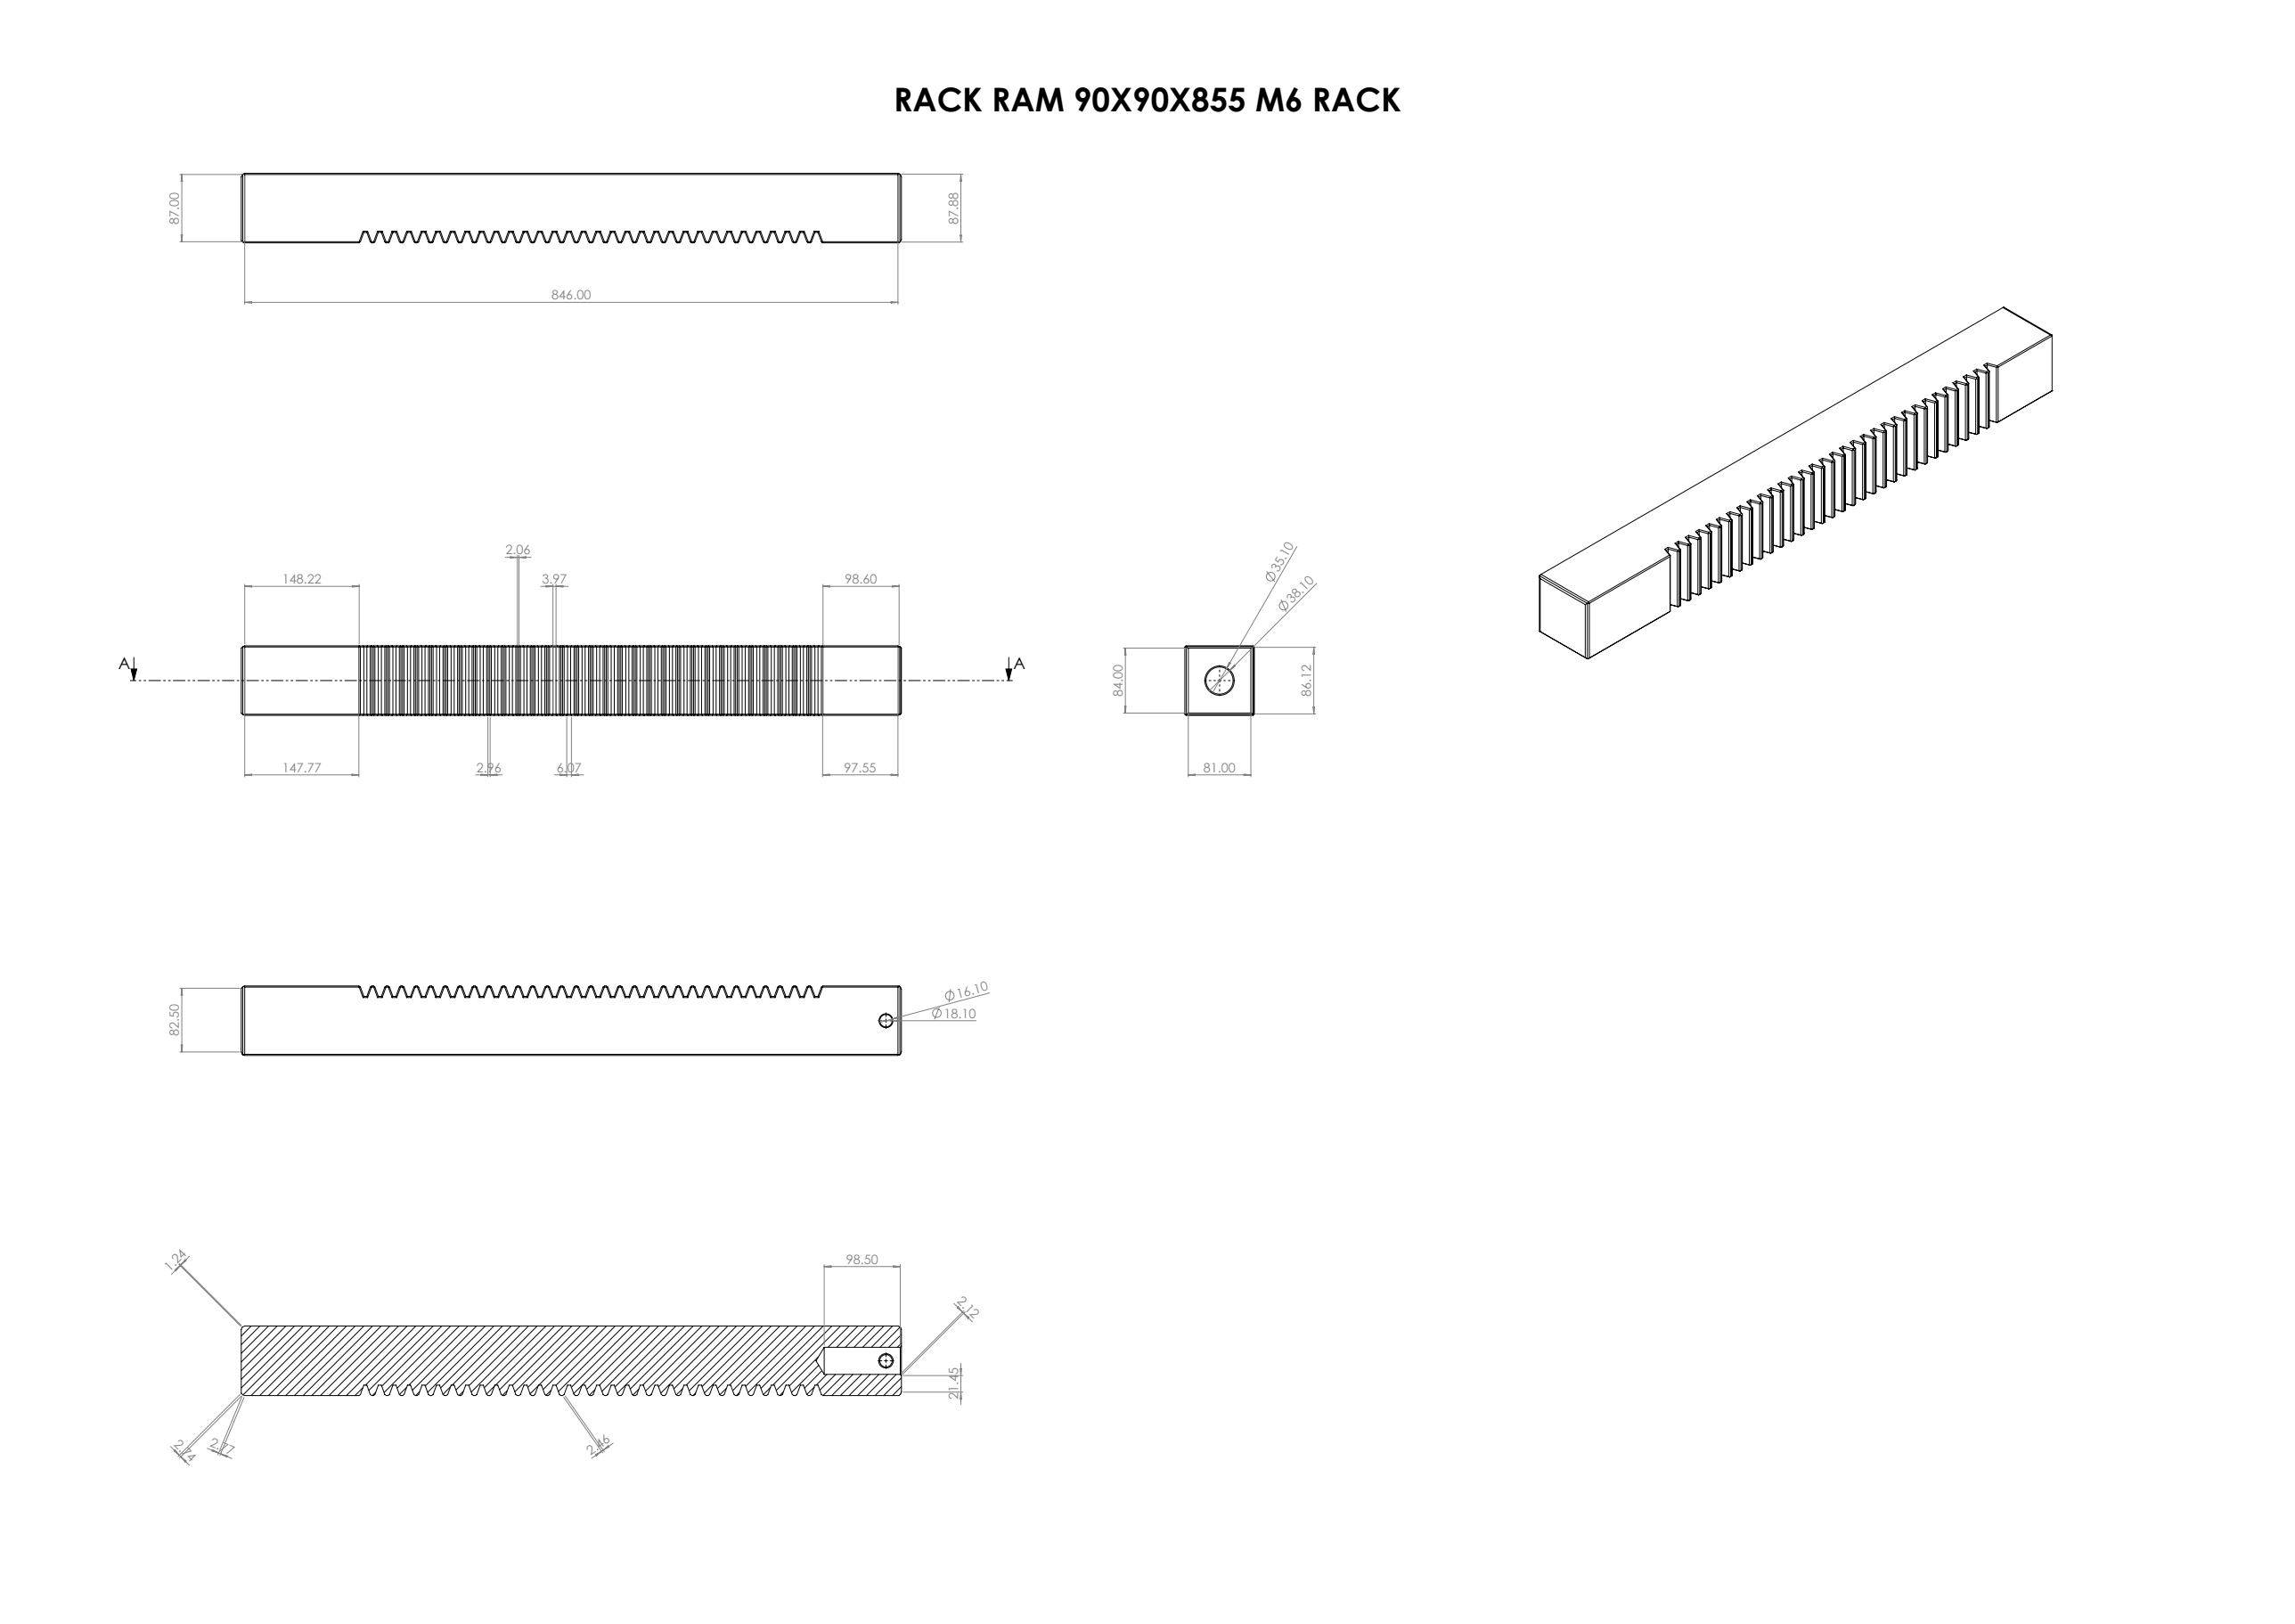
ISO-10303-21;
HEADER;
/* Generated by software containing ST-Developer
 * from STEP Tools, Inc. (www.steptools.com) 
 */

FILE_DESCRIPTION(
/* description */ (''),
/* implementation_level */ '2;1');

FILE_NAME(
/* name */ '02_Rack_Ram_90x90x855_m6_Rack.step',
/* time_stamp */ '2026-10-19T23:58:09-07:00',
/* author */ (''),
/* organization */ (''),
/* preprocessor_version */ 'ST-DEVELOPER v20.2',
/* originating_system */ 'Autodesk Translation Framework v15.15.0.0',
/* authorisation */ '');

FILE_SCHEMA (('AP203_CONFIGURATION_CONTROLLED_3D_DESIGN_OF_MECHANICAL_PARTS_AND_ASSEMBLIES_MIM_LF { 1 0 10303 203 3 1 4 }',
'AUTOMOTIVE_DESIGN { 1 0 10303 214 3 1 1 }','INTEGRATED_CNC_SCHEMA','MODEL_BASED_INTEGRATED_MANUFACTURING_SCHEMA',
'PROCESS_PLANNING_SCHEMA','AP242_MANAGED_MODEL_BASED_3D_ENGINEERING_MIM_LF { 1 0 10303 442 3 1 4 }'));
ENDSEC;

DATA;
#10=MECHANICAL_DESIGN_GEOMETRIC_PRESENTATION_REPRESENTATION('',(#418),#70757);
#286=B_SPLINE_SURFACE_WITH_KNOTS('',3,3,((#63397,#63398,#63399,#63400,#63401,
#63402,#63403,#63404,#63405,#63406,#63407,#63408,#63409,#63410,#63411,#63412,
#63413,#63414,#63415,#63416,#63417,#63418,#63419,#63420,#63421,#63422,#63423,
#63424,#63425,#63426,#63427,#63428,#63429,#63430,#63431,#63432,#63433,#63434,
#63435,#63436),(#63437,#63438,#63439,#63440,#63441,#63442,#63443,#63444,
#63445,#63446,#63447,#63448,#63449,#63450,#63451,#63452,#63453,#63454,#63455,
#63456,#63457,#63458,#63459,#63460,#63461,#63462,#63463,#63464,#63465,#63466,
#63467,#63468,#63469,#63470,#63471,#63472,#63473,#63474,#63475,#63476),
(#63477,#63478,#63479,#63480,#63481,#63482,#63483,#63484,#63485,#63486,
#63487,#63488,#63489,#63490,#63491,#63492,#63493,#63494,#63495,#63496,#63497,
#63498,#63499,#63500,#63501,#63502,#63503,#63504,#63505,#63506,#63507,#63508,
#63509,#63510,#63511,#63512,#63513,#63514,#63515,#63516),(#63517,#63518,
#63519,#63520,#63521,#63522,#63523,#63524,#63525,#63526,#63527,#63528,#63529,
#63530,#63531,#63532,#63533,#63534,#63535,#63536,#63537,#63538,#63539,#63540,
#63541,#63542,#63543,#63544,#63545,#63546,#63547,#63548,#63549,#63550,#63551,
#63552,#63553,#63554,#63555,#63556)),.UNSPECIFIED.,.F.,.T.,.F.,(4,4),(4,
1,1,1,1,1,1,1,1,1,1,1,1,1,1,1,1,1,1,1,1,1,1,1,1,1,1,1,1,1,1,1,1,1,1,1,1,
4),(0.,1.),(0.,0.176188248237271,0.352376496474541,0.528564744711812,0.704752992949082,
0.880941241186353,0.969035365304988,1.01308242736431,1.03510595839396,1.05712948942362,
1.40950598589816,1.42418833991794,1.43887069393771,1.46823540197725,1.52696481805635,
1.64442365021453,1.76188248237271,1.87934131453089,2.11425897884725,2.17298839492634,
2.23171781100543,2.34917664316361,2.58409430747997,2.64282372355906,2.81901197179633,
2.93647080395451,3.05392963611269,3.17138846827087,3.28884730042905,3.52376496474541,
3.64122379690359,3.75868262906177,3.99360029337813,4.22851795769449,4.40470620593176,
4.58089445416904,4.75708270240631,4.93327095064358),.UNSPECIFIED.);
#388=SHAPE_REPRESENTATION_RELATIONSHIP('SRR','None',#70829,#403);
#403=ADVANCED_BREP_SHAPE_REPRESENTATION('',(#478),#70753);
#418=STYLED_ITEM('',(#71033),#478);
#478=MANIFOLD_SOLID_BREP('Ram',#26883);
#728=CYLINDRICAL_SURFACE('',#28278,0.805);
#729=CYLINDRICAL_SURFACE('',#28280,1.755);
#875=FACE_BOUND('',#4734,.T.);
#876=FACE_BOUND('',#4990,.T.);
#877=FACE_BOUND('',#5104,.T.);
#1395=B_SPLINE_CURVE_WITH_KNOTS('',3,(#63561,#63562,#63563,#63564,#63565,
#63566,#63567,#63568,#63569,#63570,#63571,#63572,#63573),.UNSPECIFIED.,
 .F.,.F.,(4,1,1,1,1,1,1,1,1,1,4),(0.,0.176188248237271,0.352376496474541,
0.528564744711812,0.704752992949082,0.880941241186353,0.969035365304988,
1.01308242736431,1.03510595839396,1.05712948942362,1.23331773766089),
 .UNSPECIFIED.);
#1396=B_SPLINE_CURVE_WITH_KNOTS('',3,(#63574,#63575,#63576,#63577,#63578,
#63579,#63580,#63581,#63582,#63583,#63584,#63585,#63586,#63587,#63588,#63589,
#63590,#63591,#63592,#63593,#63594,#63595,#63596,#63597,#63598,#63599,#63600,
#63601,#63602,#63603,#63604),.UNSPECIFIED.,.F.,.F.,(4,1,1,1,1,1,1,1,1,1,
1,1,1,1,1,1,1,1,1,1,1,1,1,1,1,1,1,1,4),(1.23331773766089,1.40950598589816,
1.42418833991794,1.43887069393771,1.46823540197725,1.52696481805635,1.64442365021453,
1.76188248237271,1.87934131453089,2.11425897884725,2.17298839492634,2.23171781100543,
2.34917664316361,2.58409430747997,2.64282372355906,2.81901197179633,2.93647080395451,
3.05392963611269,3.17138846827087,3.28884730042905,3.52376496474541,3.64122379690359,
3.75868262906177,3.99360029337813,4.22851795769449,4.40470620593176,4.58089445416904,
4.75708270240631,4.93327095064358),.UNSPECIFIED.);
#1397=B_SPLINE_CURVE_WITH_KNOTS('',3,(#63605,#63606,#63607,#63608,#63609,
#63610,#63611,#63612,#63613,#63614,#63615,#63616,#63617,#63618,#63619,#63620,
#63621,#63622,#63623,#63624,#63625,#63626,#63627,#63628,#63629,#63630,#63631,
#63632,#63633,#63634,#63635,#63636,#63637,#63638,#63639,#63640,#63641,#63642,
#63643,#63644),.UNSPECIFIED.,.T.,.F.,(4,1,1,1,1,1,1,1,1,1,1,1,1,1,1,1,1,
1,1,1,1,1,1,1,1,1,1,1,1,1,1,1,1,1,1,1,1,4),(-4.93327095064358,-4.75708270240631,
-4.58089445416904,-4.40470620593176,-4.22851795769449,-3.99360029337813,
-3.75868262906177,-3.64122379690359,-3.52376496474541,-3.28884730042905,
-3.17138846827087,-3.05392963611269,-2.93647080395451,-2.81901197179633,
-2.64282372355906,-2.58409430747997,-2.34917664316361,-2.23171781100543,
-2.17298839492634,-2.11425897884725,-1.87934131453089,-1.76188248237271,
-1.64442365021453,-1.52696481805635,-1.46823540197725,-1.43887069393771,
-1.42418833991794,-1.40950598589816,-1.05712948942362,-1.03510595839396,
-1.01308242736431,-0.969035365304988,-0.880941241186353,-0.704752992949082,
-0.528564744711812,-0.352376496474541,-0.176188248237271,0.),
 .UNSPECIFIED.);
#1916=PLANE('',#27819);
#1917=PLANE('',#27820);
#1918=PLANE('',#27821);
#1919=PLANE('',#27822);
#1920=PLANE('',#27823);
#1921=PLANE('',#27824);
#1922=PLANE('',#27825);
#1923=PLANE('',#27826);
#1924=PLANE('',#27827);
#1925=PLANE('',#27828);
#1926=PLANE('',#27829);
#1927=PLANE('',#27830);
#1928=PLANE('',#27831);
#1929=PLANE('',#27832);
#1930=PLANE('',#27833);
#1931=PLANE('',#27834);
#1932=PLANE('',#27835);
#1933=PLANE('',#27836);
#1934=PLANE('',#27837);
#1935=PLANE('',#27838);
#1936=PLANE('',#27839);
#1937=PLANE('',#27840);
#1938=PLANE('',#27841);
#1939=PLANE('',#27842);
#1940=PLANE('',#27843);
#1941=PLANE('',#27844);
#1942=PLANE('',#27845);
#1943=PLANE('',#27846);
#1944=PLANE('',#27847);
#1945=PLANE('',#27848);
#1946=PLANE('',#27849);
#1947=PLANE('',#27850);
#1948=PLANE('',#27851);
#1949=PLANE('',#27852);
#1950=PLANE('',#27853);
#1951=PLANE('',#27854);
#1952=PLANE('',#27855);
#1953=PLANE('',#27856);
#1954=PLANE('',#27857);
#1955=PLANE('',#27858);
#1956=PLANE('',#27859);
#1957=PLANE('',#27860);
#1958=PLANE('',#27861);
#1959=PLANE('',#27862);
#1960=PLANE('',#27863);
#1961=PLANE('',#27864);
#1962=PLANE('',#27865);
#1963=PLANE('',#27866);
#1964=PLANE('',#27867);
#1965=PLANE('',#27868);
#1966=PLANE('',#27869);
#1967=PLANE('',#27870);
#1968=PLANE('',#27871);
#1969=PLANE('',#27872);
#1970=PLANE('',#27873);
#1971=PLANE('',#27874);
#1972=PLANE('',#27875);
#1973=PLANE('',#27876);
#1974=PLANE('',#27877);
#1975=PLANE('',#27878);
#1976=PLANE('',#27879);
#1977=PLANE('',#27880);
#1978=PLANE('',#27881);
#1979=PLANE('',#27882);
#1980=PLANE('',#27883);
#1981=PLANE('',#27884);
#1982=PLANE('',#27885);
#1983=PLANE('',#27886);
#1984=PLANE('',#27887);
#1985=PLANE('',#27888);
#1986=PLANE('',#27889);
#1987=PLANE('',#27890);
#1988=PLANE('',#27891);
#1989=PLANE('',#27892);
#1990=PLANE('',#27893);
#1991=PLANE('',#27894);
#1992=PLANE('',#27895);
#1993=PLANE('',#27896);
#1994=PLANE('',#27897);
#1995=PLANE('',#27898);
#1996=PLANE('',#27899);
#1997=PLANE('',#27900);
#1998=PLANE('',#27901);
#1999=PLANE('',#27902);
#2000=PLANE('',#27903);
#2001=PLANE('',#27904);
#2002=PLANE('',#27905);
#2003=PLANE('',#27906);
#2004=PLANE('',#27907);
#2005=PLANE('',#27908);
#2006=PLANE('',#27909);
#2007=PLANE('',#27910);
#2008=PLANE('',#27912);
#2009=PLANE('',#27913);
#2010=PLANE('',#27914);
#2011=PLANE('',#27915);
#2012=PLANE('',#27916);
#2013=PLANE('',#27917);
#2014=PLANE('',#27918);
#2015=PLANE('',#27919);
#2016=PLANE('',#27920);
#2017=PLANE('',#27921);
#2018=PLANE('',#27922);
#2019=PLANE('',#27923);
#2020=PLANE('',#27924);
#2021=PLANE('',#27925);
#2022=PLANE('',#27926);
#2023=PLANE('',#27927);
#2024=PLANE('',#27928);
#2025=PLANE('',#27929);
#2026=PLANE('',#27930);
#2027=PLANE('',#27931);
#2028=PLANE('',#27932);
#2029=PLANE('',#27933);
#2030=PLANE('',#27934);
#2031=PLANE('',#27935);
#2032=PLANE('',#27936);
#2033=PLANE('',#27937);
#2034=PLANE('',#27938);
#2035=PLANE('',#27939);
#2036=PLANE('',#27940);
#2037=PLANE('',#27941);
#2038=PLANE('',#27942);
#2039=PLANE('',#27943);
#2040=PLANE('',#27944);
#2041=PLANE('',#27945);
#2042=PLANE('',#27946);
#2043=PLANE('',#27947);
#2044=PLANE('',#27948);
#2045=PLANE('',#27949);
#2046=PLANE('',#27950);
#2047=PLANE('',#27951);
#2048=PLANE('',#27952);
#2049=PLANE('',#27953);
#2050=PLANE('',#27954);
#2051=PLANE('',#27955);
#2052=PLANE('',#27956);
#2053=PLANE('',#27957);
#2054=PLANE('',#27958);
#2055=PLANE('',#27959);
#2056=PLANE('',#27960);
#2057=PLANE('',#27961);
#2058=PLANE('',#27962);
#2059=PLANE('',#27963);
#2060=PLANE('',#27964);
#2061=PLANE('',#27965);
#2062=PLANE('',#27966);
#2063=PLANE('',#27967);
#2064=PLANE('',#27968);
#2065=PLANE('',#27969);
#2066=PLANE('',#27970);
#2067=PLANE('',#27971);
#2068=PLANE('',#27972);
#2069=PLANE('',#27973);
#2070=PLANE('',#27974);
#2071=PLANE('',#27975);
#2072=PLANE('',#27976);
#2073=PLANE('',#27977);
#2074=PLANE('',#27978);
#2075=PLANE('',#27979);
#2076=PLANE('',#27980);
#2077=PLANE('',#27981);
#2078=PLANE('',#27982);
#2079=PLANE('',#27983);
#2080=PLANE('',#27984);
#2081=PLANE('',#27985);
#2082=PLANE('',#27986);
#2083=PLANE('',#27987);
#2084=PLANE('',#27988);
#2085=PLANE('',#27989);
#2086=PLANE('',#27990);
#2087=PLANE('',#27991);
#2088=PLANE('',#27992);
#2089=PLANE('',#27993);
#2090=PLANE('',#27994);
#2091=PLANE('',#27995);
#2092=PLANE('',#27996);
#2093=PLANE('',#27997);
#2094=PLANE('',#27998);
#2095=PLANE('',#27999);
#2096=PLANE('',#28000);
#2097=PLANE('',#28001);
#2098=PLANE('',#28002);
#2099=PLANE('',#28003);
#2100=PLANE('',#28004);
#2101=PLANE('',#28005);
#2102=PLANE('',#28006);
#2103=PLANE('',#28007);
#2104=PLANE('',#28008);
#2105=PLANE('',#28009);
#2106=PLANE('',#28010);
#2107=PLANE('',#28011);
#2108=PLANE('',#28012);
#2109=PLANE('',#28013);
#2110=PLANE('',#28014);
#2111=PLANE('',#28015);
#2112=PLANE('',#28016);
#2113=PLANE('',#28017);
#2114=PLANE('',#28018);
#2115=PLANE('',#28019);
#2116=PLANE('',#28020);
#2117=PLANE('',#28021);
#2118=PLANE('',#28022);
#2119=PLANE('',#28023);
#2120=PLANE('',#28024);
#2121=PLANE('',#28025);
#2122=PLANE('',#28026);
#2123=PLANE('',#28027);
#2124=PLANE('',#28028);
#2125=PLANE('',#28029);
#2126=PLANE('',#28030);
#2127=PLANE('',#28031);
#2128=PLANE('',#28032);
#2129=PLANE('',#28033);
#2130=PLANE('',#28034);
#2131=PLANE('',#28035);
#2132=PLANE('',#28036);
#2133=PLANE('',#28037);
#2134=PLANE('',#28038);
#2135=PLANE('',#28039);
#2136=PLANE('',#28040);
#2137=PLANE('',#28041);
#2138=PLANE('',#28042);
#2139=PLANE('',#28043);
#2140=PLANE('',#28044);
#2141=PLANE('',#28045);
#2142=PLANE('',#28046);
#2143=PLANE('',#28047);
#2144=PLANE('',#28048);
#2145=PLANE('',#28049);
#2146=PLANE('',#28050);
#2147=PLANE('',#28051);
#2148=PLANE('',#28052);
#2149=PLANE('',#28053);
#2150=PLANE('',#28054);
#2151=PLANE('',#28055);
#2152=PLANE('',#28056);
#2153=PLANE('',#28057);
#2154=PLANE('',#28058);
#2155=PLANE('',#28059);
#2156=PLANE('',#28060);
#2157=PLANE('',#28061);
#2158=PLANE('',#28062);
#2159=PLANE('',#28063);
#2160=PLANE('',#28064);
#2161=PLANE('',#28065);
#2162=PLANE('',#28066);
#2163=PLANE('',#28067);
#2164=PLANE('',#28068);
#2165=PLANE('',#28069);
#2166=PLANE('',#28070);
#2167=PLANE('',#28071);
#2168=PLANE('',#28072);
#2169=PLANE('',#28073);
#2170=PLANE('',#28074);
#2171=PLANE('',#28075);
#2172=PLANE('',#28076);
#2173=PLANE('',#28077);
#2174=PLANE('',#28078);
#2175=PLANE('',#28079);
#2176=PLANE('',#28080);
#2177=PLANE('',#28081);
#2178=PLANE('',#28082);
#2179=PLANE('',#28083);
#2180=PLANE('',#28084);
#2181=PLANE('',#28085);
#2182=PLANE('',#28086);
#2183=PLANE('',#28087);
#2184=PLANE('',#28088);
#2185=PLANE('',#28089);
#2186=PLANE('',#28090);
#2187=PLANE('',#28091);
#2188=PLANE('',#28092);
#2189=PLANE('',#28093);
#2190=PLANE('',#28094);
#2191=PLANE('',#28095);
#2192=PLANE('',#28096);
#2193=PLANE('',#28097);
#2194=PLANE('',#28098);
#2195=PLANE('',#28099);
#2196=PLANE('',#28100);
#2197=PLANE('',#28101);
#2198=PLANE('',#28102);
#2199=PLANE('',#28103);
#2200=PLANE('',#28104);
#2201=PLANE('',#28105);
#2202=PLANE('',#28106);
#2203=PLANE('',#28107);
#2204=PLANE('',#28108);
#2205=PLANE('',#28109);
#2206=PLANE('',#28110);
#2207=PLANE('',#28111);
#2208=PLANE('',#28112);
#2209=PLANE('',#28113);
#2210=PLANE('',#28114);
#2211=PLANE('',#28115);
#2212=PLANE('',#28116);
#2213=PLANE('',#28117);
#2214=PLANE('',#28118);
#2215=PLANE('',#28119);
#2216=PLANE('',#28120);
#2217=PLANE('',#28121);
#2218=PLANE('',#28122);
#2219=PLANE('',#28123);
#2220=PLANE('',#28124);
#2221=PLANE('',#28125);
#2222=PLANE('',#28126);
#2223=PLANE('',#28127);
#2224=PLANE('',#28128);
#2225=PLANE('',#28129);
#2226=PLANE('',#28130);
#2227=PLANE('',#28131);
#2228=PLANE('',#28132);
#2229=PLANE('',#28133);
#2230=PLANE('',#28134);
#2231=PLANE('',#28135);
#2232=PLANE('',#28136);
#2233=PLANE('',#28137);
#2234=PLANE('',#28138);
#2235=PLANE('',#28139);
#2236=PLANE('',#28140);
#2237=PLANE('',#28141);
#2238=PLANE('',#28142);
#2239=PLANE('',#28143);
#2240=PLANE('',#28144);
#2241=PLANE('',#28145);
#2242=PLANE('',#28146);
#2243=PLANE('',#28147);
#2244=PLANE('',#28148);
#2245=PLANE('',#28149);
#2246=PLANE('',#28150);
#2247=PLANE('',#28151);
#2248=PLANE('',#28152);
#2249=PLANE('',#28153);
#2250=PLANE('',#28154);
#2251=PLANE('',#28155);
#2252=PLANE('',#28156);
#2253=PLANE('',#28157);
#2254=PLANE('',#28158);
#2255=PLANE('',#28159);
#2256=PLANE('',#28160);
#2257=PLANE('',#28161);
#2258=PLANE('',#28162);
#2259=PLANE('',#28163);
#2260=PLANE('',#28164);
#2261=PLANE('',#28165);
#2262=PLANE('',#28166);
#2263=PLANE('',#28168);
#2264=PLANE('',#28169);
#2265=PLANE('',#28170);
#2266=PLANE('',#28171);
#2267=PLANE('',#28172);
#2268=PLANE('',#28173);
#2269=PLANE('',#28174);
#2270=PLANE('',#28175);
#2271=PLANE('',#28176);
#2272=PLANE('',#28177);
#2273=PLANE('',#28178);
#2274=PLANE('',#28179);
#2275=PLANE('',#28180);
#2276=PLANE('',#28181);
#2277=PLANE('',#28182);
#2278=PLANE('',#28183);
#2279=PLANE('',#28184);
#2280=PLANE('',#28185);
#2281=PLANE('',#28186);
#2282=PLANE('',#28187);
#2283=PLANE('',#28188);
#2284=PLANE('',#28189);
#2285=PLANE('',#28190);
#2286=PLANE('',#28191);
#2287=PLANE('',#28192);
#2288=PLANE('',#28193);
#2289=PLANE('',#28194);
#2290=PLANE('',#28195);
#2291=PLANE('',#28196);
#2292=PLANE('',#28197);
#2293=PLANE('',#28198);
#2294=PLANE('',#28199);
#2295=PLANE('',#28200);
#2296=PLANE('',#28201);
#2297=PLANE('',#28202);
#2298=PLANE('',#28203);
#2299=PLANE('',#28204);
#2300=PLANE('',#28205);
#2301=PLANE('',#28206);
#2302=PLANE('',#28207);
#2303=PLANE('',#28208);
#2304=PLANE('',#28209);
#2305=PLANE('',#28210);
#2306=PLANE('',#28211);
#2307=PLANE('',#28212);
#2308=PLANE('',#28213);
#2309=PLANE('',#28214);
#2310=PLANE('',#28215);
#2311=PLANE('',#28216);
#2312=PLANE('',#28217);
#2313=PLANE('',#28218);
#2314=PLANE('',#28219);
#2315=PLANE('',#28220);
#2316=PLANE('',#28221);
#2317=PLANE('',#28222);
#2318=PLANE('',#28223);
#2319=PLANE('',#28224);
#2320=PLANE('',#28225);
#2321=PLANE('',#28226);
#2322=PLANE('',#28227);
#2323=PLANE('',#28228);
#2324=PLANE('',#28229);
#2325=PLANE('',#28230);
#2326=PLANE('',#28231);
#2327=PLANE('',#28232);
#2328=PLANE('',#28233);
#2329=PLANE('',#28234);
#2330=PLANE('',#28235);
#2331=PLANE('',#28236);
#2332=PLANE('',#28237);
#2333=PLANE('',#28238);
#2334=PLANE('',#28239);
#2335=PLANE('',#28240);
#2336=PLANE('',#28241);
#2337=PLANE('',#28242);
#2338=PLANE('',#28243);
#2339=PLANE('',#28244);
#2340=PLANE('',#28245);
#2341=PLANE('',#28246);
#2342=PLANE('',#28247);
#2343=PLANE('',#28248);
#2344=PLANE('',#28249);
#2345=PLANE('',#28250);
#2346=PLANE('',#28251);
#2347=PLANE('',#28252);
#2348=PLANE('',#28253);
#2349=PLANE('',#28254);
#2350=PLANE('',#28255);
#2351=PLANE('',#28256);
#2352=PLANE('',#28257);
#2353=PLANE('',#28258);
#2354=PLANE('',#28259);
#2355=PLANE('',#28260);
#2356=PLANE('',#28261);
#2357=PLANE('',#28262);
#2358=PLANE('',#28263);
#2359=PLANE('',#28264);
#2360=PLANE('',#28265);
#2361=PLANE('',#28266);
#2362=PLANE('',#28267);
#2363=PLANE('',#28268);
#2364=PLANE('',#28269);
#2365=PLANE('',#28270);
#2366=PLANE('',#28271);
#2367=PLANE('',#28272);
#2368=PLANE('',#28273);
#2369=PLANE('',#28274);
#2370=PLANE('',#28275);
#2371=PLANE('',#28276);
#2372=PLANE('',#28277);
#2373=PLANE('',#28286);
#2374=PLANE('',#28287);
#2375=PLANE('',#28288);
#2376=PLANE('',#28289);
#2377=PLANE('',#28290);
#2378=PLANE('',#28291);
#2379=PLANE('',#28292);
#2380=PLANE('',#28293);
#2381=PLANE('',#28294);
#2382=PLANE('',#28295);
#2383=PLANE('',#28296);
#2384=PLANE('',#28297);
#2385=PLANE('',#28298);
#2386=PLANE('',#28299);
#2387=PLANE('',#28300);
#2388=PLANE('',#28301);
#2389=PLANE('',#28302);
#2390=PLANE('',#28303);
#2391=PLANE('',#28304);
#3123=FACE_OUTER_BOUND('',#4642,.T.);
#3124=FACE_OUTER_BOUND('',#4643,.T.);
#3125=FACE_OUTER_BOUND('',#4644,.T.);
#3126=FACE_OUTER_BOUND('',#4645,.T.);
#3127=FACE_OUTER_BOUND('',#4646,.T.);
#3128=FACE_OUTER_BOUND('',#4647,.T.);
#3129=FACE_OUTER_BOUND('',#4648,.T.);
#3130=FACE_OUTER_BOUND('',#4649,.T.);
#3131=FACE_OUTER_BOUND('',#4650,.T.);
#3132=FACE_OUTER_BOUND('',#4651,.T.);
#3133=FACE_OUTER_BOUND('',#4652,.T.);
#3134=FACE_OUTER_BOUND('',#4653,.T.);
#3135=FACE_OUTER_BOUND('',#4654,.T.);
#3136=FACE_OUTER_BOUND('',#4655,.T.);
#3137=FACE_OUTER_BOUND('',#4656,.T.);
#3138=FACE_OUTER_BOUND('',#4657,.T.);
#3139=FACE_OUTER_BOUND('',#4658,.T.);
#3140=FACE_OUTER_BOUND('',#4659,.T.);
#3141=FACE_OUTER_BOUND('',#4660,.T.);
#3142=FACE_OUTER_BOUND('',#4661,.T.);
#3143=FACE_OUTER_BOUND('',#4662,.T.);
#3144=FACE_OUTER_BOUND('',#4663,.T.);
#3145=FACE_OUTER_BOUND('',#4664,.T.);
#3146=FACE_OUTER_BOUND('',#4665,.T.);
#3147=FACE_OUTER_BOUND('',#4666,.T.);
#3148=FACE_OUTER_BOUND('',#4667,.T.);
#3149=FACE_OUTER_BOUND('',#4668,.T.);
#3150=FACE_OUTER_BOUND('',#4669,.T.);
#3151=FACE_OUTER_BOUND('',#4670,.T.);
#3152=FACE_OUTER_BOUND('',#4671,.T.);
#3153=FACE_OUTER_BOUND('',#4672,.T.);
#3154=FACE_OUTER_BOUND('',#4673,.T.);
#3155=FACE_OUTER_BOUND('',#4674,.T.);
#3156=FACE_OUTER_BOUND('',#4675,.T.);
#3157=FACE_OUTER_BOUND('',#4676,.T.);
#3158=FACE_OUTER_BOUND('',#4677,.T.);
#3159=FACE_OUTER_BOUND('',#4678,.T.);
#3160=FACE_OUTER_BOUND('',#4679,.T.);
#3161=FACE_OUTER_BOUND('',#4680,.T.);
#3162=FACE_OUTER_BOUND('',#4681,.T.);
#3163=FACE_OUTER_BOUND('',#4682,.T.);
#3164=FACE_OUTER_BOUND('',#4683,.T.);
#3165=FACE_OUTER_BOUND('',#4684,.T.);
#3166=FACE_OUTER_BOUND('',#4685,.T.);
#3167=FACE_OUTER_BOUND('',#4686,.T.);
#3168=FACE_OUTER_BOUND('',#4687,.T.);
#3169=FACE_OUTER_BOUND('',#4688,.T.);
#3170=FACE_OUTER_BOUND('',#4689,.T.);
#3171=FACE_OUTER_BOUND('',#4690,.T.);
#3172=FACE_OUTER_BOUND('',#4691,.T.);
#3173=FACE_OUTER_BOUND('',#4692,.T.);
#3174=FACE_OUTER_BOUND('',#4693,.T.);
#3175=FACE_OUTER_BOUND('',#4694,.T.);
#3176=FACE_OUTER_BOUND('',#4695,.T.);
#3177=FACE_OUTER_BOUND('',#4696,.T.);
#3178=FACE_OUTER_BOUND('',#4697,.T.);
#3179=FACE_OUTER_BOUND('',#4698,.T.);
#3180=FACE_OUTER_BOUND('',#4699,.T.);
#3181=FACE_OUTER_BOUND('',#4700,.T.);
#3182=FACE_OUTER_BOUND('',#4701,.T.);
#3183=FACE_OUTER_BOUND('',#4702,.T.);
#3184=FACE_OUTER_BOUND('',#4703,.T.);
#3185=FACE_OUTER_BOUND('',#4704,.T.);
#3186=FACE_OUTER_BOUND('',#4705,.T.);
#3187=FACE_OUTER_BOUND('',#4706,.T.);
#3188=FACE_OUTER_BOUND('',#4707,.T.);
#3189=FACE_OUTER_BOUND('',#4708,.T.);
#3190=FACE_OUTER_BOUND('',#4709,.T.);
#3191=FACE_OUTER_BOUND('',#4710,.T.);
#3192=FACE_OUTER_BOUND('',#4711,.T.);
#3193=FACE_OUTER_BOUND('',#4712,.T.);
#3194=FACE_OUTER_BOUND('',#4713,.T.);
#3195=FACE_OUTER_BOUND('',#4714,.T.);
#3196=FACE_OUTER_BOUND('',#4715,.T.);
#3197=FACE_OUTER_BOUND('',#4716,.T.);
#3198=FACE_OUTER_BOUND('',#4717,.T.);
#3199=FACE_OUTER_BOUND('',#4718,.T.);
#3200=FACE_OUTER_BOUND('',#4719,.T.);
#3201=FACE_OUTER_BOUND('',#4720,.T.);
#3202=FACE_OUTER_BOUND('',#4721,.T.);
#3203=FACE_OUTER_BOUND('',#4722,.T.);
#3204=FACE_OUTER_BOUND('',#4723,.T.);
#3205=FACE_OUTER_BOUND('',#4724,.T.);
#3206=FACE_OUTER_BOUND('',#4725,.T.);
#3207=FACE_OUTER_BOUND('',#4726,.T.);
#3208=FACE_OUTER_BOUND('',#4727,.T.);
#3209=FACE_OUTER_BOUND('',#4728,.T.);
#3210=FACE_OUTER_BOUND('',#4729,.T.);
#3211=FACE_OUTER_BOUND('',#4730,.T.);
#3212=FACE_OUTER_BOUND('',#4731,.T.);
#3213=FACE_OUTER_BOUND('',#4732,.T.);
#3214=FACE_OUTER_BOUND('',#4733,.T.);
#3215=FACE_OUTER_BOUND('',#4735,.T.);
#3216=FACE_OUTER_BOUND('',#4736,.T.);
#3217=FACE_OUTER_BOUND('',#4737,.T.);
#3218=FACE_OUTER_BOUND('',#4738,.T.);
#3219=FACE_OUTER_BOUND('',#4739,.T.);
#3220=FACE_OUTER_BOUND('',#4740,.T.);
#3221=FACE_OUTER_BOUND('',#4741,.T.);
#3222=FACE_OUTER_BOUND('',#4742,.T.);
#3223=FACE_OUTER_BOUND('',#4743,.T.);
#3224=FACE_OUTER_BOUND('',#4744,.T.);
#3225=FACE_OUTER_BOUND('',#4745,.T.);
#3226=FACE_OUTER_BOUND('',#4746,.T.);
#3227=FACE_OUTER_BOUND('',#4747,.T.);
#3228=FACE_OUTER_BOUND('',#4748,.T.);
#3229=FACE_OUTER_BOUND('',#4749,.T.);
#3230=FACE_OUTER_BOUND('',#4750,.T.);
#3231=FACE_OUTER_BOUND('',#4751,.T.);
#3232=FACE_OUTER_BOUND('',#4752,.T.);
#3233=FACE_OUTER_BOUND('',#4753,.T.);
#3234=FACE_OUTER_BOUND('',#4754,.T.);
#3235=FACE_OUTER_BOUND('',#4755,.T.);
#3236=FACE_OUTER_BOUND('',#4756,.T.);
#3237=FACE_OUTER_BOUND('',#4757,.T.);
#3238=FACE_OUTER_BOUND('',#4758,.T.);
#3239=FACE_OUTER_BOUND('',#4759,.T.);
#3240=FACE_OUTER_BOUND('',#4760,.T.);
#3241=FACE_OUTER_BOUND('',#4761,.T.);
#3242=FACE_OUTER_BOUND('',#4762,.T.);
#3243=FACE_OUTER_BOUND('',#4763,.T.);
#3244=FACE_OUTER_BOUND('',#4764,.T.);
#3245=FACE_OUTER_BOUND('',#4765,.T.);
#3246=FACE_OUTER_BOUND('',#4766,.T.);
#3247=FACE_OUTER_BOUND('',#4767,.T.);
#3248=FACE_OUTER_BOUND('',#4768,.T.);
#3249=FACE_OUTER_BOUND('',#4769,.T.);
#3250=FACE_OUTER_BOUND('',#4770,.T.);
#3251=FACE_OUTER_BOUND('',#4771,.T.);
#3252=FACE_OUTER_BOUND('',#4772,.T.);
#3253=FACE_OUTER_BOUND('',#4773,.T.);
#3254=FACE_OUTER_BOUND('',#4774,.T.);
#3255=FACE_OUTER_BOUND('',#4775,.T.);
#3256=FACE_OUTER_BOUND('',#4776,.T.);
#3257=FACE_OUTER_BOUND('',#4777,.T.);
#3258=FACE_OUTER_BOUND('',#4778,.T.);
#3259=FACE_OUTER_BOUND('',#4779,.T.);
#3260=FACE_OUTER_BOUND('',#4780,.T.);
#3261=FACE_OUTER_BOUND('',#4781,.T.);
#3262=FACE_OUTER_BOUND('',#4782,.T.);
#3263=FACE_OUTER_BOUND('',#4783,.T.);
#3264=FACE_OUTER_BOUND('',#4784,.T.);
#3265=FACE_OUTER_BOUND('',#4785,.T.);
#3266=FACE_OUTER_BOUND('',#4786,.T.);
#3267=FACE_OUTER_BOUND('',#4787,.T.);
#3268=FACE_OUTER_BOUND('',#4788,.T.);
#3269=FACE_OUTER_BOUND('',#4789,.T.);
#3270=FACE_OUTER_BOUND('',#4790,.T.);
#3271=FACE_OUTER_BOUND('',#4791,.T.);
#3272=FACE_OUTER_BOUND('',#4792,.T.);
#3273=FACE_OUTER_BOUND('',#4793,.T.);
#3274=FACE_OUTER_BOUND('',#4794,.T.);
#3275=FACE_OUTER_BOUND('',#4795,.T.);
#3276=FACE_OUTER_BOUND('',#4796,.T.);
#3277=FACE_OUTER_BOUND('',#4797,.T.);
#3278=FACE_OUTER_BOUND('',#4798,.T.);
#3279=FACE_OUTER_BOUND('',#4799,.T.);
#3280=FACE_OUTER_BOUND('',#4800,.T.);
#3281=FACE_OUTER_BOUND('',#4801,.T.);
#3282=FACE_OUTER_BOUND('',#4802,.T.);
#3283=FACE_OUTER_BOUND('',#4803,.T.);
#3284=FACE_OUTER_BOUND('',#4804,.T.);
#3285=FACE_OUTER_BOUND('',#4805,.T.);
#3286=FACE_OUTER_BOUND('',#4806,.T.);
#3287=FACE_OUTER_BOUND('',#4807,.T.);
#3288=FACE_OUTER_BOUND('',#4808,.T.);
#3289=FACE_OUTER_BOUND('',#4809,.T.);
#3290=FACE_OUTER_BOUND('',#4810,.T.);
#3291=FACE_OUTER_BOUND('',#4811,.T.);
#3292=FACE_OUTER_BOUND('',#4812,.T.);
#3293=FACE_OUTER_BOUND('',#4813,.T.);
#3294=FACE_OUTER_BOUND('',#4814,.T.);
#3295=FACE_OUTER_BOUND('',#4815,.T.);
#3296=FACE_OUTER_BOUND('',#4816,.T.);
#3297=FACE_OUTER_BOUND('',#4817,.T.);
#3298=FACE_OUTER_BOUND('',#4818,.T.);
#3299=FACE_OUTER_BOUND('',#4819,.T.);
#3300=FACE_OUTER_BOUND('',#4820,.T.);
#3301=FACE_OUTER_BOUND('',#4821,.T.);
#3302=FACE_OUTER_BOUND('',#4822,.T.);
#3303=FACE_OUTER_BOUND('',#4823,.T.);
#3304=FACE_OUTER_BOUND('',#4824,.T.);
#3305=FACE_OUTER_BOUND('',#4825,.T.);
#3306=FACE_OUTER_BOUND('',#4826,.T.);
#3307=FACE_OUTER_BOUND('',#4827,.T.);
#3308=FACE_OUTER_BOUND('',#4828,.T.);
#3309=FACE_OUTER_BOUND('',#4829,.T.);
#3310=FACE_OUTER_BOUND('',#4830,.T.);
#3311=FACE_OUTER_BOUND('',#4831,.T.);
#3312=FACE_OUTER_BOUND('',#4832,.T.);
#3313=FACE_OUTER_BOUND('',#4833,.T.);
#3314=FACE_OUTER_BOUND('',#4834,.T.);
#3315=FACE_OUTER_BOUND('',#4835,.T.);
#3316=FACE_OUTER_BOUND('',#4836,.T.);
#3317=FACE_OUTER_BOUND('',#4837,.T.);
#3318=FACE_OUTER_BOUND('',#4838,.T.);
#3319=FACE_OUTER_BOUND('',#4839,.T.);
#3320=FACE_OUTER_BOUND('',#4840,.T.);
#3321=FACE_OUTER_BOUND('',#4841,.T.);
#3322=FACE_OUTER_BOUND('',#4842,.T.);
#3323=FACE_OUTER_BOUND('',#4843,.T.);
#3324=FACE_OUTER_BOUND('',#4844,.T.);
#3325=FACE_OUTER_BOUND('',#4845,.T.);
#3326=FACE_OUTER_BOUND('',#4846,.T.);
#3327=FACE_OUTER_BOUND('',#4847,.T.);
#3328=FACE_OUTER_BOUND('',#4848,.T.);
#3329=FACE_OUTER_BOUND('',#4849,.T.);
#3330=FACE_OUTER_BOUND('',#4850,.T.);
#3331=FACE_OUTER_BOUND('',#4851,.T.);
#3332=FACE_OUTER_BOUND('',#4852,.T.);
#3333=FACE_OUTER_BOUND('',#4853,.T.);
#3334=FACE_OUTER_BOUND('',#4854,.T.);
#3335=FACE_OUTER_BOUND('',#4855,.T.);
#3336=FACE_OUTER_BOUND('',#4856,.T.);
#3337=FACE_OUTER_BOUND('',#4857,.T.);
#3338=FACE_OUTER_BOUND('',#4858,.T.);
#3339=FACE_OUTER_BOUND('',#4859,.T.);
#3340=FACE_OUTER_BOUND('',#4860,.T.);
#3341=FACE_OUTER_BOUND('',#4861,.T.);
#3342=FACE_OUTER_BOUND('',#4862,.T.);
#3343=FACE_OUTER_BOUND('',#4863,.T.);
#3344=FACE_OUTER_BOUND('',#4864,.T.);
#3345=FACE_OUTER_BOUND('',#4865,.T.);
#3346=FACE_OUTER_BOUND('',#4866,.T.);
#3347=FACE_OUTER_BOUND('',#4867,.T.);
#3348=FACE_OUTER_BOUND('',#4868,.T.);
#3349=FACE_OUTER_BOUND('',#4869,.T.);
#3350=FACE_OUTER_BOUND('',#4870,.T.);
#3351=FACE_OUTER_BOUND('',#4871,.T.);
#3352=FACE_OUTER_BOUND('',#4872,.T.);
#3353=FACE_OUTER_BOUND('',#4873,.T.);
#3354=FACE_OUTER_BOUND('',#4874,.T.);
#3355=FACE_OUTER_BOUND('',#4875,.T.);
#3356=FACE_OUTER_BOUND('',#4876,.T.);
#3357=FACE_OUTER_BOUND('',#4877,.T.);
#3358=FACE_OUTER_BOUND('',#4878,.T.);
#3359=FACE_OUTER_BOUND('',#4879,.T.);
#3360=FACE_OUTER_BOUND('',#4880,.T.);
#3361=FACE_OUTER_BOUND('',#4881,.T.);
#3362=FACE_OUTER_BOUND('',#4882,.T.);
#3363=FACE_OUTER_BOUND('',#4883,.T.);
#3364=FACE_OUTER_BOUND('',#4884,.T.);
#3365=FACE_OUTER_BOUND('',#4885,.T.);
#3366=FACE_OUTER_BOUND('',#4886,.T.);
#3367=FACE_OUTER_BOUND('',#4887,.T.);
#3368=FACE_OUTER_BOUND('',#4888,.T.);
#3369=FACE_OUTER_BOUND('',#4889,.T.);
#3370=FACE_OUTER_BOUND('',#4890,.T.);
#3371=FACE_OUTER_BOUND('',#4891,.T.);
#3372=FACE_OUTER_BOUND('',#4892,.T.);
#3373=FACE_OUTER_BOUND('',#4893,.T.);
#3374=FACE_OUTER_BOUND('',#4894,.T.);
#3375=FACE_OUTER_BOUND('',#4895,.T.);
#3376=FACE_OUTER_BOUND('',#4896,.T.);
#3377=FACE_OUTER_BOUND('',#4897,.T.);
#3378=FACE_OUTER_BOUND('',#4898,.T.);
#3379=FACE_OUTER_BOUND('',#4899,.T.);
#3380=FACE_OUTER_BOUND('',#4900,.T.);
#3381=FACE_OUTER_BOUND('',#4901,.T.);
#3382=FACE_OUTER_BOUND('',#4902,.T.);
#3383=FACE_OUTER_BOUND('',#4903,.T.);
#3384=FACE_OUTER_BOUND('',#4904,.T.);
#3385=FACE_OUTER_BOUND('',#4905,.T.);
#3386=FACE_OUTER_BOUND('',#4906,.T.);
#3387=FACE_OUTER_BOUND('',#4907,.T.);
#3388=FACE_OUTER_BOUND('',#4908,.T.);
#3389=FACE_OUTER_BOUND('',#4909,.T.);
#3390=FACE_OUTER_BOUND('',#4910,.T.);
#3391=FACE_OUTER_BOUND('',#4911,.T.);
#3392=FACE_OUTER_BOUND('',#4912,.T.);
#3393=FACE_OUTER_BOUND('',#4913,.T.);
#3394=FACE_OUTER_BOUND('',#4914,.T.);
#3395=FACE_OUTER_BOUND('',#4915,.T.);
#3396=FACE_OUTER_BOUND('',#4916,.T.);
#3397=FACE_OUTER_BOUND('',#4917,.T.);
#3398=FACE_OUTER_BOUND('',#4918,.T.);
#3399=FACE_OUTER_BOUND('',#4919,.T.);
#3400=FACE_OUTER_BOUND('',#4920,.T.);
#3401=FACE_OUTER_BOUND('',#4921,.T.);
#3402=FACE_OUTER_BOUND('',#4922,.T.);
#3403=FACE_OUTER_BOUND('',#4923,.T.);
#3404=FACE_OUTER_BOUND('',#4924,.T.);
#3405=FACE_OUTER_BOUND('',#4925,.T.);
#3406=FACE_OUTER_BOUND('',#4926,.T.);
#3407=FACE_OUTER_BOUND('',#4927,.T.);
#3408=FACE_OUTER_BOUND('',#4928,.T.);
#3409=FACE_OUTER_BOUND('',#4929,.T.);
#3410=FACE_OUTER_BOUND('',#4930,.T.);
#3411=FACE_OUTER_BOUND('',#4931,.T.);
#3412=FACE_OUTER_BOUND('',#4932,.T.);
#3413=FACE_OUTER_BOUND('',#4933,.T.);
#3414=FACE_OUTER_BOUND('',#4934,.T.);
#3415=FACE_OUTER_BOUND('',#4935,.T.);
#3416=FACE_OUTER_BOUND('',#4936,.T.);
#3417=FACE_OUTER_BOUND('',#4937,.T.);
#3418=FACE_OUTER_BOUND('',#4938,.T.);
#3419=FACE_OUTER_BOUND('',#4939,.T.);
#3420=FACE_OUTER_BOUND('',#4940,.T.);
#3421=FACE_OUTER_BOUND('',#4941,.T.);
#3422=FACE_OUTER_BOUND('',#4942,.T.);
#3423=FACE_OUTER_BOUND('',#4943,.T.);
#3424=FACE_OUTER_BOUND('',#4944,.T.);
#3425=FACE_OUTER_BOUND('',#4945,.T.);
#3426=FACE_OUTER_BOUND('',#4946,.T.);
#3427=FACE_OUTER_BOUND('',#4947,.T.);
#3428=FACE_OUTER_BOUND('',#4948,.T.);
#3429=FACE_OUTER_BOUND('',#4949,.T.);
#3430=FACE_OUTER_BOUND('',#4950,.T.);
#3431=FACE_OUTER_BOUND('',#4951,.T.);
#3432=FACE_OUTER_BOUND('',#4952,.T.);
#3433=FACE_OUTER_BOUND('',#4953,.T.);
#3434=FACE_OUTER_BOUND('',#4954,.T.);
#3435=FACE_OUTER_BOUND('',#4955,.T.);
#3436=FACE_OUTER_BOUND('',#4956,.T.);
#3437=FACE_OUTER_BOUND('',#4957,.T.);
#3438=FACE_OUTER_BOUND('',#4958,.T.);
#3439=FACE_OUTER_BOUND('',#4959,.T.);
#3440=FACE_OUTER_BOUND('',#4960,.T.);
#3441=FACE_OUTER_BOUND('',#4961,.T.);
#3442=FACE_OUTER_BOUND('',#4962,.T.);
#3443=FACE_OUTER_BOUND('',#4963,.T.);
#3444=FACE_OUTER_BOUND('',#4964,.T.);
#3445=FACE_OUTER_BOUND('',#4965,.T.);
#3446=FACE_OUTER_BOUND('',#4966,.T.);
#3447=FACE_OUTER_BOUND('',#4967,.T.);
#3448=FACE_OUTER_BOUND('',#4968,.T.);
#3449=FACE_OUTER_BOUND('',#4969,.T.);
#3450=FACE_OUTER_BOUND('',#4970,.T.);
#3451=FACE_OUTER_BOUND('',#4971,.T.);
#3452=FACE_OUTER_BOUND('',#4972,.T.);
#3453=FACE_OUTER_BOUND('',#4973,.T.);
#3454=FACE_OUTER_BOUND('',#4974,.T.);
#3455=FACE_OUTER_BOUND('',#4975,.T.);
#3456=FACE_OUTER_BOUND('',#4976,.T.);
#3457=FACE_OUTER_BOUND('',#4977,.T.);
#3458=FACE_OUTER_BOUND('',#4978,.T.);
#3459=FACE_OUTER_BOUND('',#4979,.T.);
#3460=FACE_OUTER_BOUND('',#4980,.T.);
#3461=FACE_OUTER_BOUND('',#4981,.T.);
#3462=FACE_OUTER_BOUND('',#4982,.T.);
#3463=FACE_OUTER_BOUND('',#4983,.T.);
#3464=FACE_OUTER_BOUND('',#4984,.T.);
#3465=FACE_OUTER_BOUND('',#4985,.T.);
#3466=FACE_OUTER_BOUND('',#4986,.T.);
#3467=FACE_OUTER_BOUND('',#4987,.T.);
#3468=FACE_OUTER_BOUND('',#4988,.T.);
#3469=FACE_OUTER_BOUND('',#4989,.T.);
#3470=FACE_OUTER_BOUND('',#4991,.T.);
#3471=FACE_OUTER_BOUND('',#4992,.T.);
#3472=FACE_OUTER_BOUND('',#4993,.T.);
#3473=FACE_OUTER_BOUND('',#4994,.T.);
#3474=FACE_OUTER_BOUND('',#4995,.T.);
#3475=FACE_OUTER_BOUND('',#4996,.T.);
#3476=FACE_OUTER_BOUND('',#4997,.T.);
#3477=FACE_OUTER_BOUND('',#4998,.T.);
#3478=FACE_OUTER_BOUND('',#4999,.T.);
#3479=FACE_OUTER_BOUND('',#5000,.T.);
#3480=FACE_OUTER_BOUND('',#5001,.T.);
#3481=FACE_OUTER_BOUND('',#5002,.T.);
#3482=FACE_OUTER_BOUND('',#5003,.T.);
#3483=FACE_OUTER_BOUND('',#5004,.T.);
#3484=FACE_OUTER_BOUND('',#5005,.T.);
#3485=FACE_OUTER_BOUND('',#5006,.T.);
#3486=FACE_OUTER_BOUND('',#5007,.T.);
#3487=FACE_OUTER_BOUND('',#5008,.T.);
#3488=FACE_OUTER_BOUND('',#5009,.T.);
#3489=FACE_OUTER_BOUND('',#5010,.T.);
#3490=FACE_OUTER_BOUND('',#5011,.T.);
#3491=FACE_OUTER_BOUND('',#5012,.T.);
#3492=FACE_OUTER_BOUND('',#5013,.T.);
#3493=FACE_OUTER_BOUND('',#5014,.T.);
#3494=FACE_OUTER_BOUND('',#5015,.T.);
#3495=FACE_OUTER_BOUND('',#5016,.T.);
#3496=FACE_OUTER_BOUND('',#5017,.T.);
#3497=FACE_OUTER_BOUND('',#5018,.T.);
#3498=FACE_OUTER_BOUND('',#5019,.T.);
#3499=FACE_OUTER_BOUND('',#5020,.T.);
#3500=FACE_OUTER_BOUND('',#5021,.T.);
#3501=FACE_OUTER_BOUND('',#5022,.T.);
#3502=FACE_OUTER_BOUND('',#5023,.T.);
#3503=FACE_OUTER_BOUND('',#5024,.T.);
#3504=FACE_OUTER_BOUND('',#5025,.T.);
#3505=FACE_OUTER_BOUND('',#5026,.T.);
#3506=FACE_OUTER_BOUND('',#5027,.T.);
#3507=FACE_OUTER_BOUND('',#5028,.T.);
#3508=FACE_OUTER_BOUND('',#5029,.T.);
#3509=FACE_OUTER_BOUND('',#5030,.T.);
#3510=FACE_OUTER_BOUND('',#5031,.T.);
#3511=FACE_OUTER_BOUND('',#5032,.T.);
#3512=FACE_OUTER_BOUND('',#5033,.T.);
#3513=FACE_OUTER_BOUND('',#5034,.T.);
#3514=FACE_OUTER_BOUND('',#5035,.T.);
#3515=FACE_OUTER_BOUND('',#5036,.T.);
#3516=FACE_OUTER_BOUND('',#5037,.T.);
#3517=FACE_OUTER_BOUND('',#5038,.T.);
#3518=FACE_OUTER_BOUND('',#5039,.T.);
#3519=FACE_OUTER_BOUND('',#5040,.T.);
#3520=FACE_OUTER_BOUND('',#5041,.T.);
#3521=FACE_OUTER_BOUND('',#5042,.T.);
#3522=FACE_OUTER_BOUND('',#5043,.T.);
#3523=FACE_OUTER_BOUND('',#5044,.T.);
#3524=FACE_OUTER_BOUND('',#5045,.T.);
#3525=FACE_OUTER_BOUND('',#5046,.T.);
#3526=FACE_OUTER_BOUND('',#5047,.T.);
#3527=FACE_OUTER_BOUND('',#5048,.T.);
#3528=FACE_OUTER_BOUND('',#5049,.T.);
#3529=FACE_OUTER_BOUND('',#5050,.T.);
#3530=FACE_OUTER_BOUND('',#5051,.T.);
#3531=FACE_OUTER_BOUND('',#5052,.T.);
#3532=FACE_OUTER_BOUND('',#5053,.T.);
#3533=FACE_OUTER_BOUND('',#5054,.T.);
#3534=FACE_OUTER_BOUND('',#5055,.T.);
#3535=FACE_OUTER_BOUND('',#5056,.T.);
#3536=FACE_OUTER_BOUND('',#5057,.T.);
#3537=FACE_OUTER_BOUND('',#5058,.T.);
#3538=FACE_OUTER_BOUND('',#5059,.T.);
#3539=FACE_OUTER_BOUND('',#5060,.T.);
#3540=FACE_OUTER_BOUND('',#5061,.T.);
#3541=FACE_OUTER_BOUND('',#5062,.T.);
#3542=FACE_OUTER_BOUND('',#5063,.T.);
#3543=FACE_OUTER_BOUND('',#5064,.T.);
#3544=FACE_OUTER_BOUND('',#5065,.T.);
#3545=FACE_OUTER_BOUND('',#5066,.T.);
#3546=FACE_OUTER_BOUND('',#5067,.T.);
#3547=FACE_OUTER_BOUND('',#5068,.T.);
#3548=FACE_OUTER_BOUND('',#5069,.T.);
#3549=FACE_OUTER_BOUND('',#5070,.T.);
#3550=FACE_OUTER_BOUND('',#5071,.T.);
#3551=FACE_OUTER_BOUND('',#5072,.T.);
#3552=FACE_OUTER_BOUND('',#5073,.T.);
#3553=FACE_OUTER_BOUND('',#5074,.T.);
#3554=FACE_OUTER_BOUND('',#5075,.T.);
#3555=FACE_OUTER_BOUND('',#5076,.T.);
#3556=FACE_OUTER_BOUND('',#5077,.T.);
#3557=FACE_OUTER_BOUND('',#5078,.T.);
#3558=FACE_OUTER_BOUND('',#5079,.T.);
#3559=FACE_OUTER_BOUND('',#5080,.T.);
#3560=FACE_OUTER_BOUND('',#5081,.T.);
#3561=FACE_OUTER_BOUND('',#5082,.T.);
#3562=FACE_OUTER_BOUND('',#5083,.T.);
#3563=FACE_OUTER_BOUND('',#5084,.T.);
#3564=FACE_OUTER_BOUND('',#5085,.T.);
#3565=FACE_OUTER_BOUND('',#5086,.T.);
#3566=FACE_OUTER_BOUND('',#5087,.T.);
#3567=FACE_OUTER_BOUND('',#5088,.T.);
#3568=FACE_OUTER_BOUND('',#5089,.T.);
#3569=FACE_OUTER_BOUND('',#5090,.T.);
#3570=FACE_OUTER_BOUND('',#5091,.T.);
#3571=FACE_OUTER_BOUND('',#5092,.T.);
#3572=FACE_OUTER_BOUND('',#5093,.T.);
#3573=FACE_OUTER_BOUND('',#5094,.T.);
#3574=FACE_OUTER_BOUND('',#5095,.T.);
#3575=FACE_OUTER_BOUND('',#5096,.T.);
#3576=FACE_OUTER_BOUND('',#5097,.T.);
#3577=FACE_OUTER_BOUND('',#5098,.T.);
#3578=FACE_OUTER_BOUND('',#5099,.T.);
#3579=FACE_OUTER_BOUND('',#5100,.T.);
#3580=FACE_OUTER_BOUND('',#5101,.T.);
#3581=FACE_OUTER_BOUND('',#5102,.T.);
#3582=FACE_OUTER_BOUND('',#5103,.T.);
#3583=FACE_OUTER_BOUND('',#5105,.T.);
#3584=FACE_OUTER_BOUND('',#5106,.T.);
#3585=FACE_OUTER_BOUND('',#5107,.T.);
#3586=FACE_OUTER_BOUND('',#5108,.T.);
#3587=FACE_OUTER_BOUND('',#5109,.T.);
#3588=FACE_OUTER_BOUND('',#5110,.T.);
#3589=FACE_OUTER_BOUND('',#5111,.T.);
#3590=FACE_OUTER_BOUND('',#5112,.T.);
#3591=FACE_OUTER_BOUND('',#5113,.T.);
#3592=FACE_OUTER_BOUND('',#5114,.T.);
#3593=FACE_OUTER_BOUND('',#5115,.T.);
#3594=FACE_OUTER_BOUND('',#5116,.T.);
#3595=FACE_OUTER_BOUND('',#5117,.T.);
#3596=FACE_OUTER_BOUND('',#5118,.T.);
#3597=FACE_OUTER_BOUND('',#5119,.T.);
#3598=FACE_OUTER_BOUND('',#5120,.T.);
#3599=FACE_OUTER_BOUND('',#5121,.T.);
#3600=FACE_OUTER_BOUND('',#5122,.T.);
#3601=FACE_OUTER_BOUND('',#5123,.T.);
#3602=FACE_OUTER_BOUND('',#5124,.T.);
#3603=FACE_OUTER_BOUND('',#5125,.T.);
#3604=FACE_OUTER_BOUND('',#5126,.T.);
#4642=EDGE_LOOP('',(#20340,#20341,#20342,#20343,#20344,#20345));
#4643=EDGE_LOOP('',(#20346,#20347,#20348,#20349,#20350));
#4644=EDGE_LOOP('',(#20351,#20352,#20353,#20354));
#4645=EDGE_LOOP('',(#20355,#20356,#20357,#20358,#20359));
#4646=EDGE_LOOP('',(#20360,#20361,#20362,#20363,#20364,#20365));
#4647=EDGE_LOOP('',(#20366,#20367,#20368,#20369,#20370));
#4648=EDGE_LOOP('',(#20371,#20372,#20373,#20374));
#4649=EDGE_LOOP('',(#20375,#20376,#20377,#20378,#20379));
#4650=EDGE_LOOP('',(#20380,#20381,#20382,#20383,#20384,#20385));
#4651=EDGE_LOOP('',(#20386,#20387,#20388,#20389));
#4652=EDGE_LOOP('',(#20390,#20391,#20392,#20393,#20394));
#4653=EDGE_LOOP('',(#20395,#20396,#20397,#20398,#20399,#20400));
#4654=EDGE_LOOP('',(#20401,#20402,#20403,#20404,#20405,#20406));
#4655=EDGE_LOOP('',(#20407,#20408,#20409,#20410,#20411));
#4656=EDGE_LOOP('',(#20412,#20413,#20414,#20415));
#4657=EDGE_LOOP('',(#20416,#20417,#20418,#20419,#20420));
#4658=EDGE_LOOP('',(#20421,#20422,#20423,#20424,#20425,#20426));
#4659=EDGE_LOOP('',(#20427,#20428,#20429,#20430));
#4660=EDGE_LOOP('',(#20431,#20432,#20433,#20434,#20435,#20436));
#4661=EDGE_LOOP('',(#20437,#20438,#20439,#20440,#20441));
#4662=EDGE_LOOP('',(#20442,#20443,#20444,#20445,#20446,#20447));
#4663=EDGE_LOOP('',(#20448,#20449,#20450,#20451,#20452));
#4664=EDGE_LOOP('',(#20453,#20454,#20455,#20456,#20457,#20458));
#4665=EDGE_LOOP('',(#20459,#20460,#20461,#20462));
#4666=EDGE_LOOP('',(#20463,#20464,#20465,#20466,#20467,#20468));
#4667=EDGE_LOOP('',(#20469,#20470,#20471,#20472,#20473));
#4668=EDGE_LOOP('',(#20474,#20475,#20476,#20477,#20478,#20479));
#4669=EDGE_LOOP('',(#20480,#20481,#20482,#20483));
#4670=EDGE_LOOP('',(#20484,#20485,#20486,#20487,#20488));
#4671=EDGE_LOOP('',(#20489,#20490,#20491,#20492,#20493,#20494));
#4672=EDGE_LOOP('',(#20495,#20496,#20497,#20498,#20499,#20500));
#4673=EDGE_LOOP('',(#20501,#20502,#20503,#20504));
#4674=EDGE_LOOP('',(#20505,#20506,#20507,#20508,#20509,#20510));
#4675=EDGE_LOOP('',(#20511,#20512,#20513,#20514,#20515));
#4676=EDGE_LOOP('',(#20516,#20517,#20518,#20519,#20520,#20521));
#4677=EDGE_LOOP('',(#20522,#20523,#20524,#20525,#20526));
#4678=EDGE_LOOP('',(#20527,#20528,#20529,#20530,#20531,#20532));
#4679=EDGE_LOOP('',(#20533,#20534,#20535,#20536));
#4680=EDGE_LOOP('',(#20537,#20538,#20539,#20540,#20541,#20542));
#4681=EDGE_LOOP('',(#20543,#20544,#20545,#20546,#20547));
#4682=EDGE_LOOP('',(#20548,#20549,#20550,#20551,#20552,#20553));
#4683=EDGE_LOOP('',(#20554,#20555,#20556,#20557));
#4684=EDGE_LOOP('',(#20558,#20559,#20560,#20561,#20562));
#4685=EDGE_LOOP('',(#20563,#20564,#20565,#20566,#20567,#20568));
#4686=EDGE_LOOP('',(#20569,#20570,#20571,#20572,#20573,#20574));
#4687=EDGE_LOOP('',(#20575,#20576,#20577,#20578,#20579));
#4688=EDGE_LOOP('',(#20580,#20581,#20582,#20583,#20584,#20585));
#4689=EDGE_LOOP('',(#20586,#20587,#20588,#20589));
#4690=EDGE_LOOP('',(#20590,#20591,#20592,#20593,#20594,#20595));
#4691=EDGE_LOOP('',(#20596,#20597,#20598,#20599,#20600));
#4692=EDGE_LOOP('',(#20601,#20602,#20603,#20604,#20605,#20606));
#4693=EDGE_LOOP('',(#20607,#20608,#20609,#20610));
#4694=EDGE_LOOP('',(#20611,#20612,#20613,#20614,#20615));
#4695=EDGE_LOOP('',(#20616,#20617,#20618,#20619,#20620,#20621));
#4696=EDGE_LOOP('',(#20622,#20623,#20624,#20625,#20626,#20627));
#4697=EDGE_LOOP('',(#20628,#20629,#20630,#20631));
#4698=EDGE_LOOP('',(#20632,#20633,#20634,#20635,#20636));
#4699=EDGE_LOOP('',(#20637,#20638,#20639,#20640,#20641,#20642));
#4700=EDGE_LOOP('',(#20643,#20644,#20645,#20646,#20647,#20648));
#4701=EDGE_LOOP('',(#20649,#20650,#20651,#20652,#20653));
#4702=EDGE_LOOP('',(#20654,#20655,#20656,#20657,#20658,#20659));
#4703=EDGE_LOOP('',(#20660,#20661,#20662,#20663));
#4704=EDGE_LOOP('',(#20664,#20665,#20666,#20667,#20668,#20669));
#4705=EDGE_LOOP('',(#20670,#20671,#20672,#20673,#20674));
#4706=EDGE_LOOP('',(#20675,#20676,#20677,#20678,#20679,#20680));
#4707=EDGE_LOOP('',(#20681,#20682,#20683,#20684,#20685));
#4708=EDGE_LOOP('',(#20686,#20687,#20688,#20689,#20690,#20691));
#4709=EDGE_LOOP('',(#20692,#20693,#20694,#20695));
#4710=EDGE_LOOP('',(#20696,#20697,#20698,#20699,#20700,#20701));
#4711=EDGE_LOOP('',(#20702,#20703,#20704,#20705,#20706));
#4712=EDGE_LOOP('',(#20707,#20708,#20709,#20710,#20711,#20712));
#4713=EDGE_LOOP('',(#20713,#20714,#20715,#20716,#20717));
#4714=EDGE_LOOP('',(#20718,#20719,#20720,#20721));
#4715=EDGE_LOOP('',(#20722,#20723,#20724,#20725,#20726));
#4716=EDGE_LOOP('',(#20727,#20728,#20729,#20730,#20731,#20732));
#4717=EDGE_LOOP('',(#20733,#20734,#20735,#20736,#20737));
#4718=EDGE_LOOP('',(#20738,#20739,#20740,#20741,#20742,#20743));
#4719=EDGE_LOOP('',(#20744,#20745,#20746,#20747));
#4720=EDGE_LOOP('',(#20748,#20749,#20750,#20751,#20752,#20753));
#4721=EDGE_LOOP('',(#20754,#20755,#20756,#20757,#20758));
#4722=EDGE_LOOP('',(#20759,#20760,#20761,#20762,#20763,#20764));
#4723=EDGE_LOOP('',(#20765,#20766,#20767,#20768,#20769));
#4724=EDGE_LOOP('',(#20770,#20771,#20772,#20773,#20774,#20775));
#4725=EDGE_LOOP('',(#20776,#20777,#20778,#20779));
#4726=EDGE_LOOP('',(#20780,#20781,#20782,#20783,#20784,#20785));
#4727=EDGE_LOOP('',(#20786,#20787,#20788,#20789,#20790));
#4728=EDGE_LOOP('',(#20791,#20792,#20793,#20794,#20795,#20796));
#4729=EDGE_LOOP('',(#20797,#20798,#20799,#20800,#20801));
#4730=EDGE_LOOP('',(#20802,#20803,#20804,#20805));
#4731=EDGE_LOOP('',(#20806,#20807,#20808,#20809,#20810));
#4732=EDGE_LOOP('',(#20811,#20812,#20813,#20814));
#4733=EDGE_LOOP('',(#20815,#20816,#20817,#20818));
#4734=EDGE_LOOP('',(#20819));
#4735=EDGE_LOOP('',(#20820,#20821,#20822,#20823,#20824,#20825));
#4736=EDGE_LOOP('',(#20826,#20827,#20828,#20829,#20830,#20831));
#4737=EDGE_LOOP('',(#20832,#20833,#20834,#20835));
#4738=EDGE_LOOP('',(#20836,#20837,#20838,#20839,#20840,#20841));
#4739=EDGE_LOOP('',(#20842,#20843,#20844,#20845,#20846,#20847));
#4740=EDGE_LOOP('',(#20848,#20849,#20850,#20851));
#4741=EDGE_LOOP('',(#20852,#20853,#20854,#20855,#20856,#20857));
#4742=EDGE_LOOP('',(#20858,#20859,#20860,#20861,#20862,#20863));
#4743=EDGE_LOOP('',(#20864,#20865,#20866,#20867,#20868,#20869));
#4744=EDGE_LOOP('',(#20870,#20871,#20872,#20873));
#4745=EDGE_LOOP('',(#20874,#20875,#20876,#20877,#20878,#20879));
#4746=EDGE_LOOP('',(#20880,#20881,#20882,#20883,#20884));
#4747=EDGE_LOOP('',(#20885,#20886,#20887,#20888,#20889,#20890));
#4748=EDGE_LOOP('',(#20891,#20892,#20893,#20894));
#4749=EDGE_LOOP('',(#20895,#20896,#20897,#20898,#20899,#20900));
#4750=EDGE_LOOP('',(#20901,#20902,#20903,#20904,#20905));
#4751=EDGE_LOOP('',(#20906,#20907,#20908,#20909,#20910,#20911));
#4752=EDGE_LOOP('',(#20912,#20913,#20914,#20915,#20916));
#4753=EDGE_LOOP('',(#20917,#20918,#20919,#20920,#20921,#20922));
#4754=EDGE_LOOP('',(#20923,#20924,#20925,#20926));
#4755=EDGE_LOOP('',(#20927,#20928,#20929,#20930,#20931,#20932));
#4756=EDGE_LOOP('',(#20933,#20934,#20935,#20936,#20937));
#4757=EDGE_LOOP('',(#20938,#20939,#20940,#20941,#20942,#20943));
#4758=EDGE_LOOP('',(#20944,#20945,#20946,#20947,#20948));
#4759=EDGE_LOOP('',(#20949,#20950,#20951,#20952,#20953,#20954));
#4760=EDGE_LOOP('',(#20955,#20956,#20957,#20958));
#4761=EDGE_LOOP('',(#20959,#20960,#20961,#20962,#20963,#20964));
#4762=EDGE_LOOP('',(#20965,#20966,#20967,#20968,#20969));
#4763=EDGE_LOOP('',(#20970,#20971,#20972,#20973,#20974,#20975));
#4764=EDGE_LOOP('',(#20976,#20977,#20978,#20979,#20980));
#4765=EDGE_LOOP('',(#20981,#20982,#20983,#20984,#20985,#20986));
#4766=EDGE_LOOP('',(#20987,#20988,#20989,#20990));
#4767=EDGE_LOOP('',(#20991,#20992,#20993,#20994,#20995,#20996));
#4768=EDGE_LOOP('',(#20997,#20998,#20999,#21000,#21001));
#4769=EDGE_LOOP('',(#21002,#21003,#21004,#21005,#21006,#21007));
#4770=EDGE_LOOP('',(#21008,#21009,#21010,#21011));
#4771=EDGE_LOOP('',(#21012,#21013,#21014,#21015,#21016));
#4772=EDGE_LOOP('',(#21017,#21018,#21019,#21020,#21021,#21022));
#4773=EDGE_LOOP('',(#21023,#21024,#21025,#21026));
#4774=EDGE_LOOP('',(#21027,#21028,#21029,#21030));
#4775=EDGE_LOOP('',(#21031,#21032,#21033,#21034));
#4776=EDGE_LOOP('',(#21035,#21036,#21037,#21038));
#4777=EDGE_LOOP('',(#21039,#21040,#21041,#21042));
#4778=EDGE_LOOP('',(#21043,#21044,#21045,#21046));
#4779=EDGE_LOOP('',(#21047,#21048,#21049,#21050));
#4780=EDGE_LOOP('',(#21051,#21052,#21053,#21054));
#4781=EDGE_LOOP('',(#21055,#21056,#21057,#21058));
#4782=EDGE_LOOP('',(#21059,#21060,#21061,#21062));
#4783=EDGE_LOOP('',(#21063,#21064,#21065,#21066,#21067,#21068,#21069,#21070,
#21071,#21072,#21073,#21074,#21075,#21076,#21077,#21078,#21079,#21080,#21081,
#21082,#21083,#21084,#21085,#21086,#21087,#21088,#21089,#21090,#21091,#21092,
#21093,#21094,#21095,#21096,#21097,#21098,#21099,#21100,#21101,#21102,#21103,
#21104,#21105,#21106,#21107,#21108,#21109,#21110,#21111,#21112,#21113,#21114,
#21115,#21116,#21117,#21118,#21119,#21120,#21121,#21122,#21123,#21124,#21125,
#21126,#21127,#21128,#21129,#21130,#21131,#21132,#21133,#21134,#21135,#21136,
#21137,#21138,#21139,#21140,#21141,#21142,#21143,#21144,#21145,#21146,#21147,
#21148,#21149,#21150,#21151,#21152,#21153,#21154,#21155,#21156,#21157,#21158,
#21159,#21160,#21161,#21162,#21163,#21164,#21165,#21166,#21167,#21168,#21169,
#21170,#21171,#21172,#21173,#21174,#21175,#21176,#21177,#21178,#21179,#21180,
#21181,#21182,#21183,#21184,#21185,#21186,#21187,#21188,#21189,#21190,#21191,
#21192,#21193,#21194));
#4784=EDGE_LOOP('',(#21195,#21196,#21197,#21198));
#4785=EDGE_LOOP('',(#21199,#21200,#21201,#21202));
#4786=EDGE_LOOP('',(#21203,#21204,#21205,#21206));
#4787=EDGE_LOOP('',(#21207,#21208,#21209,#21210));
#4788=EDGE_LOOP('',(#21211,#21212,#21213,#21214));
#4789=EDGE_LOOP('',(#21215,#21216,#21217,#21218));
#4790=EDGE_LOOP('',(#21219,#21220,#21221,#21222));
#4791=EDGE_LOOP('',(#21223,#21224,#21225,#21226));
#4792=EDGE_LOOP('',(#21227,#21228,#21229,#21230));
#4793=EDGE_LOOP('',(#21231,#21232,#21233,#21234));
#4794=EDGE_LOOP('',(#21235,#21236,#21237,#21238));
#4795=EDGE_LOOP('',(#21239,#21240,#21241,#21242));
#4796=EDGE_LOOP('',(#21243,#21244,#21245,#21246));
#4797=EDGE_LOOP('',(#21247,#21248,#21249,#21250));
#4798=EDGE_LOOP('',(#21251,#21252,#21253,#21254));
#4799=EDGE_LOOP('',(#21255,#21256,#21257,#21258));
#4800=EDGE_LOOP('',(#21259,#21260,#21261,#21262));
#4801=EDGE_LOOP('',(#21263,#21264,#21265,#21266));
#4802=EDGE_LOOP('',(#21267,#21268,#21269,#21270));
#4803=EDGE_LOOP('',(#21271,#21272,#21273,#21274,#21275));
#4804=EDGE_LOOP('',(#21276,#21277,#21278,#21279));
#4805=EDGE_LOOP('',(#21280,#21281,#21282,#21283,#21284,#21285));
#4806=EDGE_LOOP('',(#21286,#21287,#21288,#21289,#21290,#21291));
#4807=EDGE_LOOP('',(#21292,#21293,#21294,#21295,#21296,#21297));
#4808=EDGE_LOOP('',(#21298,#21299,#21300,#21301,#21302,#21303));
#4809=EDGE_LOOP('',(#21304,#21305,#21306,#21307,#21308));
#4810=EDGE_LOOP('',(#21309,#21310,#21311,#21312,#21313,#21314));
#4811=EDGE_LOOP('',(#21315,#21316,#21317,#21318,#21319));
#4812=EDGE_LOOP('',(#21320,#21321,#21322,#21323,#21324,#21325));
#4813=EDGE_LOOP('',(#21326,#21327,#21328,#21329));
#4814=EDGE_LOOP('',(#21330,#21331,#21332,#21333,#21334,#21335));
#4815=EDGE_LOOP('',(#21336,#21337,#21338,#21339,#21340));
#4816=EDGE_LOOP('',(#21341,#21342,#21343,#21344));
#4817=EDGE_LOOP('',(#21345,#21346,#21347,#21348));
#4818=EDGE_LOOP('',(#21349,#21350,#21351,#21352));
#4819=EDGE_LOOP('',(#21353,#21354,#21355,#21356));
#4820=EDGE_LOOP('',(#21357,#21358,#21359,#21360));
#4821=EDGE_LOOP('',(#21361,#21362,#21363,#21364));
#4822=EDGE_LOOP('',(#21365,#21366,#21367,#21368));
#4823=EDGE_LOOP('',(#21369,#21370,#21371,#21372));
#4824=EDGE_LOOP('',(#21373,#21374,#21375,#21376));
#4825=EDGE_LOOP('',(#21377,#21378,#21379,#21380));
#4826=EDGE_LOOP('',(#21381,#21382,#21383,#21384));
#4827=EDGE_LOOP('',(#21385,#21386,#21387,#21388));
#4828=EDGE_LOOP('',(#21389,#21390,#21391,#21392,#21393));
#4829=EDGE_LOOP('',(#21394,#21395,#21396,#21397));
#4830=EDGE_LOOP('',(#21398,#21399,#21400,#21401));
#4831=EDGE_LOOP('',(#21402,#21403,#21404,#21405));
#4832=EDGE_LOOP('',(#21406,#21407,#21408,#21409));
#4833=EDGE_LOOP('',(#21410,#21411,#21412,#21413));
#4834=EDGE_LOOP('',(#21414,#21415,#21416,#21417));
#4835=EDGE_LOOP('',(#21418,#21419,#21420,#21421));
#4836=EDGE_LOOP('',(#21422,#21423,#21424,#21425));
#4837=EDGE_LOOP('',(#21426,#21427,#21428,#21429));
#4838=EDGE_LOOP('',(#21430,#21431,#21432,#21433));
#4839=EDGE_LOOP('',(#21434,#21435,#21436,#21437));
#4840=EDGE_LOOP('',(#21438,#21439,#21440,#21441));
#4841=EDGE_LOOP('',(#21442,#21443,#21444,#21445));
#4842=EDGE_LOOP('',(#21446,#21447,#21448,#21449));
#4843=EDGE_LOOP('',(#21450,#21451,#21452,#21453));
#4844=EDGE_LOOP('',(#21454,#21455,#21456,#21457));
#4845=EDGE_LOOP('',(#21458,#21459,#21460,#21461,#21462,#21463));
#4846=EDGE_LOOP('',(#21464,#21465,#21466,#21467,#21468));
#4847=EDGE_LOOP('',(#21469,#21470,#21471,#21472,#21473,#21474));
#4848=EDGE_LOOP('',(#21475,#21476,#21477,#21478));
#4849=EDGE_LOOP('',(#21479,#21480,#21481,#21482,#21483,#21484));
#4850=EDGE_LOOP('',(#21485,#21486,#21487,#21488,#21489));
#4851=EDGE_LOOP('',(#21490,#21491,#21492,#21493,#21494,#21495));
#4852=EDGE_LOOP('',(#21496,#21497,#21498,#21499,#21500));
#4853=EDGE_LOOP('',(#21501,#21502,#21503,#21504,#21505,#21506));
#4854=EDGE_LOOP('',(#21507,#21508,#21509,#21510));
#4855=EDGE_LOOP('',(#21511,#21512,#21513,#21514,#21515,#21516));
#4856=EDGE_LOOP('',(#21517,#21518,#21519,#21520,#21521));
#4857=EDGE_LOOP('',(#21522,#21523,#21524,#21525,#21526,#21527));
#4858=EDGE_LOOP('',(#21528,#21529,#21530,#21531,#21532));
#4859=EDGE_LOOP('',(#21533,#21534,#21535,#21536,#21537,#21538));
#4860=EDGE_LOOP('',(#21539,#21540,#21541,#21542));
#4861=EDGE_LOOP('',(#21543,#21544,#21545,#21546,#21547,#21548));
#4862=EDGE_LOOP('',(#21549,#21550,#21551,#21552,#21553));
#4863=EDGE_LOOP('',(#21554,#21555,#21556,#21557,#21558,#21559));
#4864=EDGE_LOOP('',(#21560,#21561,#21562,#21563));
#4865=EDGE_LOOP('',(#21564,#21565,#21566,#21567,#21568));
#4866=EDGE_LOOP('',(#21569,#21570,#21571,#21572,#21573,#21574));
#4867=EDGE_LOOP('',(#21575,#21576,#21577,#21578,#21579,#21580));
#4868=EDGE_LOOP('',(#21581,#21582,#21583,#21584));
#4869=EDGE_LOOP('',(#21585,#21586,#21587,#21588,#21589));
#4870=EDGE_LOOP('',(#21590,#21591,#21592,#21593,#21594,#21595));
#4871=EDGE_LOOP('',(#21596,#21597,#21598,#21599,#21600,#21601));
#4872=EDGE_LOOP('',(#21602,#21603,#21604,#21605,#21606));
#4873=EDGE_LOOP('',(#21607,#21608,#21609,#21610,#21611,#21612));
#4874=EDGE_LOOP('',(#21613,#21614,#21615,#21616));
#4875=EDGE_LOOP('',(#21617,#21618,#21619,#21620,#21621,#21622));
#4876=EDGE_LOOP('',(#21623,#21624,#21625,#21626,#21627));
#4877=EDGE_LOOP('',(#21628,#21629,#21630,#21631,#21632,#21633));
#4878=EDGE_LOOP('',(#21634,#21635,#21636,#21637,#21638));
#4879=EDGE_LOOP('',(#21639,#21640,#21641,#21642,#21643,#21644));
#4880=EDGE_LOOP('',(#21645,#21646,#21647,#21648));
#4881=EDGE_LOOP('',(#21649,#21650,#21651,#21652,#21653,#21654));
#4882=EDGE_LOOP('',(#21655,#21656,#21657,#21658,#21659));
#4883=EDGE_LOOP('',(#21660,#21661,#21662,#21663,#21664,#21665));
#4884=EDGE_LOOP('',(#21666,#21667,#21668,#21669,#21670));
#4885=EDGE_LOOP('',(#21671,#21672,#21673,#21674));
#4886=EDGE_LOOP('',(#21675,#21676,#21677,#21678,#21679));
#4887=EDGE_LOOP('',(#21680,#21681,#21682,#21683));
#4888=EDGE_LOOP('',(#21684,#21685,#21686,#21687));
#4889=EDGE_LOOP('',(#21688,#21689,#21690,#21691));
#4890=EDGE_LOOP('',(#21692,#21693,#21694,#21695));
#4891=EDGE_LOOP('',(#21696,#21697,#21698,#21699));
#4892=EDGE_LOOP('',(#21700,#21701,#21702,#21703));
#4893=EDGE_LOOP('',(#21704,#21705,#21706,#21707));
#4894=EDGE_LOOP('',(#21708,#21709,#21710,#21711,#21712));
#4895=EDGE_LOOP('',(#21713,#21714,#21715,#21716));
#4896=EDGE_LOOP('',(#21717,#21718,#21719,#21720));
#4897=EDGE_LOOP('',(#21721,#21722,#21723,#21724));
#4898=EDGE_LOOP('',(#21725,#21726,#21727,#21728));
#4899=EDGE_LOOP('',(#21729,#21730,#21731,#21732));
#4900=EDGE_LOOP('',(#21733,#21734,#21735,#21736));
#4901=EDGE_LOOP('',(#21737,#21738,#21739,#21740));
#4902=EDGE_LOOP('',(#21741,#21742,#21743,#21744));
#4903=EDGE_LOOP('',(#21745,#21746,#21747,#21748));
#4904=EDGE_LOOP('',(#21749,#21750,#21751,#21752));
#4905=EDGE_LOOP('',(#21753,#21754,#21755,#21756));
#4906=EDGE_LOOP('',(#21757,#21758,#21759,#21760));
#4907=EDGE_LOOP('',(#21761,#21762,#21763,#21764));
#4908=EDGE_LOOP('',(#21765,#21766,#21767,#21768));
#4909=EDGE_LOOP('',(#21769,#21770,#21771,#21772));
#4910=EDGE_LOOP('',(#21773,#21774,#21775,#21776));
#4911=EDGE_LOOP('',(#21777,#21778,#21779,#21780));
#4912=EDGE_LOOP('',(#21781,#21782,#21783,#21784));
#4913=EDGE_LOOP('',(#21785,#21786,#21787,#21788));
#4914=EDGE_LOOP('',(#21789,#21790,#21791,#21792));
#4915=EDGE_LOOP('',(#21793,#21794,#21795,#21796));
#4916=EDGE_LOOP('',(#21797,#21798,#21799,#21800));
#4917=EDGE_LOOP('',(#21801,#21802,#21803,#21804));
#4918=EDGE_LOOP('',(#21805,#21806,#21807,#21808));
#4919=EDGE_LOOP('',(#21809,#21810,#21811,#21812,#21813,#21814));
#4920=EDGE_LOOP('',(#21815,#21816,#21817,#21818,#21819));
#4921=EDGE_LOOP('',(#21820,#21821,#21822,#21823,#21824,#21825));
#4922=EDGE_LOOP('',(#21826,#21827,#21828,#21829));
#4923=EDGE_LOOP('',(#21830,#21831,#21832,#21833,#21834,#21835));
#4924=EDGE_LOOP('',(#21836,#21837,#21838,#21839,#21840));
#4925=EDGE_LOOP('',(#21841,#21842,#21843,#21844,#21845,#21846));
#4926=EDGE_LOOP('',(#21847,#21848,#21849,#21850,#21851));
#4927=EDGE_LOOP('',(#21852,#21853,#21854,#21855,#21856,#21857));
#4928=EDGE_LOOP('',(#21858,#21859,#21860,#21861));
#4929=EDGE_LOOP('',(#21862,#21863,#21864,#21865,#21866,#21867));
#4930=EDGE_LOOP('',(#21868,#21869,#21870,#21871,#21872));
#4931=EDGE_LOOP('',(#21873,#21874,#21875,#21876,#21877,#21878));
#4932=EDGE_LOOP('',(#21879,#21880,#21881,#21882,#21883));
#4933=EDGE_LOOP('',(#21884,#21885,#21886,#21887,#21888,#21889));
#4934=EDGE_LOOP('',(#21890,#21891,#21892,#21893));
#4935=EDGE_LOOP('',(#21894,#21895,#21896,#21897,#21898,#21899));
#4936=EDGE_LOOP('',(#21900,#21901,#21902,#21903,#21904));
#4937=EDGE_LOOP('',(#21905,#21906,#21907,#21908,#21909,#21910));
#4938=EDGE_LOOP('',(#21911,#21912,#21913,#21914,#21915));
#4939=EDGE_LOOP('',(#21916,#21917,#21918,#21919,#21920,#21921));
#4940=EDGE_LOOP('',(#21922,#21923,#21924,#21925));
#4941=EDGE_LOOP('',(#21926,#21927,#21928,#21929,#21930,#21931));
#4942=EDGE_LOOP('',(#21932,#21933,#21934,#21935,#21936));
#4943=EDGE_LOOP('',(#21937,#21938,#21939,#21940,#21941,#21942));
#4944=EDGE_LOOP('',(#21943,#21944,#21945,#21946,#21947));
#4945=EDGE_LOOP('',(#21948,#21949,#21950,#21951,#21952,#21953));
#4946=EDGE_LOOP('',(#21954,#21955,#21956,#21957));
#4947=EDGE_LOOP('',(#21958,#21959,#21960,#21961,#21962,#21963));
#4948=EDGE_LOOP('',(#21964,#21965,#21966,#21967,#21968));
#4949=EDGE_LOOP('',(#21969,#21970,#21971,#21972,#21973,#21974));
#4950=EDGE_LOOP('',(#21975,#21976,#21977,#21978,#21979));
#4951=EDGE_LOOP('',(#21980,#21981,#21982,#21983,#21984,#21985));
#4952=EDGE_LOOP('',(#21986,#21987,#21988,#21989));
#4953=EDGE_LOOP('',(#21990,#21991,#21992,#21993,#21994,#21995));
#4954=EDGE_LOOP('',(#21996,#21997,#21998,#21999,#22000));
#4955=EDGE_LOOP('',(#22001,#22002,#22003,#22004,#22005,#22006));
#4956=EDGE_LOOP('',(#22007,#22008,#22009,#22010,#22011));
#4957=EDGE_LOOP('',(#22012,#22013,#22014,#22015));
#4958=EDGE_LOOP('',(#22016,#22017,#22018,#22019,#22020));
#4959=EDGE_LOOP('',(#22021,#22022,#22023,#22024));
#4960=EDGE_LOOP('',(#22025,#22026,#22027,#22028));
#4961=EDGE_LOOP('',(#22029,#22030,#22031,#22032));
#4962=EDGE_LOOP('',(#22033,#22034,#22035,#22036));
#4963=EDGE_LOOP('',(#22037,#22038,#22039,#22040));
#4964=EDGE_LOOP('',(#22041,#22042,#22043,#22044));
#4965=EDGE_LOOP('',(#22045,#22046,#22047,#22048));
#4966=EDGE_LOOP('',(#22049,#22050,#22051,#22052));
#4967=EDGE_LOOP('',(#22053,#22054,#22055,#22056));
#4968=EDGE_LOOP('',(#22057,#22058,#22059,#22060));
#4969=EDGE_LOOP('',(#22061,#22062,#22063,#22064));
#4970=EDGE_LOOP('',(#22065,#22066,#22067,#22068));
#4971=EDGE_LOOP('',(#22069,#22070,#22071,#22072));
#4972=EDGE_LOOP('',(#22073,#22074,#22075,#22076));
#4973=EDGE_LOOP('',(#22077,#22078,#22079,#22080));
#4974=EDGE_LOOP('',(#22081,#22082,#22083,#22084));
#4975=EDGE_LOOP('',(#22085,#22086,#22087,#22088));
#4976=EDGE_LOOP('',(#22089,#22090,#22091,#22092));
#4977=EDGE_LOOP('',(#22093,#22094,#22095,#22096));
#4978=EDGE_LOOP('',(#22097,#22098,#22099,#22100));
#4979=EDGE_LOOP('',(#22101,#22102,#22103,#22104));
#4980=EDGE_LOOP('',(#22105,#22106,#22107,#22108));
#4981=EDGE_LOOP('',(#22109,#22110,#22111,#22112));
#4982=EDGE_LOOP('',(#22113,#22114,#22115,#22116));
#4983=EDGE_LOOP('',(#22117,#22118,#22119,#22120));
#4984=EDGE_LOOP('',(#22121,#22122,#22123,#22124));
#4985=EDGE_LOOP('',(#22125,#22126,#22127,#22128,#22129));
#4986=EDGE_LOOP('',(#22130,#22131,#22132,#22133,#22134));
#4987=EDGE_LOOP('',(#22135,#22136,#22137,#22138));
#4988=EDGE_LOOP('',(#22139,#22140,#22141,#22142,#22143));
#4989=EDGE_LOOP('',(#22144,#22145,#22146,#22147,#22148,#22149,#22150,#22151,
#22152,#22153,#22154,#22155,#22156,#22157,#22158,#22159,#22160,#22161,#22162,
#22163,#22164,#22165,#22166,#22167,#22168,#22169,#22170,#22171,#22172,#22173,
#22174,#22175,#22176,#22177,#22178,#22179,#22180,#22181,#22182,#22183,#22184,
#22185,#22186,#22187,#22188,#22189,#22190,#22191,#22192,#22193,#22194,#22195,
#22196,#22197,#22198,#22199,#22200,#22201,#22202,#22203,#22204,#22205,#22206,
#22207,#22208,#22209,#22210,#22211,#22212,#22213,#22214,#22215,#22216,#22217,
#22218,#22219,#22220,#22221,#22222,#22223,#22224,#22225,#22226,#22227,#22228,
#22229,#22230,#22231,#22232,#22233,#22234,#22235,#22236,#22237,#22238,#22239,
#22240,#22241,#22242,#22243,#22244,#22245,#22246,#22247,#22248,#22249,#22250,
#22251,#22252,#22253,#22254,#22255,#22256,#22257,#22258,#22259,#22260,#22261,
#22262,#22263,#22264,#22265,#22266,#22267,#22268,#22269,#22270,#22271,#22272,
#22273,#22274,#22275));
#4990=EDGE_LOOP('',(#22276));
#4991=EDGE_LOOP('',(#22277,#22278,#22279,#22280,#22281,#22282));
#4992=EDGE_LOOP('',(#22283,#22284,#22285,#22286,#22287));
#4993=EDGE_LOOP('',(#22288,#22289,#22290,#22291));
#4994=EDGE_LOOP('',(#22292,#22293,#22294,#22295,#22296));
#4995=EDGE_LOOP('',(#22297,#22298,#22299,#22300,#22301,#22302));
#4996=EDGE_LOOP('',(#22303,#22304,#22305,#22306,#22307));
#4997=EDGE_LOOP('',(#22308,#22309,#22310,#22311));
#4998=EDGE_LOOP('',(#22312,#22313,#22314,#22315,#22316));
#4999=EDGE_LOOP('',(#22317,#22318,#22319,#22320,#22321,#22322));
#5000=EDGE_LOOP('',(#22323,#22324,#22325,#22326,#22327));
#5001=EDGE_LOOP('',(#22328,#22329,#22330,#22331));
#5002=EDGE_LOOP('',(#22332,#22333,#22334,#22335,#22336));
#5003=EDGE_LOOP('',(#22337,#22338,#22339,#22340,#22341,#22342));
#5004=EDGE_LOOP('',(#22343,#22344,#22345,#22346));
#5005=EDGE_LOOP('',(#22347,#22348,#22349,#22350,#22351));
#5006=EDGE_LOOP('',(#22352,#22353,#22354,#22355,#22356,#22357));
#5007=EDGE_LOOP('',(#22358,#22359,#22360,#22361,#22362));
#5008=EDGE_LOOP('',(#22363,#22364,#22365,#22366));
#5009=EDGE_LOOP('',(#22367,#22368,#22369,#22370,#22371));
#5010=EDGE_LOOP('',(#22372,#22373,#22374,#22375,#22376,#22377));
#5011=EDGE_LOOP('',(#22378,#22379,#22380,#22381,#22382));
#5012=EDGE_LOOP('',(#22383,#22384,#22385,#22386));
#5013=EDGE_LOOP('',(#22387,#22388,#22389,#22390));
#5014=EDGE_LOOP('',(#22391,#22392,#22393,#22394,#22395));
#5015=EDGE_LOOP('',(#22396,#22397,#22398,#22399,#22400));
#5016=EDGE_LOOP('',(#22401,#22402,#22403,#22404));
#5017=EDGE_LOOP('',(#22405,#22406,#22407,#22408,#22409));
#5018=EDGE_LOOP('',(#22410,#22411,#22412,#22413,#22414,#22415));
#5019=EDGE_LOOP('',(#22416,#22417,#22418,#22419,#22420));
#5020=EDGE_LOOP('',(#22421,#22422,#22423,#22424));
#5021=EDGE_LOOP('',(#22425,#22426,#22427,#22428,#22429));
#5022=EDGE_LOOP('',(#22430,#22431,#22432,#22433,#22434,#22435));
#5023=EDGE_LOOP('',(#22436,#22437,#22438,#22439,#22440));
#5024=EDGE_LOOP('',(#22441,#22442,#22443,#22444));
#5025=EDGE_LOOP('',(#22445,#22446,#22447,#22448,#22449));
#5026=EDGE_LOOP('',(#22450,#22451,#22452,#22453,#22454,#22455));
#5027=EDGE_LOOP('',(#22456,#22457,#22458,#22459,#22460));
#5028=EDGE_LOOP('',(#22461,#22462,#22463,#22464));
#5029=EDGE_LOOP('',(#22465,#22466,#22467,#22468,#22469));
#5030=EDGE_LOOP('',(#22470,#22471,#22472,#22473,#22474,#22475));
#5031=EDGE_LOOP('',(#22476,#22477,#22478,#22479,#22480));
#5032=EDGE_LOOP('',(#22481,#22482,#22483,#22484));
#5033=EDGE_LOOP('',(#22485,#22486,#22487,#22488,#22489));
#5034=EDGE_LOOP('',(#22490,#22491,#22492,#22493,#22494,#22495));
#5035=EDGE_LOOP('',(#22496,#22497,#22498,#22499,#22500));
#5036=EDGE_LOOP('',(#22501,#22502,#22503,#22504));
#5037=EDGE_LOOP('',(#22505,#22506,#22507,#22508,#22509,#22510));
#5038=EDGE_LOOP('',(#22511,#22512,#22513,#22514,#22515));
#5039=EDGE_LOOP('',(#22516,#22517,#22518,#22519));
#5040=EDGE_LOOP('',(#22520,#22521,#22522,#22523,#22524));
#5041=EDGE_LOOP('',(#22525,#22526,#22527,#22528,#22529,#22530));
#5042=EDGE_LOOP('',(#22531,#22532,#22533,#22534,#22535));
#5043=EDGE_LOOP('',(#22536,#22537,#22538,#22539));
#5044=EDGE_LOOP('',(#22540,#22541,#22542,#22543,#22544));
#5045=EDGE_LOOP('',(#22545,#22546,#22547,#22548,#22549,#22550));
#5046=EDGE_LOOP('',(#22551,#22552,#22553,#22554));
#5047=EDGE_LOOP('',(#22555,#22556,#22557,#22558,#22559));
#5048=EDGE_LOOP('',(#22560,#22561,#22562,#22563,#22564,#22565));
#5049=EDGE_LOOP('',(#22566,#22567,#22568,#22569,#22570));
#5050=EDGE_LOOP('',(#22571,#22572,#22573,#22574));
#5051=EDGE_LOOP('',(#22575,#22576,#22577,#22578,#22579));
#5052=EDGE_LOOP('',(#22580,#22581,#22582,#22583,#22584,#22585));
#5053=EDGE_LOOP('',(#22586,#22587,#22588,#22589,#22590));
#5054=EDGE_LOOP('',(#22591,#22592,#22593,#22594));
#5055=EDGE_LOOP('',(#22595,#22596,#22597,#22598,#22599));
#5056=EDGE_LOOP('',(#22600,#22601,#22602,#22603,#22604,#22605));
#5057=EDGE_LOOP('',(#22606,#22607,#22608,#22609,#22610));
#5058=EDGE_LOOP('',(#22611,#22612,#22613,#22614));
#5059=EDGE_LOOP('',(#22615,#22616,#22617,#22618,#22619));
#5060=EDGE_LOOP('',(#22620,#22621,#22622,#22623));
#5061=EDGE_LOOP('',(#22624,#22625,#22626,#22627,#22628));
#5062=EDGE_LOOP('',(#22629,#22630,#22631,#22632,#22633));
#5063=EDGE_LOOP('',(#22634,#22635,#22636,#22637));
#5064=EDGE_LOOP('',(#22638,#22639,#22640,#22641,#22642));
#5065=EDGE_LOOP('',(#22643,#22644,#22645,#22646,#22647,#22648));
#5066=EDGE_LOOP('',(#22649,#22650,#22651,#22652,#22653));
#5067=EDGE_LOOP('',(#22654,#22655,#22656,#22657));
#5068=EDGE_LOOP('',(#22658,#22659,#22660,#22661,#22662,#22663));
#5069=EDGE_LOOP('',(#22664,#22665,#22666,#22667,#22668));
#5070=EDGE_LOOP('',(#22669,#22670,#22671,#22672));
#5071=EDGE_LOOP('',(#22673,#22674,#22675,#22676,#22677));
#5072=EDGE_LOOP('',(#22678,#22679,#22680,#22681,#22682,#22683));
#5073=EDGE_LOOP('',(#22684,#22685,#22686,#22687,#22688));
#5074=EDGE_LOOP('',(#22689,#22690,#22691,#22692));
#5075=EDGE_LOOP('',(#22693,#22694,#22695,#22696,#22697));
#5076=EDGE_LOOP('',(#22698,#22699,#22700,#22701,#22702,#22703));
#5077=EDGE_LOOP('',(#22704,#22705,#22706,#22707));
#5078=EDGE_LOOP('',(#22708,#22709,#22710,#22711,#22712));
#5079=EDGE_LOOP('',(#22713,#22714,#22715,#22716,#22717,#22718));
#5080=EDGE_LOOP('',(#22719,#22720,#22721,#22722,#22723));
#5081=EDGE_LOOP('',(#22724,#22725,#22726,#22727));
#5082=EDGE_LOOP('',(#22728,#22729,#22730,#22731,#22732));
#5083=EDGE_LOOP('',(#22733,#22734,#22735,#22736));
#5084=EDGE_LOOP('',(#22737,#22738,#22739,#22740,#22741));
#5085=EDGE_LOOP('',(#22742,#22743,#22744,#22745,#22746));
#5086=EDGE_LOOP('',(#22747,#22748,#22749,#22750));
#5087=EDGE_LOOP('',(#22751,#22752,#22753,#22754,#22755));
#5088=EDGE_LOOP('',(#22756,#22757,#22758,#22759,#22760,#22761));
#5089=EDGE_LOOP('',(#22762,#22763,#22764,#22765,#22766));
#5090=EDGE_LOOP('',(#22767,#22768,#22769,#22770));
#5091=EDGE_LOOP('',(#22771,#22772,#22773,#22774,#22775,#22776));
#5092=EDGE_LOOP('',(#22777,#22778,#22779,#22780,#22781,#22782));
#5093=EDGE_LOOP('',(#22783,#22784,#22785,#22786,#22787));
#5094=EDGE_LOOP('',(#22788,#22789,#22790,#22791));
#5095=EDGE_LOOP('',(#22792,#22793,#22794,#22795,#22796));
#5096=EDGE_LOOP('',(#22797,#22798,#22799,#22800,#22801,#22802));
#5097=EDGE_LOOP('',(#22803,#22804,#22805,#22806,#22807));
#5098=EDGE_LOOP('',(#22808,#22809,#22810,#22811));
#5099=EDGE_LOOP('',(#22812,#22813,#22814,#22815,#22816));
#5100=EDGE_LOOP('',(#22817,#22818,#22819,#22820,#22821,#22822));
#5101=EDGE_LOOP('',(#22823,#22824,#22825,#22826,#22827));
#5102=EDGE_LOOP('',(#22828,#22829,#22830,#22831,#22832));
#5103=EDGE_LOOP('',(#22833,#22834,#22835,#22836));
#5104=EDGE_LOOP('',(#22837));
#5105=EDGE_LOOP('',(#22838,#22839,#22840,#22841));
#5106=EDGE_LOOP('',(#22842,#22843,#22844,#22845));
#5107=EDGE_LOOP('',(#22846,#22847,#22848));
#5108=EDGE_LOOP('',(#22849,#22850,#22851,#22852,#22853,#22854));
#5109=EDGE_LOOP('',(#22855,#22856,#22857,#22858,#22859,#22860));
#5110=EDGE_LOOP('',(#22861,#22862,#22863,#22864));
#5111=EDGE_LOOP('',(#22865,#22866,#22867,#22868));
#5112=EDGE_LOOP('',(#22869,#22870,#22871,#22872));
#5113=EDGE_LOOP('',(#22873,#22874,#22875,#22876));
#5114=EDGE_LOOP('',(#22877,#22878,#22879,#22880));
#5115=EDGE_LOOP('',(#22881,#22882,#22883,#22884));
#5116=EDGE_LOOP('',(#22885,#22886,#22887,#22888));
#5117=EDGE_LOOP('',(#22889,#22890,#22891,#22892,#22893,#22894));
#5118=EDGE_LOOP('',(#22895,#22896,#22897,#22898,#22899,#22900));
#5119=EDGE_LOOP('',(#22901,#22902,#22903,#22904,#22905,#22906));
#5120=EDGE_LOOP('',(#22907,#22908,#22909,#22910,#22911,#22912));
#5121=EDGE_LOOP('',(#22913,#22914,#22915,#22916,#22917));
#5122=EDGE_LOOP('',(#22918,#22919,#22920,#22921,#22922,#22923,#22924,#22925));
#5123=EDGE_LOOP('',(#22926,#22927,#22928,#22929));
#5124=EDGE_LOOP('',(#22930,#22931,#22932,#22933,#22934,#22935));
#5125=EDGE_LOOP('',(#22936,#22937,#22938,#22939));
#5126=EDGE_LOOP('',(#22940,#22941,#22942,#22943));
#6249=LINE('',#60850,#8746);
#6250=LINE('',#60852,#8747);
#6251=LINE('',#60854,#8748);
#6252=LINE('',#60856,#8749);
#6253=LINE('',#60858,#8750);
#6254=LINE('',#60859,#8751);
#6255=LINE('',#60862,#8752);
#6256=LINE('',#60864,#8753);
#6257=LINE('',#60866,#8754);
#6258=LINE('',#60867,#8755);
#6259=LINE('',#60870,#8756);
#6260=LINE('',#60871,#8757);
#6261=LINE('',#60874,#8758);
#6262=LINE('',#60876,#8759);
#6263=LINE('',#60877,#8760);
#6264=LINE('',#60881,#8761);
#6265=LINE('',#60883,#8762);
#6266=LINE('',#60885,#8763);
#6267=LINE('',#60887,#8764);
#6268=LINE('',#60889,#8765);
#6269=LINE('',#60890,#8766);
#6270=LINE('',#60893,#8767);
#6271=LINE('',#60895,#8768);
#6272=LINE('',#60897,#8769);
#6273=LINE('',#60898,#8770);
#6274=LINE('',#60901,#8771);
#6275=LINE('',#60902,#8772);
#6276=LINE('',#60905,#8773);
#6277=LINE('',#60907,#8774);
#6278=LINE('',#60908,#8775);
#6279=LINE('',#60912,#8776);
#6280=LINE('',#60914,#8777);
#6281=LINE('',#60916,#8778);
#6282=LINE('',#60918,#8779);
#6283=LINE('',#60920,#8780);
#6284=LINE('',#60921,#8781);
#6285=LINE('',#60924,#8782);
#6286=LINE('',#60926,#8783);
#6287=LINE('',#60927,#8784);
#6288=LINE('',#60930,#8785);
#6289=LINE('',#60932,#8786);
#6290=LINE('',#60933,#8787);
#6291=LINE('',#60936,#8788);
#6292=LINE('',#60938,#8789);
#6293=LINE('',#60940,#8790);
#6294=LINE('',#60941,#8791);
#6295=LINE('',#60945,#8792);
#6296=LINE('',#60947,#8793);
#6297=LINE('',#60949,#8794);
#6298=LINE('',#60951,#8795);
#6299=LINE('',#60953,#8796);
#6300=LINE('',#60954,#8797);
#6301=LINE('',#60957,#8798);
#6302=LINE('',#60959,#8799);
#6303=LINE('',#60961,#8800);
#6304=LINE('',#60962,#8801);
#6305=LINE('',#60965,#8802);
#6306=LINE('',#60966,#8803);
#6307=LINE('',#60969,#8804);
#6308=LINE('',#60971,#8805);
#6309=LINE('',#60972,#8806);
#6310=LINE('',#60976,#8807);
#6311=LINE('',#60978,#8808);
#6312=LINE('',#60980,#8809);
#6313=LINE('',#60982,#8810);
#6314=LINE('',#60984,#8811);
#6315=LINE('',#60985,#8812);
#6316=LINE('',#60988,#8813);
#6317=LINE('',#60990,#8814);
#6318=LINE('',#60991,#8815);
#6319=LINE('',#60994,#8816);
#6320=LINE('',#60996,#8817);
#6321=LINE('',#60998,#8818);
#6322=LINE('',#60999,#8819);
#6323=LINE('',#61002,#8820);
#6324=LINE('',#61004,#8821);
#6325=LINE('',#61005,#8822);
#6326=LINE('',#61009,#8823);
#6327=LINE('',#61011,#8824);
#6328=LINE('',#61013,#8825);
#6329=LINE('',#61015,#8826);
#6330=LINE('',#61017,#8827);
#6331=LINE('',#61018,#8828);
#6332=LINE('',#61021,#8829);
#6333=LINE('',#61023,#8830);
#6334=LINE('',#61025,#8831);
#6335=LINE('',#61026,#8832);
#6336=LINE('',#61029,#8833);
#6337=LINE('',#61031,#8834);
#6338=LINE('',#61033,#8835);
#6339=LINE('',#61034,#8836);
#6340=LINE('',#61037,#8837);
#6341=LINE('',#61038,#8838);
#6342=LINE('',#61041,#8839);
#6343=LINE('',#61043,#8840);
#6344=LINE('',#61045,#8841);
#6345=LINE('',#61046,#8842);
#6346=LINE('',#61049,#8843);
#6347=LINE('',#61051,#8844);
#6348=LINE('',#61052,#8845);
#6349=LINE('',#61056,#8846);
#6350=LINE('',#61058,#8847);
#6351=LINE('',#61060,#8848);
#6352=LINE('',#61062,#8849);
#6353=LINE('',#61064,#8850);
#6354=LINE('',#61065,#8851);
#6355=LINE('',#61068,#8852);
#6356=LINE('',#61070,#8853);
#6357=LINE('',#61071,#8854);
#6358=LINE('',#61074,#8855);
#6359=LINE('',#61076,#8856);
#6360=LINE('',#61077,#8857);
#6361=LINE('',#61079,#8858);
#6362=LINE('',#61080,#8859);
#6363=LINE('',#61084,#8860);
#6364=LINE('',#61086,#8861);
#6365=LINE('',#61088,#8862);
#6366=LINE('',#61090,#8863);
#6367=LINE('',#61092,#8864);
#6368=LINE('',#61093,#8865);
#6369=LINE('',#61096,#8866);
#6370=LINE('',#61098,#8867);
#6371=LINE('',#61099,#8868);
#6372=LINE('',#61102,#8869);
#6373=LINE('',#61104,#8870);
#6374=LINE('',#61106,#8871);
#6375=LINE('',#61107,#8872);
#6376=LINE('',#61110,#8873);
#6377=LINE('',#61112,#8874);
#6378=LINE('',#61113,#8875);
#6379=LINE('',#61117,#8876);
#6380=LINE('',#61119,#8877);
#6381=LINE('',#61121,#8878);
#6382=LINE('',#61123,#8879);
#6383=LINE('',#61125,#8880);
#6384=LINE('',#61126,#8881);
#6385=LINE('',#61129,#8882);
#6386=LINE('',#61131,#8883);
#6387=LINE('',#61133,#8884);
#6388=LINE('',#61134,#8885);
#6389=LINE('',#61137,#8886);
#6390=LINE('',#61139,#8887);
#6391=LINE('',#61141,#8888);
#6392=LINE('',#61142,#8889);
#6393=LINE('',#61145,#8890);
#6394=LINE('',#61146,#8891);
#6395=LINE('',#61149,#8892);
#6396=LINE('',#61151,#8893);
#6397=LINE('',#61153,#8894);
#6398=LINE('',#61154,#8895);
#6399=LINE('',#61157,#8896);
#6400=LINE('',#61159,#8897);
#6401=LINE('',#61160,#8898);
#6402=LINE('',#61164,#8899);
#6403=LINE('',#61166,#8900);
#6404=LINE('',#61168,#8901);
#6405=LINE('',#61170,#8902);
#6406=LINE('',#61172,#8903);
#6407=LINE('',#61173,#8904);
#6408=LINE('',#61176,#8905);
#6409=LINE('',#61178,#8906);
#6410=LINE('',#61179,#8907);
#6411=LINE('',#61182,#8908);
#6412=LINE('',#61184,#8909);
#6413=LINE('',#61185,#8910);
#6414=LINE('',#61187,#8911);
#6415=LINE('',#61188,#8912);
#6416=LINE('',#61192,#8913);
#6417=LINE('',#61194,#8914);
#6418=LINE('',#61196,#8915);
#6419=LINE('',#61198,#8916);
#6420=LINE('',#61200,#8917);
#6421=LINE('',#61201,#8918);
#6422=LINE('',#61204,#8919);
#6423=LINE('',#61206,#8920);
#6424=LINE('',#61208,#8921);
#6425=LINE('',#61209,#8922);
#6426=LINE('',#61212,#8923);
#6427=LINE('',#61214,#8924);
#6428=LINE('',#61216,#8925);
#6429=LINE('',#61217,#8926);
#6430=LINE('',#61220,#8927);
#6431=LINE('',#61221,#8928);
#6432=LINE('',#61224,#8929);
#6433=LINE('',#61226,#8930);
#6434=LINE('',#61228,#8931);
#6435=LINE('',#61229,#8932);
#6436=LINE('',#61232,#8933);
#6437=LINE('',#61234,#8934);
#6438=LINE('',#61235,#8935);
#6439=LINE('',#61239,#8936);
#6440=LINE('',#61241,#8937);
#6441=LINE('',#61243,#8938);
#6442=LINE('',#61245,#8939);
#6443=LINE('',#61247,#8940);
#6444=LINE('',#61248,#8941);
#6445=LINE('',#61251,#8942);
#6446=LINE('',#61253,#8943);
#6447=LINE('',#61254,#8944);
#6448=LINE('',#61257,#8945);
#6449=LINE('',#61259,#8946);
#6450=LINE('',#61260,#8947);
#6451=LINE('',#61263,#8948);
#6452=LINE('',#61265,#8949);
#6453=LINE('',#61267,#8950);
#6454=LINE('',#61268,#8951);
#6455=LINE('',#61271,#8952);
#6456=LINE('',#61273,#8953);
#6457=LINE('',#61275,#8954);
#6458=LINE('',#61277,#8955);
#6459=LINE('',#61278,#8956);
#6460=LINE('',#61281,#8957);
#6461=LINE('',#61283,#8958);
#6462=LINE('',#61284,#8959);
#6463=LINE('',#61287,#8960);
#6464=LINE('',#61289,#8961);
#6465=LINE('',#61290,#8962);
#6466=LINE('',#61293,#8963);
#6467=LINE('',#61294,#8964);
#6468=LINE('',#61295,#8965);
#6469=LINE('',#61299,#8966);
#6470=LINE('',#61301,#8967);
#6471=LINE('',#61303,#8968);
#6472=LINE('',#61305,#8969);
#6473=LINE('',#61307,#8970);
#6474=LINE('',#61308,#8971);
#6475=LINE('',#61311,#8972);
#6476=LINE('',#61313,#8973);
#6477=LINE('',#61315,#8974);
#6478=LINE('',#61316,#8975);
#6479=LINE('',#61319,#8976);
#6480=LINE('',#61321,#8977);
#6481=LINE('',#61323,#8978);
#6482=LINE('',#61324,#8979);
#6483=LINE('',#61327,#8980);
#6484=LINE('',#61328,#8981);
#6485=LINE('',#61331,#8982);
#6486=LINE('',#61333,#8983);
#6487=LINE('',#61335,#8984);
#6488=LINE('',#61336,#8985);
#6489=LINE('',#61339,#8986);
#6490=LINE('',#61341,#8987);
#6491=LINE('',#61342,#8988);
#6492=LINE('',#61346,#8989);
#6493=LINE('',#61348,#8990);
#6494=LINE('',#61350,#8991);
#6495=LINE('',#61352,#8992);
#6496=LINE('',#61354,#8993);
#6497=LINE('',#61355,#8994);
#6498=LINE('',#61358,#8995);
#6499=LINE('',#61360,#8996);
#6500=LINE('',#61362,#8997);
#6501=LINE('',#61363,#8998);
#6502=LINE('',#61366,#8999);
#6503=LINE('',#61368,#9000);
#6504=LINE('',#61370,#9001);
#6505=LINE('',#61371,#9002);
#6506=LINE('',#61374,#9003);
#6507=LINE('',#61375,#9004);
#6508=LINE('',#61378,#9005);
#6509=LINE('',#61380,#9006);
#6510=LINE('',#61382,#9007);
#6511=LINE('',#61383,#9008);
#6512=LINE('',#61386,#9009);
#6513=LINE('',#61388,#9010);
#6514=LINE('',#61389,#9011);
#6515=LINE('',#61393,#9012);
#6516=LINE('',#61395,#9013);
#6517=LINE('',#61397,#9014);
#6518=LINE('',#61399,#9015);
#6519=LINE('',#61401,#9016);
#6520=LINE('',#61402,#9017);
#6521=LINE('',#61405,#9018);
#6522=LINE('',#61407,#9019);
#6523=LINE('',#61409,#9020);
#6524=LINE('',#61410,#9021);
#6525=LINE('',#61413,#9022);
#6526=LINE('',#61414,#9023);
#6527=LINE('',#61417,#9024);
#6528=LINE('',#61419,#9025);
#6529=LINE('',#61420,#9026);
#6530=LINE('',#61424,#9027);
#6531=LINE('',#61426,#9028);
#6532=LINE('',#61428,#9029);
#6533=LINE('',#61430,#9030);
#6534=LINE('',#61432,#9031);
#6535=LINE('',#61433,#9032);
#6536=LINE('',#61436,#9033);
#6537=LINE('',#61438,#9034);
#6538=LINE('',#61440,#9035);
#6539=LINE('',#61441,#9036);
#6540=LINE('',#61444,#9037);
#6541=LINE('',#61446,#9038);
#6542=LINE('',#61448,#9039);
#6543=LINE('',#61449,#9040);
#6544=LINE('',#61452,#9041);
#6545=LINE('',#61453,#9042);
#6546=LINE('',#61456,#9043);
#6547=LINE('',#61458,#9044);
#6548=LINE('',#61460,#9045);
#6549=LINE('',#61461,#9046);
#6550=LINE('',#61464,#9047);
#6551=LINE('',#61466,#9048);
#6552=LINE('',#61467,#9049);
#6553=LINE('',#61471,#9050);
#6554=LINE('',#61473,#9051);
#6555=LINE('',#61475,#9052);
#6556=LINE('',#61477,#9053);
#6557=LINE('',#61479,#9054);
#6558=LINE('',#61480,#9055);
#6559=LINE('',#61483,#9056);
#6560=LINE('',#61485,#9057);
#6561=LINE('',#61487,#9058);
#6562=LINE('',#61488,#9059);
#6563=LINE('',#61491,#9060);
#6564=LINE('',#61493,#9061);
#6565=LINE('',#61495,#9062);
#6566=LINE('',#61496,#9063);
#6567=LINE('',#61499,#9064);
#6568=LINE('',#61500,#9065);
#6569=LINE('',#61503,#9066);
#6570=LINE('',#61505,#9067);
#6571=LINE('',#61507,#9068);
#6572=LINE('',#61508,#9069);
#6573=LINE('',#61511,#9070);
#6574=LINE('',#61513,#9071);
#6575=LINE('',#61514,#9072);
#6576=LINE('',#61517,#9073);
#6577=LINE('',#61519,#9074);
#6578=LINE('',#61521,#9075);
#6579=LINE('',#61523,#9076);
#6580=LINE('',#61524,#9077);
#6581=LINE('',#61527,#9078);
#6582=LINE('',#61529,#9079);
#6583=LINE('',#61530,#9080);
#6584=LINE('',#61533,#9081);
#6585=LINE('',#61534,#9082);
#6586=LINE('',#61537,#9083);
#6587=LINE('',#61539,#9084);
#6588=LINE('',#61540,#9085);
#6589=LINE('',#61544,#9086);
#6590=LINE('',#61546,#9087);
#6591=LINE('',#61548,#9088);
#6592=LINE('',#61549,#9089);
#6593=LINE('',#61552,#9090);
#6594=LINE('',#61554,#9091);
#6595=LINE('',#61555,#9092);
#6596=LINE('',#61560,#9093);
#6597=LINE('',#61562,#9094);
#6598=LINE('',#61564,#9095);
#6599=LINE('',#61565,#9096);
#6600=LINE('',#61569,#9097);
#6601=LINE('',#61570,#9098);
#6602=LINE('',#61572,#9099);
#6603=LINE('',#61574,#9100);
#6604=LINE('',#61576,#9101);
#6605=LINE('',#61577,#9102);
#6606=LINE('',#61580,#9103);
#6607=LINE('',#61581,#9104);
#6608=LINE('',#61584,#9105);
#6609=LINE('',#61586,#9106);
#6610=LINE('',#61588,#9107);
#6611=LINE('',#61590,#9108);
#6612=LINE('',#61591,#9109);
#6613=LINE('',#61594,#9110);
#6614=LINE('',#61596,#9111);
#6615=LINE('',#61598,#9112);
#6616=LINE('',#61599,#9113);
#6617=LINE('',#61601,#9114);
#6618=LINE('',#61605,#9115);
#6619=LINE('',#61607,#9116);
#6620=LINE('',#61609,#9117);
#6621=LINE('',#61611,#9118);
#6622=LINE('',#61613,#9119);
#6623=LINE('',#61614,#9120);
#6624=LINE('',#61617,#9121);
#6625=LINE('',#61618,#9122);
#6626=LINE('',#61620,#9123);
#6627=LINE('',#61621,#9124);
#6628=LINE('',#61624,#9125);
#6629=LINE('',#61626,#9126);
#6630=LINE('',#61628,#9127);
#6631=LINE('',#61629,#9128);
#6632=LINE('',#61632,#9129);
#6633=LINE('',#61633,#9130);
#6634=LINE('',#61637,#9131);
#6635=LINE('',#61639,#9132);
#6636=LINE('',#61641,#9133);
#6637=LINE('',#61643,#9134);
#6638=LINE('',#61645,#9135);
#6639=LINE('',#61646,#9136);
#6640=LINE('',#61649,#9137);
#6641=LINE('',#61651,#9138);
#6642=LINE('',#61653,#9139);
#6643=LINE('',#61654,#9140);
#6644=LINE('',#61657,#9141);
#6645=LINE('',#61659,#9142);
#6646=LINE('',#61661,#9143);
#6647=LINE('',#61662,#9144);
#6648=LINE('',#61665,#9145);
#6649=LINE('',#61666,#9146);
#6650=LINE('',#61669,#9147);
#6651=LINE('',#61671,#9148);
#6652=LINE('',#61673,#9149);
#6653=LINE('',#61674,#9150);
#6654=LINE('',#61677,#9151);
#6655=LINE('',#61679,#9152);
#6656=LINE('',#61680,#9153);
#6657=LINE('',#61684,#9154);
#6658=LINE('',#61686,#9155);
#6659=LINE('',#61688,#9156);
#6660=LINE('',#61690,#9157);
#6661=LINE('',#61692,#9158);
#6662=LINE('',#61693,#9159);
#6663=LINE('',#61696,#9160);
#6664=LINE('',#61698,#9161);
#6665=LINE('',#61700,#9162);
#6666=LINE('',#61701,#9163);
#6667=LINE('',#61704,#9164);
#6668=LINE('',#61706,#9165);
#6669=LINE('',#61708,#9166);
#6670=LINE('',#61709,#9167);
#6671=LINE('',#61712,#9168);
#6672=LINE('',#61713,#9169);
#6673=LINE('',#61716,#9170);
#6674=LINE('',#61718,#9171);
#6675=LINE('',#61720,#9172);
#6676=LINE('',#61721,#9173);
#6677=LINE('',#61724,#9174);
#6678=LINE('',#61726,#9175);
#6679=LINE('',#61727,#9176);
#6680=LINE('',#61731,#9177);
#6681=LINE('',#61733,#9178);
#6682=LINE('',#61735,#9179);
#6683=LINE('',#61737,#9180);
#6684=LINE('',#61739,#9181);
#6685=LINE('',#61740,#9182);
#6686=LINE('',#61743,#9183);
#6687=LINE('',#61745,#9184);
#6688=LINE('',#61747,#9185);
#6689=LINE('',#61748,#9186);
#6690=LINE('',#61751,#9187);
#6691=LINE('',#61753,#9188);
#6692=LINE('',#61755,#9189);
#6693=LINE('',#61756,#9190);
#6694=LINE('',#61759,#9191);
#6695=LINE('',#61760,#9192);
#6696=LINE('',#61763,#9193);
#6697=LINE('',#61765,#9194);
#6698=LINE('',#61767,#9195);
#6699=LINE('',#61768,#9196);
#6700=LINE('',#61771,#9197);
#6701=LINE('',#61773,#9198);
#6702=LINE('',#61774,#9199);
#6703=LINE('',#61778,#9200);
#6704=LINE('',#61780,#9201);
#6705=LINE('',#61782,#9202);
#6706=LINE('',#61784,#9203);
#6707=LINE('',#61786,#9204);
#6708=LINE('',#61787,#9205);
#6709=LINE('',#61790,#9206);
#6710=LINE('',#61792,#9207);
#6711=LINE('',#61794,#9208);
#6712=LINE('',#61795,#9209);
#6713=LINE('',#61798,#9210);
#6714=LINE('',#61800,#9211);
#6715=LINE('',#61802,#9212);
#6716=LINE('',#61803,#9213);
#6717=LINE('',#61806,#9214);
#6718=LINE('',#61807,#9215);
#6719=LINE('',#61810,#9216);
#6720=LINE('',#61812,#9217);
#6721=LINE('',#61814,#9218);
#6722=LINE('',#61815,#9219);
#6723=LINE('',#61818,#9220);
#6724=LINE('',#61820,#9221);
#6725=LINE('',#61821,#9222);
#6726=LINE('',#61825,#9223);
#6727=LINE('',#61827,#9224);
#6728=LINE('',#61829,#9225);
#6729=LINE('',#61831,#9226);
#6730=LINE('',#61833,#9227);
#6731=LINE('',#61834,#9228);
#6732=LINE('',#61837,#9229);
#6733=LINE('',#61839,#9230);
#6734=LINE('',#61840,#9231);
#6735=LINE('',#61843,#9232);
#6736=LINE('',#61845,#9233);
#6737=LINE('',#61846,#9234);
#6738=LINE('',#61848,#9235);
#6739=LINE('',#61849,#9236);
#6740=LINE('',#61851,#9237);
#6741=LINE('',#61852,#9238);
#6742=LINE('',#61855,#9239);
#6743=LINE('',#61856,#9240);
#6744=LINE('',#61858,#9241);
#6745=LINE('',#61860,#9242);
#6746=LINE('',#61861,#9243);
#6747=LINE('',#61864,#9244);
#6748=LINE('',#61865,#9245);
#6749=LINE('',#61868,#9246);
#6750=LINE('',#61869,#9247);
#6751=LINE('',#61871,#9248);
#6752=LINE('',#61873,#9249);
#6753=LINE('',#61874,#9250);
#6754=LINE('',#61877,#9251);
#6755=LINE('',#61878,#9252);
#6756=LINE('',#61880,#9253);
#6757=LINE('',#61883,#9254);
#6758=LINE('',#61885,#9255);
#6759=LINE('',#61887,#9256);
#6760=LINE('',#61889,#9257);
#6761=LINE('',#61891,#9258);
#6762=LINE('',#61893,#9259);
#6763=LINE('',#61895,#9260);
#6764=LINE('',#61897,#9261);
#6765=LINE('',#61899,#9262);
#6766=LINE('',#61901,#9263);
#6767=LINE('',#61903,#9264);
#6768=LINE('',#61905,#9265);
#6769=LINE('',#61907,#9266);
#6770=LINE('',#61909,#9267);
#6771=LINE('',#61911,#9268);
#6772=LINE('',#61913,#9269);
#6773=LINE('',#61915,#9270);
#6774=LINE('',#61917,#9271);
#6775=LINE('',#61919,#9272);
#6776=LINE('',#61921,#9273);
#6777=LINE('',#61923,#9274);
#6778=LINE('',#61925,#9275);
#6779=LINE('',#61927,#9276);
#6780=LINE('',#61929,#9277);
#6781=LINE('',#61931,#9278);
#6782=LINE('',#61933,#9279);
#6783=LINE('',#61935,#9280);
#6784=LINE('',#61936,#9281);
#6785=LINE('',#61937,#9282);
#6786=LINE('',#61938,#9283);
#6787=LINE('',#61940,#9284);
#6788=LINE('',#61942,#9285);
#6789=LINE('',#61944,#9286);
#6790=LINE('',#61946,#9287);
#6791=LINE('',#61948,#9288);
#6792=LINE('',#61950,#9289);
#6793=LINE('',#61952,#9290);
#6794=LINE('',#61954,#9291);
#6795=LINE('',#61956,#9292);
#6796=LINE('',#61958,#9293);
#6797=LINE('',#61960,#9294);
#6798=LINE('',#61962,#9295);
#6799=LINE('',#61964,#9296);
#6800=LINE('',#61966,#9297);
#6801=LINE('',#61968,#9298);
#6802=LINE('',#61970,#9299);
#6803=LINE('',#61972,#9300);
#6804=LINE('',#61974,#9301);
#6805=LINE('',#61976,#9302);
#6806=LINE('',#61978,#9303);
#6807=LINE('',#61980,#9304);
#6808=LINE('',#61982,#9305);
#6809=LINE('',#61984,#9306);
#6810=LINE('',#61986,#9307);
#6811=LINE('',#61988,#9308);
#6812=LINE('',#61989,#9309);
#6813=LINE('',#61990,#9310);
#6814=LINE('',#61991,#9311);
#6815=LINE('',#61992,#9312);
#6816=LINE('',#61993,#9313);
#6817=LINE('',#61995,#9314);
#6818=LINE('',#61996,#9315);
#6819=LINE('',#61997,#9316);
#6820=LINE('',#61998,#9317);
#6821=LINE('',#61999,#9318);
#6822=LINE('',#62001,#9319);
#6823=LINE('',#62003,#9320);
#6824=LINE('',#62005,#9321);
#6825=LINE('',#62007,#9322);
#6826=LINE('',#62009,#9323);
#6827=LINE('',#62010,#9324);
#6828=LINE('',#62011,#9325);
#6829=LINE('',#62012,#9326);
#6830=LINE('',#62013,#9327);
#6831=LINE('',#62014,#9328);
#6832=LINE('',#62016,#9329);
#6833=LINE('',#62019,#9330);
#6834=LINE('',#62020,#9331);
#6835=LINE('',#62022,#9332);
#6836=LINE('',#62024,#9333);
#6837=LINE('',#62027,#9334);
#6838=LINE('',#62028,#9335);
#6839=LINE('',#62031,#9336);
#6840=LINE('',#62032,#9337);
#6841=LINE('',#62034,#9338);
#6842=LINE('',#62036,#9339);
#6843=LINE('',#62039,#9340);
#6844=LINE('',#62040,#9341);
#6845=LINE('',#62043,#9342);
#6846=LINE('',#62044,#9343);
#6847=LINE('',#62046,#9344);
#6848=LINE('',#62048,#9345);
#6849=LINE('',#62051,#9346);
#6850=LINE('',#62052,#9347);
#6851=LINE('',#62055,#9348);
#6852=LINE('',#62056,#9349);
#6853=LINE('',#62058,#9350);
#6854=LINE('',#62061,#9351);
#6855=LINE('',#62062,#9352);
#6856=LINE('',#62065,#9353);
#6857=LINE('',#62066,#9354);
#6858=LINE('',#62069,#9355);
#6859=LINE('',#62070,#9356);
#6860=LINE('',#62074,#9357);
#6861=LINE('',#62076,#9358);
#6862=LINE('',#62078,#9359);
#6863=LINE('',#62079,#9360);
#6864=LINE('',#62082,#9361);
#6865=LINE('',#62083,#9362);
#6866=LINE('',#62085,#9363);
#6867=LINE('',#62086,#9364);
#6868=LINE('',#62088,#9365);
#6869=LINE('',#62089,#9366);
#6870=LINE('',#62092,#9367);
#6871=LINE('',#62094,#9368);
#6872=LINE('',#62095,#9369);
#6873=LINE('',#62098,#9370);
#6874=LINE('',#62100,#9371);
#6875=LINE('',#62101,#9372);
#6876=LINE('',#62104,#9373);
#6877=LINE('',#62105,#9374);
#6878=LINE('',#62106,#9375);
#6879=LINE('',#62109,#9376);
#6880=LINE('',#62111,#9377);
#6881=LINE('',#62113,#9378);
#6882=LINE('',#62114,#9379);
#6883=LINE('',#62117,#9380);
#6884=LINE('',#62118,#9381);
#6885=LINE('',#62122,#9382);
#6886=LINE('',#62124,#9383);
#6887=LINE('',#62126,#9384);
#6888=LINE('',#62128,#9385);
#6889=LINE('',#62130,#9386);
#6890=LINE('',#62131,#9387);
#6891=LINE('',#62133,#9388);
#6892=LINE('',#62135,#9389);
#6893=LINE('',#62136,#9390);
#6894=LINE('',#62139,#9391);
#6895=LINE('',#62141,#9392);
#6896=LINE('',#62142,#9393);
#6897=LINE('',#62145,#9394);
#6898=LINE('',#62146,#9395);
#6899=LINE('',#62149,#9396);
#6900=LINE('',#62151,#9397);
#6901=LINE('',#62153,#9398);
#6902=LINE('',#62154,#9399);
#6903=LINE('',#62156,#9400);
#6904=LINE('',#62158,#9401);
#6905=LINE('',#62160,#9402);
#6906=LINE('',#62163,#9403);
#6907=LINE('',#62164,#9404);
#6908=LINE('',#62167,#9405);
#6909=LINE('',#62168,#9406);
#6910=LINE('',#62170,#9407);
#6911=LINE('',#62172,#9408);
#6912=LINE('',#62175,#9409);
#6913=LINE('',#62176,#9410);
#6914=LINE('',#62178,#9411);
#6915=LINE('',#62180,#9412);
#6916=LINE('',#62183,#9413);
#6917=LINE('',#62184,#9414);
#6918=LINE('',#62187,#9415);
#6919=LINE('',#62188,#9416);
#6920=LINE('',#62190,#9417);
#6921=LINE('',#62192,#9418);
#6922=LINE('',#62194,#9419);
#6923=LINE('',#62197,#9420);
#6924=LINE('',#62198,#9421);
#6925=LINE('',#62200,#9422);
#6926=LINE('',#62202,#9423);
#6927=LINE('',#62205,#9424);
#6928=LINE('',#62206,#9425);
#6929=LINE('',#62208,#9426);
#6930=LINE('',#62210,#9427);
#6931=LINE('',#62213,#9428);
#6932=LINE('',#62214,#9429);
#6933=LINE('',#62216,#9430);
#6934=LINE('',#62218,#9431);
#6935=LINE('',#62221,#9432);
#6936=LINE('',#62222,#9433);
#6937=LINE('',#62224,#9434);
#6938=LINE('',#62226,#9435);
#6939=LINE('',#62229,#9436);
#6940=LINE('',#62230,#9437);
#6941=LINE('',#62233,#9438);
#6942=LINE('',#62234,#9439);
#6943=LINE('',#62236,#9440);
#6944=LINE('',#62240,#9441);
#6945=LINE('',#62242,#9442);
#6946=LINE('',#62244,#9443);
#6947=LINE('',#62246,#9444);
#6948=LINE('',#62248,#9445);
#6949=LINE('',#62249,#9446);
#6950=LINE('',#62251,#9447);
#6951=LINE('',#62253,#9448);
#6952=LINE('',#62254,#9449);
#6953=LINE('',#62257,#9450);
#6954=LINE('',#62259,#9451);
#6955=LINE('',#62260,#9452);
#6956=LINE('',#62263,#9453);
#6957=LINE('',#62264,#9454);
#6958=LINE('',#62267,#9455);
#6959=LINE('',#62269,#9456);
#6960=LINE('',#62271,#9457);
#6961=LINE('',#62272,#9458);
#6962=LINE('',#62275,#9459);
#6963=LINE('',#62276,#9460);
#6964=LINE('',#62280,#9461);
#6965=LINE('',#62282,#9462);
#6966=LINE('',#62284,#9463);
#6967=LINE('',#62286,#9464);
#6968=LINE('',#62288,#9465);
#6969=LINE('',#62289,#9466);
#6970=LINE('',#62291,#9467);
#6971=LINE('',#62293,#9468);
#6972=LINE('',#62294,#9469);
#6973=LINE('',#62297,#9470);
#6974=LINE('',#62299,#9471);
#6975=LINE('',#62300,#9472);
#6976=LINE('',#62303,#9473);
#6977=LINE('',#62304,#9474);
#6978=LINE('',#62307,#9475);
#6979=LINE('',#62309,#9476);
#6980=LINE('',#62311,#9477);
#6981=LINE('',#62312,#9478);
#6982=LINE('',#62315,#9479);
#6983=LINE('',#62316,#9480);
#6984=LINE('',#62320,#9481);
#6985=LINE('',#62322,#9482);
#6986=LINE('',#62324,#9483);
#6987=LINE('',#62326,#9484);
#6988=LINE('',#62328,#9485);
#6989=LINE('',#62329,#9486);
#6990=LINE('',#62331,#9487);
#6991=LINE('',#62333,#9488);
#6992=LINE('',#62334,#9489);
#6993=LINE('',#62337,#9490);
#6994=LINE('',#62339,#9491);
#6995=LINE('',#62340,#9492);
#6996=LINE('',#62343,#9493);
#6997=LINE('',#62344,#9494);
#6998=LINE('',#62347,#9495);
#6999=LINE('',#62349,#9496);
#7000=LINE('',#62351,#9497);
#7001=LINE('',#62352,#9498);
#7002=LINE('',#62355,#9499);
#7003=LINE('',#62356,#9500);
#7004=LINE('',#62360,#9501);
#7005=LINE('',#62362,#9502);
#7006=LINE('',#62364,#9503);
#7007=LINE('',#62366,#9504);
#7008=LINE('',#62368,#9505);
#7009=LINE('',#62369,#9506);
#7010=LINE('',#62372,#9507);
#7011=LINE('',#62374,#9508);
#7012=LINE('',#62375,#9509);
#7013=LINE('',#62377,#9510);
#7014=LINE('',#62378,#9511);
#7015=LINE('',#62381,#9512);
#7016=LINE('',#62383,#9513);
#7017=LINE('',#62384,#9514);
#7018=LINE('',#62387,#9515);
#7019=LINE('',#62389,#9516);
#7020=LINE('',#62391,#9517);
#7021=LINE('',#62393,#9518);
#7022=LINE('',#62394,#9519);
#7023=LINE('',#62397,#9520);
#7024=LINE('',#62399,#9521);
#7025=LINE('',#62400,#9522);
#7026=LINE('',#62403,#9523);
#7027=LINE('',#62405,#9524);
#7028=LINE('',#62406,#9525);
#7029=LINE('',#62409,#9526);
#7030=LINE('',#62410,#9527);
#7031=LINE('',#62411,#9528);
#7032=LINE('',#62415,#9529);
#7033=LINE('',#62417,#9530);
#7034=LINE('',#62419,#9531);
#7035=LINE('',#62421,#9532);
#7036=LINE('',#62423,#9533);
#7037=LINE('',#62424,#9534);
#7038=LINE('',#62426,#9535);
#7039=LINE('',#62428,#9536);
#7040=LINE('',#62429,#9537);
#7041=LINE('',#62432,#9538);
#7042=LINE('',#62434,#9539);
#7043=LINE('',#62435,#9540);
#7044=LINE('',#62438,#9541);
#7045=LINE('',#62439,#9542);
#7046=LINE('',#62442,#9543);
#7047=LINE('',#62444,#9544);
#7048=LINE('',#62446,#9545);
#7049=LINE('',#62447,#9546);
#7050=LINE('',#62450,#9547);
#7051=LINE('',#62451,#9548);
#7052=LINE('',#62455,#9549);
#7053=LINE('',#62457,#9550);
#7054=LINE('',#62459,#9551);
#7055=LINE('',#62461,#9552);
#7056=LINE('',#62463,#9553);
#7057=LINE('',#62464,#9554);
#7058=LINE('',#62466,#9555);
#7059=LINE('',#62468,#9556);
#7060=LINE('',#62469,#9557);
#7061=LINE('',#62472,#9558);
#7062=LINE('',#62474,#9559);
#7063=LINE('',#62475,#9560);
#7064=LINE('',#62478,#9561);
#7065=LINE('',#62479,#9562);
#7066=LINE('',#62482,#9563);
#7067=LINE('',#62484,#9564);
#7068=LINE('',#62486,#9565);
#7069=LINE('',#62487,#9566);
#7070=LINE('',#62490,#9567);
#7071=LINE('',#62491,#9568);
#7072=LINE('',#62494,#9569);
#7073=LINE('',#62496,#9570);
#7074=LINE('',#62498,#9571);
#7075=LINE('',#62499,#9572);
#7076=LINE('',#62502,#9573);
#7077=LINE('',#62504,#9574);
#7078=LINE('',#62506,#9575);
#7079=LINE('',#62507,#9576);
#7080=LINE('',#62510,#9577);
#7081=LINE('',#62511,#9578);
#7082=LINE('',#62513,#9579);
#7083=LINE('',#62515,#9580);
#7084=LINE('',#62518,#9581);
#7085=LINE('',#62519,#9582);
#7086=LINE('',#62521,#9583);
#7087=LINE('',#62523,#9584);
#7088=LINE('',#62526,#9585);
#7089=LINE('',#62527,#9586);
#7090=LINE('',#62530,#9587);
#7091=LINE('',#62531,#9588);
#7092=LINE('',#62533,#9589);
#7093=LINE('',#62535,#9590);
#7094=LINE('',#62537,#9591);
#7095=LINE('',#62540,#9592);
#7096=LINE('',#62541,#9593);
#7097=LINE('',#62543,#9594);
#7098=LINE('',#62545,#9595);
#7099=LINE('',#62548,#9596);
#7100=LINE('',#62549,#9597);
#7101=LINE('',#62551,#9598);
#7102=LINE('',#62553,#9599);
#7103=LINE('',#62556,#9600);
#7104=LINE('',#62557,#9601);
#7105=LINE('',#62560,#9602);
#7106=LINE('',#62561,#9603);
#7107=LINE('',#62563,#9604);
#7108=LINE('',#62565,#9605);
#7109=LINE('',#62568,#9606);
#7110=LINE('',#62569,#9607);
#7111=LINE('',#62572,#9608);
#7112=LINE('',#62573,#9609);
#7113=LINE('',#62575,#9610);
#7114=LINE('',#62577,#9611);
#7115=LINE('',#62580,#9612);
#7116=LINE('',#62581,#9613);
#7117=LINE('',#62583,#9614);
#7118=LINE('',#62585,#9615);
#7119=LINE('',#62588,#9616);
#7120=LINE('',#62589,#9617);
#7121=LINE('',#62591,#9618);
#7122=LINE('',#62593,#9619);
#7123=LINE('',#62596,#9620);
#7124=LINE('',#62597,#9621);
#7125=LINE('',#62600,#9622);
#7126=LINE('',#62601,#9623);
#7127=LINE('',#62603,#9624);
#7128=LINE('',#62607,#9625);
#7129=LINE('',#62609,#9626);
#7130=LINE('',#62611,#9627);
#7131=LINE('',#62613,#9628);
#7132=LINE('',#62615,#9629);
#7133=LINE('',#62616,#9630);
#7134=LINE('',#62618,#9631);
#7135=LINE('',#62620,#9632);
#7136=LINE('',#62621,#9633);
#7137=LINE('',#62624,#9634);
#7138=LINE('',#62626,#9635);
#7139=LINE('',#62627,#9636);
#7140=LINE('',#62630,#9637);
#7141=LINE('',#62631,#9638);
#7142=LINE('',#62634,#9639);
#7143=LINE('',#62636,#9640);
#7144=LINE('',#62638,#9641);
#7145=LINE('',#62639,#9642);
#7146=LINE('',#62642,#9643);
#7147=LINE('',#62643,#9644);
#7148=LINE('',#62647,#9645);
#7149=LINE('',#62649,#9646);
#7150=LINE('',#62651,#9647);
#7151=LINE('',#62653,#9648);
#7152=LINE('',#62655,#9649);
#7153=LINE('',#62656,#9650);
#7154=LINE('',#62658,#9651);
#7155=LINE('',#62660,#9652);
#7156=LINE('',#62661,#9653);
#7157=LINE('',#62664,#9654);
#7158=LINE('',#62666,#9655);
#7159=LINE('',#62667,#9656);
#7160=LINE('',#62670,#9657);
#7161=LINE('',#62671,#9658);
#7162=LINE('',#62674,#9659);
#7163=LINE('',#62676,#9660);
#7164=LINE('',#62678,#9661);
#7165=LINE('',#62679,#9662);
#7166=LINE('',#62682,#9663);
#7167=LINE('',#62683,#9664);
#7168=LINE('',#62687,#9665);
#7169=LINE('',#62689,#9666);
#7170=LINE('',#62691,#9667);
#7171=LINE('',#62693,#9668);
#7172=LINE('',#62695,#9669);
#7173=LINE('',#62696,#9670);
#7174=LINE('',#62698,#9671);
#7175=LINE('',#62700,#9672);
#7176=LINE('',#62701,#9673);
#7177=LINE('',#62704,#9674);
#7178=LINE('',#62706,#9675);
#7179=LINE('',#62707,#9676);
#7180=LINE('',#62710,#9677);
#7181=LINE('',#62711,#9678);
#7182=LINE('',#62714,#9679);
#7183=LINE('',#62716,#9680);
#7184=LINE('',#62718,#9681);
#7185=LINE('',#62719,#9682);
#7186=LINE('',#62722,#9683);
#7187=LINE('',#62723,#9684);
#7188=LINE('',#62727,#9685);
#7189=LINE('',#62729,#9686);
#7190=LINE('',#62731,#9687);
#7191=LINE('',#62733,#9688);
#7192=LINE('',#62735,#9689);
#7193=LINE('',#62736,#9690);
#7194=LINE('',#62738,#9691);
#7195=LINE('',#62740,#9692);
#7196=LINE('',#62741,#9693);
#7197=LINE('',#62744,#9694);
#7198=LINE('',#62746,#9695);
#7199=LINE('',#62747,#9696);
#7200=LINE('',#62750,#9697);
#7201=LINE('',#62751,#9698);
#7202=LINE('',#62754,#9699);
#7203=LINE('',#62756,#9700);
#7204=LINE('',#62758,#9701);
#7205=LINE('',#62759,#9702);
#7206=LINE('',#62762,#9703);
#7207=LINE('',#62763,#9704);
#7208=LINE('',#62767,#9705);
#7209=LINE('',#62769,#9706);
#7210=LINE('',#62771,#9707);
#7211=LINE('',#62773,#9708);
#7212=LINE('',#62775,#9709);
#7213=LINE('',#62776,#9710);
#7214=LINE('',#62778,#9711);
#7215=LINE('',#62780,#9712);
#7216=LINE('',#62781,#9713);
#7217=LINE('',#62784,#9714);
#7218=LINE('',#62786,#9715);
#7219=LINE('',#62787,#9716);
#7220=LINE('',#62790,#9717);
#7221=LINE('',#62791,#9718);
#7222=LINE('',#62794,#9719);
#7223=LINE('',#62796,#9720);
#7224=LINE('',#62798,#9721);
#7225=LINE('',#62799,#9722);
#7226=LINE('',#62802,#9723);
#7227=LINE('',#62803,#9724);
#7228=LINE('',#62807,#9725);
#7229=LINE('',#62809,#9726);
#7230=LINE('',#62811,#9727);
#7231=LINE('',#62813,#9728);
#7232=LINE('',#62815,#9729);
#7233=LINE('',#62816,#9730);
#7234=LINE('',#62818,#9731);
#7235=LINE('',#62820,#9732);
#7236=LINE('',#62821,#9733);
#7237=LINE('',#62824,#9734);
#7238=LINE('',#62826,#9735);
#7239=LINE('',#62827,#9736);
#7240=LINE('',#62830,#9737);
#7241=LINE('',#62831,#9738);
#7242=LINE('',#62834,#9739);
#7243=LINE('',#62836,#9740);
#7244=LINE('',#62838,#9741);
#7245=LINE('',#62839,#9742);
#7246=LINE('',#62842,#9743);
#7247=LINE('',#62843,#9744);
#7248=LINE('',#62846,#9745);
#7249=LINE('',#62848,#9746);
#7250=LINE('',#62850,#9747);
#7251=LINE('',#62851,#9748);
#7252=LINE('',#62854,#9749);
#7253=LINE('',#62856,#9750);
#7254=LINE('',#62858,#9751);
#7255=LINE('',#62859,#9752);
#7256=LINE('',#62862,#9753);
#7257=LINE('',#62863,#9754);
#7258=LINE('',#62865,#9755);
#7259=LINE('',#62867,#9756);
#7260=LINE('',#62870,#9757);
#7261=LINE('',#62871,#9758);
#7262=LINE('',#62873,#9759);
#7263=LINE('',#62875,#9760);
#7264=LINE('',#62878,#9761);
#7265=LINE('',#62879,#9762);
#7266=LINE('',#62882,#9763);
#7267=LINE('',#62883,#9764);
#7268=LINE('',#62885,#9765);
#7269=LINE('',#62887,#9766);
#7270=LINE('',#62890,#9767);
#7271=LINE('',#62891,#9768);
#7272=LINE('',#62894,#9769);
#7273=LINE('',#62895,#9770);
#7274=LINE('',#62897,#9771);
#7275=LINE('',#62899,#9772);
#7276=LINE('',#62902,#9773);
#7277=LINE('',#62903,#9774);
#7278=LINE('',#62906,#9775);
#7279=LINE('',#62907,#9776);
#7280=LINE('',#62909,#9777);
#7281=LINE('',#62911,#9778);
#7282=LINE('',#62914,#9779);
#7283=LINE('',#62915,#9780);
#7284=LINE('',#62918,#9781);
#7285=LINE('',#62919,#9782);
#7286=LINE('',#62921,#9783);
#7287=LINE('',#62923,#9784);
#7288=LINE('',#62926,#9785);
#7289=LINE('',#62927,#9786);
#7290=LINE('',#62930,#9787);
#7291=LINE('',#62931,#9788);
#7292=LINE('',#62933,#9789);
#7293=LINE('',#62935,#9790);
#7294=LINE('',#62936,#9791);
#7295=LINE('',#62939,#9792);
#7296=LINE('',#62940,#9793);
#7297=LINE('',#62942,#9794);
#7298=LINE('',#62944,#9795);
#7299=LINE('',#62947,#9796);
#7300=LINE('',#62949,#9797);
#7301=LINE('',#62950,#9798);
#7302=LINE('',#62953,#9799);
#7303=LINE('',#62954,#9800);
#7304=LINE('',#62957,#9801);
#7305=LINE('',#62958,#9802);
#7306=LINE('',#62961,#9803);
#7307=LINE('',#62963,#9804);
#7308=LINE('',#62965,#9805);
#7309=LINE('',#62967,#9806);
#7310=LINE('',#62969,#9807);
#7311=LINE('',#62971,#9808);
#7312=LINE('',#62973,#9809);
#7313=LINE('',#62975,#9810);
#7314=LINE('',#62976,#9811);
#7315=LINE('',#62978,#9812);
#7316=LINE('',#62979,#9813);
#7317=LINE('',#62981,#9814);
#7318=LINE('',#62983,#9815);
#7319=LINE('',#62985,#9816);
#7320=LINE('',#62987,#9817);
#7321=LINE('',#62989,#9818);
#7322=LINE('',#62991,#9819);
#7323=LINE('',#62993,#9820);
#7324=LINE('',#62995,#9821);
#7325=LINE('',#62996,#9822);
#7326=LINE('',#62998,#9823);
#7327=LINE('',#63000,#9824);
#7328=LINE('',#63002,#9825);
#7329=LINE('',#63004,#9826);
#7330=LINE('',#63006,#9827);
#7331=LINE('',#63007,#9828);
#7332=LINE('',#63009,#9829);
#7333=LINE('',#63011,#9830);
#7334=LINE('',#63013,#9831);
#7335=LINE('',#63015,#9832);
#7336=LINE('',#63017,#9833);
#7337=LINE('',#63019,#9834);
#7338=LINE('',#63021,#9835);
#7339=LINE('',#63023,#9836);
#7340=LINE('',#63024,#9837);
#7341=LINE('',#63026,#9838);
#7342=LINE('',#63028,#9839);
#7343=LINE('',#63030,#9840);
#7344=LINE('',#63032,#9841);
#7345=LINE('',#63034,#9842);
#7346=LINE('',#63036,#9843);
#7347=LINE('',#63038,#9844);
#7348=LINE('',#63040,#9845);
#7349=LINE('',#63041,#9846);
#7350=LINE('',#63043,#9847);
#7351=LINE('',#63045,#9848);
#7352=LINE('',#63047,#9849);
#7353=LINE('',#63049,#9850);
#7354=LINE('',#63051,#9851);
#7355=LINE('',#63053,#9852);
#7356=LINE('',#63055,#9853);
#7357=LINE('',#63057,#9854);
#7358=LINE('',#63059,#9855);
#7359=LINE('',#63061,#9856);
#7360=LINE('',#63063,#9857);
#7361=LINE('',#63065,#9858);
#7362=LINE('',#63067,#9859);
#7363=LINE('',#63068,#9860);
#7364=LINE('',#63070,#9861);
#7365=LINE('',#63072,#9862);
#7366=LINE('',#63074,#9863);
#7367=LINE('',#63076,#9864);
#7368=LINE('',#63078,#9865);
#7369=LINE('',#63080,#9866);
#7370=LINE('',#63082,#9867);
#7371=LINE('',#63084,#9868);
#7372=LINE('',#63085,#9869);
#7373=LINE('',#63087,#9870);
#7374=LINE('',#63089,#9871);
#7375=LINE('',#63091,#9872);
#7376=LINE('',#63093,#9873);
#7377=LINE('',#63095,#9874);
#7378=LINE('',#63097,#9875);
#7379=LINE('',#63099,#9876);
#7380=LINE('',#63101,#9877);
#7381=LINE('',#63103,#9878);
#7382=LINE('',#63105,#9879);
#7383=LINE('',#63107,#9880);
#7384=LINE('',#63109,#9881);
#7385=LINE('',#63111,#9882);
#7386=LINE('',#63113,#9883);
#7387=LINE('',#63115,#9884);
#7388=LINE('',#63117,#9885);
#7389=LINE('',#63119,#9886);
#7390=LINE('',#63121,#9887);
#7391=LINE('',#63123,#9888);
#7392=LINE('',#63125,#9889);
#7393=LINE('',#63127,#9890);
#7394=LINE('',#63129,#9891);
#7395=LINE('',#63131,#9892);
#7396=LINE('',#63133,#9893);
#7397=LINE('',#63134,#9894);
#7398=LINE('',#63136,#9895);
#7399=LINE('',#63138,#9896);
#7400=LINE('',#63140,#9897);
#7401=LINE('',#63142,#9898);
#7402=LINE('',#63144,#9899);
#7403=LINE('',#63146,#9900);
#7404=LINE('',#63148,#9901);
#7405=LINE('',#63150,#9902);
#7406=LINE('',#63151,#9903);
#7407=LINE('',#63153,#9904);
#7408=LINE('',#63155,#9905);
#7409=LINE('',#63157,#9906);
#7410=LINE('',#63159,#9907);
#7411=LINE('',#63161,#9908);
#7412=LINE('',#63163,#9909);
#7413=LINE('',#63165,#9910);
#7414=LINE('',#63167,#9911);
#7415=LINE('',#63169,#9912);
#7416=LINE('',#63171,#9913);
#7417=LINE('',#63173,#9914);
#7418=LINE('',#63175,#9915);
#7419=LINE('',#63176,#9916);
#7420=LINE('',#63180,#9917);
#7421=LINE('',#63182,#9918);
#7422=LINE('',#63183,#9919);
#7423=LINE('',#63185,#9920);
#7424=LINE('',#63187,#9921);
#7425=LINE('',#63190,#9922);
#7426=LINE('',#63191,#9923);
#7427=LINE('',#63193,#9924);
#7428=LINE('',#63195,#9925);
#7429=LINE('',#63198,#9926);
#7430=LINE('',#63199,#9927);
#7431=LINE('',#63201,#9928);
#7432=LINE('',#63203,#9929);
#7433=LINE('',#63206,#9930);
#7434=LINE('',#63208,#9931);
#7435=LINE('',#63210,#9932);
#7436=LINE('',#63212,#9933);
#7437=LINE('',#63213,#9934);
#7438=LINE('',#63215,#9935);
#7439=LINE('',#63217,#9936);
#7440=LINE('',#63220,#9937);
#7441=LINE('',#63221,#9938);
#7442=LINE('',#63224,#9939);
#7443=LINE('',#63226,#9940);
#7444=LINE('',#63228,#9941);
#7445=LINE('',#63229,#9942);
#7446=LINE('',#63231,#9943);
#7447=LINE('',#63233,#9944);
#7448=LINE('',#63236,#9945);
#7449=LINE('',#63237,#9946);
#7450=LINE('',#63239,#9947);
#7451=LINE('',#63241,#9948);
#7452=LINE('',#63244,#9949);
#7453=LINE('',#63245,#9950);
#7454=LINE('',#63247,#9951);
#7455=LINE('',#63249,#9952);
#7456=LINE('',#63252,#9953);
#7457=LINE('',#63253,#9954);
#7458=LINE('',#63255,#9955);
#7459=LINE('',#63257,#9956);
#7460=LINE('',#63260,#9957);
#7461=LINE('',#63261,#9958);
#7462=LINE('',#63263,#9959);
#7463=LINE('',#63265,#9960);
#7464=LINE('',#63268,#9961);
#7465=LINE('',#63269,#9962);
#7466=LINE('',#63273,#9963);
#7467=LINE('',#63274,#9964);
#7468=LINE('',#63276,#9965);
#7469=LINE('',#63278,#9966);
#7470=LINE('',#63281,#9967);
#7471=LINE('',#63282,#9968);
#7472=LINE('',#63284,#9969);
#7473=LINE('',#63286,#9970);
#7474=LINE('',#63289,#9971);
#7475=LINE('',#63291,#9972);
#7476=LINE('',#63293,#9973);
#7477=LINE('',#63295,#9974);
#7478=LINE('',#63296,#9975);
#7479=LINE('',#63298,#9976);
#7480=LINE('',#63300,#9977);
#7481=LINE('',#63303,#9978);
#7482=LINE('',#63304,#9979);
#7483=LINE('',#63306,#9980);
#7484=LINE('',#63308,#9981);
#7485=LINE('',#63311,#9982);
#7486=LINE('',#63312,#9983);
#7487=LINE('',#63314,#9984);
#7488=LINE('',#63317,#9985);
#7489=LINE('',#63319,#9986);
#7490=LINE('',#63321,#9987);
#7491=LINE('',#63322,#9988);
#7492=LINE('',#63324,#9989);
#7493=LINE('',#63326,#9990);
#7494=LINE('',#63329,#9991);
#7495=LINE('',#63330,#9992);
#7496=LINE('',#63334,#9993);
#7497=LINE('',#63335,#9994);
#7498=LINE('',#63337,#9995);
#7499=LINE('',#63339,#9996);
#7500=LINE('',#63342,#9997);
#7501=LINE('',#63343,#9998);
#7502=LINE('',#63345,#9999);
#7503=LINE('',#63347,#10000);
#7504=LINE('',#63350,#10001);
#7505=LINE('',#63352,#10002);
#7506=LINE('',#63354,#10003);
#7507=LINE('',#63356,#10004);
#7508=LINE('',#63357,#10005);
#7509=LINE('',#63359,#10006);
#7510=LINE('',#63362,#10007);
#7511=LINE('',#63364,#10008);
#7512=LINE('',#63366,#10009);
#7513=LINE('',#63367,#10010);
#7514=LINE('',#63369,#10011);
#7515=LINE('',#63371,#10012);
#7516=LINE('',#63374,#10013);
#7517=LINE('',#63375,#10014);
#7518=LINE('',#63380,#10015);
#7519=LINE('',#63381,#10016);
#7520=LINE('',#63383,#10017);
#7521=LINE('',#63384,#10018);
#7522=LINE('',#63386,#10019);
#7523=LINE('',#63388,#10020);
#7524=LINE('',#63391,#10021);
#7525=LINE('',#63392,#10022);
#7526=LINE('',#63394,#10023);
#7527=LINE('',#63559,#10024);
#7528=LINE('',#63648,#10025);
#7529=LINE('',#63653,#10026);
#7530=LINE('',#63656,#10027);
#7531=LINE('',#63658,#10028);
#7532=LINE('',#63661,#10029);
#7533=LINE('',#63664,#10030);
#7534=LINE('',#63665,#10031);
#7535=LINE('',#63667,#10032);
#7536=LINE('',#63670,#10033);
#7537=LINE('',#63671,#10034);
#7538=LINE('',#63679,#10035);
#7539=LINE('',#63685,#10036);
#7540=LINE('',#63686,#10037);
#7541=LINE('',#63688,#10038);
#7542=LINE('',#63690,#10039);
#8746=VECTOR('',#31138,1.);
#8747=VECTOR('',#31139,1.);
#8748=VECTOR('',#31140,1.);
#8749=VECTOR('',#31141,1.);
#8750=VECTOR('',#31142,1.);
#8751=VECTOR('',#31143,1.);
#8752=VECTOR('',#31146,1.);
#8753=VECTOR('',#31147,1.);
#8754=VECTOR('',#31148,1.);
#8755=VECTOR('',#31149,1.);
#8756=VECTOR('',#31152,1.);
#8757=VECTOR('',#31153,1.);
#8758=VECTOR('',#31156,1.);
#8759=VECTOR('',#31157,1.);
#8760=VECTOR('',#31158,1.);
#8761=VECTOR('',#31161,1.);
#8762=VECTOR('',#31162,1.);
#8763=VECTOR('',#31163,1.);
#8764=VECTOR('',#31164,1.);
#8765=VECTOR('',#31165,1.);
#8766=VECTOR('',#31166,1.);
#8767=VECTOR('',#31169,1.);
#8768=VECTOR('',#31170,1.);
#8769=VECTOR('',#31171,1.);
#8770=VECTOR('',#31172,1.);
#8771=VECTOR('',#31175,1.);
#8772=VECTOR('',#31176,1.);
#8773=VECTOR('',#31179,1.);
#8774=VECTOR('',#31180,1.);
#8775=VECTOR('',#31181,1.);
#8776=VECTOR('',#31184,1.);
#8777=VECTOR('',#31185,1.);
#8778=VECTOR('',#31186,1.);
#8779=VECTOR('',#31187,1.);
#8780=VECTOR('',#31188,1.);
#8781=VECTOR('',#31189,1.);
#8782=VECTOR('',#31192,1.);
#8783=VECTOR('',#31193,1.);
#8784=VECTOR('',#31194,1.);
#8785=VECTOR('',#31197,1.);
#8786=VECTOR('',#31198,1.);
#8787=VECTOR('',#31199,1.);
#8788=VECTOR('',#31202,1.);
#8789=VECTOR('',#31203,1.);
#8790=VECTOR('',#31204,1.);
#8791=VECTOR('',#31205,1.);
#8792=VECTOR('',#31208,1.);
#8793=VECTOR('',#31209,1.);
#8794=VECTOR('',#31210,1.);
#8795=VECTOR('',#31211,1.);
#8796=VECTOR('',#31212,1.);
#8797=VECTOR('',#31213,1.);
#8798=VECTOR('',#31216,1.);
#8799=VECTOR('',#31217,1.);
#8800=VECTOR('',#31218,1.);
#8801=VECTOR('',#31219,1.);
#8802=VECTOR('',#31222,1.);
#8803=VECTOR('',#31223,1.);
#8804=VECTOR('',#31226,1.);
#8805=VECTOR('',#31227,1.);
#8806=VECTOR('',#31228,1.);
#8807=VECTOR('',#31231,1.);
#8808=VECTOR('',#31232,1.);
#8809=VECTOR('',#31233,1.);
#8810=VECTOR('',#31234,1.);
#8811=VECTOR('',#31235,1.);
#8812=VECTOR('',#31236,1.);
#8813=VECTOR('',#31239,1.);
#8814=VECTOR('',#31240,1.);
#8815=VECTOR('',#31241,1.);
#8816=VECTOR('',#31244,1.);
#8817=VECTOR('',#31245,1.);
#8818=VECTOR('',#31246,1.);
#8819=VECTOR('',#31247,1.);
#8820=VECTOR('',#31250,1.);
#8821=VECTOR('',#31251,1.);
#8822=VECTOR('',#31252,1.);
#8823=VECTOR('',#31255,1.);
#8824=VECTOR('',#31256,1.);
#8825=VECTOR('',#31257,1.);
#8826=VECTOR('',#31258,1.);
#8827=VECTOR('',#31259,1.);
#8828=VECTOR('',#31260,1.);
#8829=VECTOR('',#31263,1.);
#8830=VECTOR('',#31264,1.);
#8831=VECTOR('',#31265,1.);
#8832=VECTOR('',#31266,1.);
#8833=VECTOR('',#31269,1.);
#8834=VECTOR('',#31270,1.);
#8835=VECTOR('',#31271,1.);
#8836=VECTOR('',#31272,1.);
#8837=VECTOR('',#31275,1.);
#8838=VECTOR('',#31276,1.);
#8839=VECTOR('',#31279,1.);
#8840=VECTOR('',#31280,1.);
#8841=VECTOR('',#31281,1.);
#8842=VECTOR('',#31282,1.);
#8843=VECTOR('',#31285,1.);
#8844=VECTOR('',#31286,1.);
#8845=VECTOR('',#31287,1.);
#8846=VECTOR('',#31290,1.);
#8847=VECTOR('',#31291,1.);
#8848=VECTOR('',#31292,1.);
#8849=VECTOR('',#31293,1.);
#8850=VECTOR('',#31294,1.);
#8851=VECTOR('',#31295,1.);
#8852=VECTOR('',#31298,1.);
#8853=VECTOR('',#31299,1.);
#8854=VECTOR('',#31300,1.);
#8855=VECTOR('',#31303,1.);
#8856=VECTOR('',#31304,1.);
#8857=VECTOR('',#31305,1.);
#8858=VECTOR('',#31308,1.);
#8859=VECTOR('',#31309,1.);
#8860=VECTOR('',#31312,1.);
#8861=VECTOR('',#31313,1.);
#8862=VECTOR('',#31314,1.);
#8863=VECTOR('',#31315,1.);
#8864=VECTOR('',#31316,1.);
#8865=VECTOR('',#31317,1.);
#8866=VECTOR('',#31320,1.);
#8867=VECTOR('',#31321,1.);
#8868=VECTOR('',#31322,1.);
#8869=VECTOR('',#31325,1.);
#8870=VECTOR('',#31326,1.);
#8871=VECTOR('',#31327,1.);
#8872=VECTOR('',#31328,1.);
#8873=VECTOR('',#31331,1.);
#8874=VECTOR('',#31332,1.);
#8875=VECTOR('',#31333,1.);
#8876=VECTOR('',#31336,1.);
#8877=VECTOR('',#31337,1.);
#8878=VECTOR('',#31338,1.);
#8879=VECTOR('',#31339,1.);
#8880=VECTOR('',#31340,1.);
#8881=VECTOR('',#31341,1.);
#8882=VECTOR('',#31344,1.);
#8883=VECTOR('',#31345,1.);
#8884=VECTOR('',#31346,1.);
#8885=VECTOR('',#31347,1.);
#8886=VECTOR('',#31350,1.);
#8887=VECTOR('',#31351,1.);
#8888=VECTOR('',#31352,1.);
#8889=VECTOR('',#31353,1.);
#8890=VECTOR('',#31356,1.);
#8891=VECTOR('',#31357,1.);
#8892=VECTOR('',#31360,1.);
#8893=VECTOR('',#31361,1.);
#8894=VECTOR('',#31362,1.);
#8895=VECTOR('',#31363,1.);
#8896=VECTOR('',#31366,1.);
#8897=VECTOR('',#31367,1.);
#8898=VECTOR('',#31368,1.);
#8899=VECTOR('',#31371,1.);
#8900=VECTOR('',#31372,1.);
#8901=VECTOR('',#31373,1.);
#8902=VECTOR('',#31374,1.);
#8903=VECTOR('',#31375,1.);
#8904=VECTOR('',#31376,1.);
#8905=VECTOR('',#31379,1.);
#8906=VECTOR('',#31380,1.);
#8907=VECTOR('',#31381,1.);
#8908=VECTOR('',#31384,1.);
#8909=VECTOR('',#31385,1.);
#8910=VECTOR('',#31386,1.);
#8911=VECTOR('',#31389,1.);
#8912=VECTOR('',#31390,1.);
#8913=VECTOR('',#31393,1.);
#8914=VECTOR('',#31394,1.);
#8915=VECTOR('',#31395,1.);
#8916=VECTOR('',#31396,1.);
#8917=VECTOR('',#31397,1.);
#8918=VECTOR('',#31398,1.);
#8919=VECTOR('',#31401,1.);
#8920=VECTOR('',#31402,1.);
#8921=VECTOR('',#31403,1.);
#8922=VECTOR('',#31404,1.);
#8923=VECTOR('',#31407,1.);
#8924=VECTOR('',#31408,1.);
#8925=VECTOR('',#31409,1.);
#8926=VECTOR('',#31410,1.);
#8927=VECTOR('',#31413,1.);
#8928=VECTOR('',#31414,1.);
#8929=VECTOR('',#31417,1.);
#8930=VECTOR('',#31418,1.);
#8931=VECTOR('',#31419,1.);
#8932=VECTOR('',#31420,1.);
#8933=VECTOR('',#31423,1.);
#8934=VECTOR('',#31424,1.);
#8935=VECTOR('',#31425,1.);
#8936=VECTOR('',#31428,1.);
#8937=VECTOR('',#31429,1.);
#8938=VECTOR('',#31430,1.);
#8939=VECTOR('',#31431,1.);
#8940=VECTOR('',#31432,1.);
#8941=VECTOR('',#31433,1.);
#8942=VECTOR('',#31436,1.);
#8943=VECTOR('',#31437,1.);
#8944=VECTOR('',#31438,1.);
#8945=VECTOR('',#31441,1.);
#8946=VECTOR('',#31442,1.);
#8947=VECTOR('',#31443,1.);
#8948=VECTOR('',#31446,1.);
#8949=VECTOR('',#31447,1.);
#8950=VECTOR('',#31448,1.);
#8951=VECTOR('',#31449,1.);
#8952=VECTOR('',#31452,1.);
#8953=VECTOR('',#31453,1.);
#8954=VECTOR('',#31454,1.);
#8955=VECTOR('',#31455,1.);
#8956=VECTOR('',#31456,1.);
#8957=VECTOR('',#31459,1.);
#8958=VECTOR('',#31460,1.);
#8959=VECTOR('',#31461,1.);
#8960=VECTOR('',#31464,1.);
#8961=VECTOR('',#31465,1.);
#8962=VECTOR('',#31466,1.);
#8963=VECTOR('',#31469,1.);
#8964=VECTOR('',#31470,1.);
#8965=VECTOR('',#31471,1.);
#8966=VECTOR('',#31474,1.);
#8967=VECTOR('',#31475,1.);
#8968=VECTOR('',#31476,1.);
#8969=VECTOR('',#31477,1.);
#8970=VECTOR('',#31478,1.);
#8971=VECTOR('',#31479,1.);
#8972=VECTOR('',#31482,1.);
#8973=VECTOR('',#31483,1.);
#8974=VECTOR('',#31484,1.);
#8975=VECTOR('',#31485,1.);
#8976=VECTOR('',#31488,1.);
#8977=VECTOR('',#31489,1.);
#8978=VECTOR('',#31490,1.);
#8979=VECTOR('',#31491,1.);
#8980=VECTOR('',#31494,1.);
#8981=VECTOR('',#31495,1.);
#8982=VECTOR('',#31498,1.);
#8983=VECTOR('',#31499,1.);
#8984=VECTOR('',#31500,1.);
#8985=VECTOR('',#31501,1.);
#8986=VECTOR('',#31504,1.);
#8987=VECTOR('',#31505,1.);
#8988=VECTOR('',#31506,1.);
#8989=VECTOR('',#31509,1.);
#8990=VECTOR('',#31510,1.);
#8991=VECTOR('',#31511,1.);
#8992=VECTOR('',#31512,1.);
#8993=VECTOR('',#31513,1.);
#8994=VECTOR('',#31514,1.);
#8995=VECTOR('',#31517,1.);
#8996=VECTOR('',#31518,1.);
#8997=VECTOR('',#31519,1.);
#8998=VECTOR('',#31520,1.);
#8999=VECTOR('',#31523,1.);
#9000=VECTOR('',#31524,1.);
#9001=VECTOR('',#31525,1.);
#9002=VECTOR('',#31526,1.);
#9003=VECTOR('',#31529,1.);
#9004=VECTOR('',#31530,1.);
#9005=VECTOR('',#31533,1.);
#9006=VECTOR('',#31534,1.);
#9007=VECTOR('',#31535,1.);
#9008=VECTOR('',#31536,1.);
#9009=VECTOR('',#31539,1.);
#9010=VECTOR('',#31540,1.);
#9011=VECTOR('',#31541,1.);
#9012=VECTOR('',#31544,1.);
#9013=VECTOR('',#31545,1.);
#9014=VECTOR('',#31546,1.);
#9015=VECTOR('',#31547,1.);
#9016=VECTOR('',#31548,1.);
#9017=VECTOR('',#31549,1.);
#9018=VECTOR('',#31552,1.);
#9019=VECTOR('',#31553,1.);
#9020=VECTOR('',#31554,1.);
#9021=VECTOR('',#31555,1.);
#9022=VECTOR('',#31558,1.);
#9023=VECTOR('',#31559,1.);
#9024=VECTOR('',#31562,1.);
#9025=VECTOR('',#31563,1.);
#9026=VECTOR('',#31564,1.);
#9027=VECTOR('',#31567,1.);
#9028=VECTOR('',#31568,1.);
#9029=VECTOR('',#31569,1.);
#9030=VECTOR('',#31570,1.);
#9031=VECTOR('',#31571,1.);
#9032=VECTOR('',#31572,1.);
#9033=VECTOR('',#31575,1.);
#9034=VECTOR('',#31576,1.);
#9035=VECTOR('',#31577,1.);
#9036=VECTOR('',#31578,1.);
#9037=VECTOR('',#31581,1.);
#9038=VECTOR('',#31582,1.);
#9039=VECTOR('',#31583,1.);
#9040=VECTOR('',#31584,1.);
#9041=VECTOR('',#31587,1.);
#9042=VECTOR('',#31588,1.);
#9043=VECTOR('',#31591,1.);
#9044=VECTOR('',#31592,1.);
#9045=VECTOR('',#31593,1.);
#9046=VECTOR('',#31594,1.);
#9047=VECTOR('',#31597,1.);
#9048=VECTOR('',#31598,1.);
#9049=VECTOR('',#31599,1.);
#9050=VECTOR('',#31602,1.);
#9051=VECTOR('',#31603,1.);
#9052=VECTOR('',#31604,1.);
#9053=VECTOR('',#31605,1.);
#9054=VECTOR('',#31606,1.);
#9055=VECTOR('',#31607,1.);
#9056=VECTOR('',#31610,1.);
#9057=VECTOR('',#31611,1.);
#9058=VECTOR('',#31612,1.);
#9059=VECTOR('',#31613,1.);
#9060=VECTOR('',#31616,1.);
#9061=VECTOR('',#31617,1.);
#9062=VECTOR('',#31618,1.);
#9063=VECTOR('',#31619,1.);
#9064=VECTOR('',#31622,1.);
#9065=VECTOR('',#31623,1.);
#9066=VECTOR('',#31626,1.);
#9067=VECTOR('',#31627,1.);
#9068=VECTOR('',#31628,1.);
#9069=VECTOR('',#31629,1.);
#9070=VECTOR('',#31632,1.);
#9071=VECTOR('',#31633,1.);
#9072=VECTOR('',#31634,1.);
#9073=VECTOR('',#31637,1.);
#9074=VECTOR('',#31638,1.);
#9075=VECTOR('',#31639,1.);
#9076=VECTOR('',#31640,1.);
#9077=VECTOR('',#31641,1.);
#9078=VECTOR('',#31644,1.);
#9079=VECTOR('',#31645,1.);
#9080=VECTOR('',#31646,1.);
#9081=VECTOR('',#31649,1.);
#9082=VECTOR('',#31650,1.);
#9083=VECTOR('',#31653,1.);
#9084=VECTOR('',#31654,1.);
#9085=VECTOR('',#31655,1.);
#9086=VECTOR('',#31658,1.);
#9087=VECTOR('',#31659,1.);
#9088=VECTOR('',#31660,1.);
#9089=VECTOR('',#31661,1.);
#9090=VECTOR('',#31664,1.);
#9091=VECTOR('',#31665,1.);
#9092=VECTOR('',#31666,1.);
#9093=VECTOR('',#31671,1.);
#9094=VECTOR('',#31672,1.);
#9095=VECTOR('',#31673,1.);
#9096=VECTOR('',#31674,1.);
#9097=VECTOR('',#31677,1.);
#9098=VECTOR('',#31678,1.);
#9099=VECTOR('',#31679,1.);
#9100=VECTOR('',#31680,1.);
#9101=VECTOR('',#31681,1.);
#9102=VECTOR('',#31682,1.);
#9103=VECTOR('',#31685,1.);
#9104=VECTOR('',#31686,1.);
#9105=VECTOR('',#31689,1.);
#9106=VECTOR('',#31690,1.);
#9107=VECTOR('',#31691,1.);
#9108=VECTOR('',#31692,1.);
#9109=VECTOR('',#31693,1.);
#9110=VECTOR('',#31696,1.);
#9111=VECTOR('',#31697,1.);
#9112=VECTOR('',#31698,1.);
#9113=VECTOR('',#31699,1.);
#9114=VECTOR('',#31702,1.);
#9115=VECTOR('',#31705,1.);
#9116=VECTOR('',#31706,1.);
#9117=VECTOR('',#31707,1.);
#9118=VECTOR('',#31708,1.);
#9119=VECTOR('',#31709,1.);
#9120=VECTOR('',#31710,1.);
#9121=VECTOR('',#31713,1.);
#9122=VECTOR('',#31714,1.);
#9123=VECTOR('',#31715,1.);
#9124=VECTOR('',#31716,1.);
#9125=VECTOR('',#31719,1.);
#9126=VECTOR('',#31720,1.);
#9127=VECTOR('',#31721,1.);
#9128=VECTOR('',#31722,1.);
#9129=VECTOR('',#31725,1.);
#9130=VECTOR('',#31726,1.);
#9131=VECTOR('',#31729,1.);
#9132=VECTOR('',#31730,1.);
#9133=VECTOR('',#31731,1.);
#9134=VECTOR('',#31732,1.);
#9135=VECTOR('',#31733,1.);
#9136=VECTOR('',#31734,1.);
#9137=VECTOR('',#31737,1.);
#9138=VECTOR('',#31738,1.);
#9139=VECTOR('',#31739,1.);
#9140=VECTOR('',#31740,1.);
#9141=VECTOR('',#31743,1.);
#9142=VECTOR('',#31744,1.);
#9143=VECTOR('',#31745,1.);
#9144=VECTOR('',#31746,1.);
#9145=VECTOR('',#31749,1.);
#9146=VECTOR('',#31750,1.);
#9147=VECTOR('',#31753,1.);
#9148=VECTOR('',#31754,1.);
#9149=VECTOR('',#31755,1.);
#9150=VECTOR('',#31756,1.);
#9151=VECTOR('',#31759,1.);
#9152=VECTOR('',#31760,1.);
#9153=VECTOR('',#31761,1.);
#9154=VECTOR('',#31764,1.);
#9155=VECTOR('',#31765,1.);
#9156=VECTOR('',#31766,1.);
#9157=VECTOR('',#31767,1.);
#9158=VECTOR('',#31768,1.);
#9159=VECTOR('',#31769,1.);
#9160=VECTOR('',#31772,1.);
#9161=VECTOR('',#31773,1.);
#9162=VECTOR('',#31774,1.);
#9163=VECTOR('',#31775,1.);
#9164=VECTOR('',#31778,1.);
#9165=VECTOR('',#31779,1.);
#9166=VECTOR('',#31780,1.);
#9167=VECTOR('',#31781,1.);
#9168=VECTOR('',#31784,1.);
#9169=VECTOR('',#31785,1.);
#9170=VECTOR('',#31788,1.);
#9171=VECTOR('',#31789,1.);
#9172=VECTOR('',#31790,1.);
#9173=VECTOR('',#31791,1.);
#9174=VECTOR('',#31794,1.);
#9175=VECTOR('',#31795,1.);
#9176=VECTOR('',#31796,1.);
#9177=VECTOR('',#31799,1.);
#9178=VECTOR('',#31800,1.);
#9179=VECTOR('',#31801,1.);
#9180=VECTOR('',#31802,1.);
#9181=VECTOR('',#31803,1.);
#9182=VECTOR('',#31804,1.);
#9183=VECTOR('',#31807,1.);
#9184=VECTOR('',#31808,1.);
#9185=VECTOR('',#31809,1.);
#9186=VECTOR('',#31810,1.);
#9187=VECTOR('',#31813,1.);
#9188=VECTOR('',#31814,1.);
#9189=VECTOR('',#31815,1.);
#9190=VECTOR('',#31816,1.);
#9191=VECTOR('',#31819,1.);
#9192=VECTOR('',#31820,1.);
#9193=VECTOR('',#31823,1.);
#9194=VECTOR('',#31824,1.);
#9195=VECTOR('',#31825,1.);
#9196=VECTOR('',#31826,1.);
#9197=VECTOR('',#31829,1.);
#9198=VECTOR('',#31830,1.);
#9199=VECTOR('',#31831,1.);
#9200=VECTOR('',#31834,1.);
#9201=VECTOR('',#31835,1.);
#9202=VECTOR('',#31836,1.);
#9203=VECTOR('',#31837,1.);
#9204=VECTOR('',#31838,1.);
#9205=VECTOR('',#31839,1.);
#9206=VECTOR('',#31842,1.);
#9207=VECTOR('',#31843,1.);
#9208=VECTOR('',#31844,1.);
#9209=VECTOR('',#31845,1.);
#9210=VECTOR('',#31848,1.);
#9211=VECTOR('',#31849,1.);
#9212=VECTOR('',#31850,1.);
#9213=VECTOR('',#31851,1.);
#9214=VECTOR('',#31854,1.);
#9215=VECTOR('',#31855,1.);
#9216=VECTOR('',#31858,1.);
#9217=VECTOR('',#31859,1.);
#9218=VECTOR('',#31860,1.);
#9219=VECTOR('',#31861,1.);
#9220=VECTOR('',#31864,1.);
#9221=VECTOR('',#31865,1.);
#9222=VECTOR('',#31866,1.);
#9223=VECTOR('',#31869,1.);
#9224=VECTOR('',#31870,1.);
#9225=VECTOR('',#31871,1.);
#9226=VECTOR('',#31872,1.);
#9227=VECTOR('',#31873,1.);
#9228=VECTOR('',#31874,1.);
#9229=VECTOR('',#31877,1.);
#9230=VECTOR('',#31878,1.);
#9231=VECTOR('',#31879,1.);
#9232=VECTOR('',#31882,1.);
#9233=VECTOR('',#31883,1.);
#9234=VECTOR('',#31884,1.);
#9235=VECTOR('',#31887,1.);
#9236=VECTOR('',#31888,1.);
#9237=VECTOR('',#31891,1.);
#9238=VECTOR('',#31892,1.);
#9239=VECTOR('',#31895,1.);
#9240=VECTOR('',#31896,1.);
#9241=VECTOR('',#31899,1.);
#9242=VECTOR('',#31902,1.);
#9243=VECTOR('',#31903,1.);
#9244=VECTOR('',#31906,1.);
#9245=VECTOR('',#31907,1.);
#9246=VECTOR('',#31910,1.);
#9247=VECTOR('',#31911,1.);
#9248=VECTOR('',#31914,1.);
#9249=VECTOR('',#31917,1.);
#9250=VECTOR('',#31918,1.);
#9251=VECTOR('',#31921,1.);
#9252=VECTOR('',#31922,1.);
#9253=VECTOR('',#31925,1.);
#9254=VECTOR('',#31928,1.);
#9255=VECTOR('',#31929,1.);
#9256=VECTOR('',#31930,1.);
#9257=VECTOR('',#31931,1.);
#9258=VECTOR('',#31932,1.);
#9259=VECTOR('',#31933,1.);
#9260=VECTOR('',#31934,1.);
#9261=VECTOR('',#31935,1.);
#9262=VECTOR('',#31936,1.);
#9263=VECTOR('',#31937,1.);
#9264=VECTOR('',#31938,1.);
#9265=VECTOR('',#31939,1.);
#9266=VECTOR('',#31940,1.);
#9267=VECTOR('',#31941,1.);
#9268=VECTOR('',#31942,1.);
#9269=VECTOR('',#31943,1.);
#9270=VECTOR('',#31944,1.);
#9271=VECTOR('',#31945,1.);
#9272=VECTOR('',#31946,1.);
#9273=VECTOR('',#31947,1.);
#9274=VECTOR('',#31948,1.);
#9275=VECTOR('',#31949,1.);
#9276=VECTOR('',#31950,1.);
#9277=VECTOR('',#31951,1.);
#9278=VECTOR('',#31952,1.);
#9279=VECTOR('',#31953,1.);
#9280=VECTOR('',#31954,1.);
#9281=VECTOR('',#31955,1.);
#9282=VECTOR('',#31956,1.);
#9283=VECTOR('',#31957,1.);
#9284=VECTOR('',#31958,1.);
#9285=VECTOR('',#31959,1.);
#9286=VECTOR('',#31960,1.);
#9287=VECTOR('',#31961,1.);
#9288=VECTOR('',#31962,1.);
#9289=VECTOR('',#31963,1.);
#9290=VECTOR('',#31964,1.);
#9291=VECTOR('',#31965,1.);
#9292=VECTOR('',#31966,1.);
#9293=VECTOR('',#31967,1.);
#9294=VECTOR('',#31968,1.);
#9295=VECTOR('',#31969,1.);
#9296=VECTOR('',#31970,1.);
#9297=VECTOR('',#31971,1.);
#9298=VECTOR('',#31972,1.);
#9299=VECTOR('',#31973,1.);
#9300=VECTOR('',#31974,1.);
#9301=VECTOR('',#31975,1.);
#9302=VECTOR('',#31976,1.);
#9303=VECTOR('',#31977,1.);
#9304=VECTOR('',#31978,1.);
#9305=VECTOR('',#31979,1.);
#9306=VECTOR('',#31980,1.);
#9307=VECTOR('',#31981,1.);
#9308=VECTOR('',#31982,1.);
#9309=VECTOR('',#31983,1.);
#9310=VECTOR('',#31984,1.);
#9311=VECTOR('',#31985,1.);
#9312=VECTOR('',#31986,1.);
#9313=VECTOR('',#31987,1.);
#9314=VECTOR('',#31988,1.);
#9315=VECTOR('',#31989,1.);
#9316=VECTOR('',#31990,1.);
#9317=VECTOR('',#31991,1.);
#9318=VECTOR('',#31992,1.);
#9319=VECTOR('',#31993,1.);
#9320=VECTOR('',#31994,1.);
#9321=VECTOR('',#31995,1.);
#9322=VECTOR('',#31996,1.);
#9323=VECTOR('',#31997,1.);
#9324=VECTOR('',#31998,1.);
#9325=VECTOR('',#31999,1.);
#9326=VECTOR('',#32000,1.);
#9327=VECTOR('',#32001,1.);
#9328=VECTOR('',#32002,1.);
#9329=VECTOR('',#32005,1.);
#9330=VECTOR('',#32008,1.);
#9331=VECTOR('',#32009,1.);
#9332=VECTOR('',#32012,1.);
#9333=VECTOR('',#32015,1.);
#9334=VECTOR('',#32018,1.);
#9335=VECTOR('',#32019,1.);
#9336=VECTOR('',#32022,1.);
#9337=VECTOR('',#32023,1.);
#9338=VECTOR('',#32026,1.);
#9339=VECTOR('',#32029,1.);
#9340=VECTOR('',#32032,1.);
#9341=VECTOR('',#32033,1.);
#9342=VECTOR('',#32036,1.);
#9343=VECTOR('',#32037,1.);
#9344=VECTOR('',#32040,1.);
#9345=VECTOR('',#32043,1.);
#9346=VECTOR('',#32046,1.);
#9347=VECTOR('',#32047,1.);
#9348=VECTOR('',#32050,1.);
#9349=VECTOR('',#32051,1.);
#9350=VECTOR('',#32054,1.);
#9351=VECTOR('',#32057,1.);
#9352=VECTOR('',#32058,1.);
#9353=VECTOR('',#32061,1.);
#9354=VECTOR('',#32062,1.);
#9355=VECTOR('',#32065,1.);
#9356=VECTOR('',#32066,1.);
#9357=VECTOR('',#32069,1.);
#9358=VECTOR('',#32070,1.);
#9359=VECTOR('',#32071,1.);
#9360=VECTOR('',#32072,1.);
#9361=VECTOR('',#32075,1.);
#9362=VECTOR('',#32076,1.);
#9363=VECTOR('',#32077,1.);
#9364=VECTOR('',#32078,1.);
#9365=VECTOR('',#32081,1.);
#9366=VECTOR('',#32082,1.);
#9367=VECTOR('',#32085,1.);
#9368=VECTOR('',#32086,1.);
#9369=VECTOR('',#32087,1.);
#9370=VECTOR('',#32090,1.);
#9371=VECTOR('',#32091,1.);
#9372=VECTOR('',#32092,1.);
#9373=VECTOR('',#32095,1.);
#9374=VECTOR('',#32096,1.);
#9375=VECTOR('',#32097,1.);
#9376=VECTOR('',#32100,1.);
#9377=VECTOR('',#32101,1.);
#9378=VECTOR('',#32102,1.);
#9379=VECTOR('',#32103,1.);
#9380=VECTOR('',#32106,1.);
#9381=VECTOR('',#32107,1.);
#9382=VECTOR('',#32110,1.);
#9383=VECTOR('',#32111,1.);
#9384=VECTOR('',#32112,1.);
#9385=VECTOR('',#32113,1.);
#9386=VECTOR('',#32114,1.);
#9387=VECTOR('',#32115,1.);
#9388=VECTOR('',#32118,1.);
#9389=VECTOR('',#32119,1.);
#9390=VECTOR('',#32120,1.);
#9391=VECTOR('',#32123,1.);
#9392=VECTOR('',#32124,1.);
#9393=VECTOR('',#32125,1.);
#9394=VECTOR('',#32128,1.);
#9395=VECTOR('',#32129,1.);
#9396=VECTOR('',#32132,1.);
#9397=VECTOR('',#32133,1.);
#9398=VECTOR('',#32134,1.);
#9399=VECTOR('',#32135,1.);
#9400=VECTOR('',#32138,1.);
#9401=VECTOR('',#32141,1.);
#9402=VECTOR('',#32144,1.);
#9403=VECTOR('',#32147,1.);
#9404=VECTOR('',#32148,1.);
#9405=VECTOR('',#32151,1.);
#9406=VECTOR('',#32152,1.);
#9407=VECTOR('',#32155,1.);
#9408=VECTOR('',#32158,1.);
#9409=VECTOR('',#32161,1.);
#9410=VECTOR('',#32162,1.);
#9411=VECTOR('',#32165,1.);
#9412=VECTOR('',#32168,1.);
#9413=VECTOR('',#32171,1.);
#9414=VECTOR('',#32172,1.);
#9415=VECTOR('',#32175,1.);
#9416=VECTOR('',#32176,1.);
#9417=VECTOR('',#32179,1.);
#9418=VECTOR('',#32182,1.);
#9419=VECTOR('',#32185,1.);
#9420=VECTOR('',#32188,1.);
#9421=VECTOR('',#32189,1.);
#9422=VECTOR('',#32192,1.);
#9423=VECTOR('',#32195,1.);
#9424=VECTOR('',#32198,1.);
#9425=VECTOR('',#32199,1.);
#9426=VECTOR('',#32202,1.);
#9427=VECTOR('',#32205,1.);
#9428=VECTOR('',#32208,1.);
#9429=VECTOR('',#32209,1.);
#9430=VECTOR('',#32212,1.);
#9431=VECTOR('',#32215,1.);
#9432=VECTOR('',#32218,1.);
#9433=VECTOR('',#32219,1.);
#9434=VECTOR('',#32222,1.);
#9435=VECTOR('',#32225,1.);
#9436=VECTOR('',#32228,1.);
#9437=VECTOR('',#32229,1.);
#9438=VECTOR('',#32232,1.);
#9439=VECTOR('',#32233,1.);
#9440=VECTOR('',#32236,1.);
#9441=VECTOR('',#32239,1.);
#9442=VECTOR('',#32240,1.);
#9443=VECTOR('',#32241,1.);
#9444=VECTOR('',#32242,1.);
#9445=VECTOR('',#32243,1.);
#9446=VECTOR('',#32244,1.);
#9447=VECTOR('',#32247,1.);
#9448=VECTOR('',#32248,1.);
#9449=VECTOR('',#32249,1.);
#9450=VECTOR('',#32252,1.);
#9451=VECTOR('',#32253,1.);
#9452=VECTOR('',#32254,1.);
#9453=VECTOR('',#32257,1.);
#9454=VECTOR('',#32258,1.);
#9455=VECTOR('',#32261,1.);
#9456=VECTOR('',#32262,1.);
#9457=VECTOR('',#32263,1.);
#9458=VECTOR('',#32264,1.);
#9459=VECTOR('',#32267,1.);
#9460=VECTOR('',#32268,1.);
#9461=VECTOR('',#32271,1.);
#9462=VECTOR('',#32272,1.);
#9463=VECTOR('',#32273,1.);
#9464=VECTOR('',#32274,1.);
#9465=VECTOR('',#32275,1.);
#9466=VECTOR('',#32276,1.);
#9467=VECTOR('',#32279,1.);
#9468=VECTOR('',#32280,1.);
#9469=VECTOR('',#32281,1.);
#9470=VECTOR('',#32284,1.);
#9471=VECTOR('',#32285,1.);
#9472=VECTOR('',#32286,1.);
#9473=VECTOR('',#32289,1.);
#9474=VECTOR('',#32290,1.);
#9475=VECTOR('',#32293,1.);
#9476=VECTOR('',#32294,1.);
#9477=VECTOR('',#32295,1.);
#9478=VECTOR('',#32296,1.);
#9479=VECTOR('',#32299,1.);
#9480=VECTOR('',#32300,1.);
#9481=VECTOR('',#32303,1.);
#9482=VECTOR('',#32304,1.);
#9483=VECTOR('',#32305,1.);
#9484=VECTOR('',#32306,1.);
#9485=VECTOR('',#32307,1.);
#9486=VECTOR('',#32308,1.);
#9487=VECTOR('',#32311,1.);
#9488=VECTOR('',#32312,1.);
#9489=VECTOR('',#32313,1.);
#9490=VECTOR('',#32316,1.);
#9491=VECTOR('',#32317,1.);
#9492=VECTOR('',#32318,1.);
#9493=VECTOR('',#32321,1.);
#9494=VECTOR('',#32322,1.);
#9495=VECTOR('',#32325,1.);
#9496=VECTOR('',#32326,1.);
#9497=VECTOR('',#32327,1.);
#9498=VECTOR('',#32328,1.);
#9499=VECTOR('',#32331,1.);
#9500=VECTOR('',#32332,1.);
#9501=VECTOR('',#32335,1.);
#9502=VECTOR('',#32336,1.);
#9503=VECTOR('',#32337,1.);
#9504=VECTOR('',#32338,1.);
#9505=VECTOR('',#32339,1.);
#9506=VECTOR('',#32340,1.);
#9507=VECTOR('',#32343,1.);
#9508=VECTOR('',#32344,1.);
#9509=VECTOR('',#32345,1.);
#9510=VECTOR('',#32348,1.);
#9511=VECTOR('',#32349,1.);
#9512=VECTOR('',#32352,1.);
#9513=VECTOR('',#32353,1.);
#9514=VECTOR('',#32354,1.);
#9515=VECTOR('',#32357,1.);
#9516=VECTOR('',#32358,1.);
#9517=VECTOR('',#32359,1.);
#9518=VECTOR('',#32360,1.);
#9519=VECTOR('',#32361,1.);
#9520=VECTOR('',#32364,1.);
#9521=VECTOR('',#32365,1.);
#9522=VECTOR('',#32366,1.);
#9523=VECTOR('',#32369,1.);
#9524=VECTOR('',#32370,1.);
#9525=VECTOR('',#32371,1.);
#9526=VECTOR('',#32374,1.);
#9527=VECTOR('',#32375,1.);
#9528=VECTOR('',#32376,1.);
#9529=VECTOR('',#32379,1.);
#9530=VECTOR('',#32380,1.);
#9531=VECTOR('',#32381,1.);
#9532=VECTOR('',#32382,1.);
#9533=VECTOR('',#32383,1.);
#9534=VECTOR('',#32384,1.);
#9535=VECTOR('',#32387,1.);
#9536=VECTOR('',#32388,1.);
#9537=VECTOR('',#32389,1.);
#9538=VECTOR('',#32392,1.);
#9539=VECTOR('',#32393,1.);
#9540=VECTOR('',#32394,1.);
#9541=VECTOR('',#32397,1.);
#9542=VECTOR('',#32398,1.);
#9543=VECTOR('',#32401,1.);
#9544=VECTOR('',#32402,1.);
#9545=VECTOR('',#32403,1.);
#9546=VECTOR('',#32404,1.);
#9547=VECTOR('',#32407,1.);
#9548=VECTOR('',#32408,1.);
#9549=VECTOR('',#32411,1.);
#9550=VECTOR('',#32412,1.);
#9551=VECTOR('',#32413,1.);
#9552=VECTOR('',#32414,1.);
#9553=VECTOR('',#32415,1.);
#9554=VECTOR('',#32416,1.);
#9555=VECTOR('',#32419,1.);
#9556=VECTOR('',#32420,1.);
#9557=VECTOR('',#32421,1.);
#9558=VECTOR('',#32424,1.);
#9559=VECTOR('',#32425,1.);
#9560=VECTOR('',#32426,1.);
#9561=VECTOR('',#32429,1.);
#9562=VECTOR('',#32430,1.);
#9563=VECTOR('',#32433,1.);
#9564=VECTOR('',#32434,1.);
#9565=VECTOR('',#32435,1.);
#9566=VECTOR('',#32436,1.);
#9567=VECTOR('',#32439,1.);
#9568=VECTOR('',#32440,1.);
#9569=VECTOR('',#32443,1.);
#9570=VECTOR('',#32444,1.);
#9571=VECTOR('',#32445,1.);
#9572=VECTOR('',#32446,1.);
#9573=VECTOR('',#32449,1.);
#9574=VECTOR('',#32450,1.);
#9575=VECTOR('',#32451,1.);
#9576=VECTOR('',#32452,1.);
#9577=VECTOR('',#32455,1.);
#9578=VECTOR('',#32456,1.);
#9579=VECTOR('',#32459,1.);
#9580=VECTOR('',#32462,1.);
#9581=VECTOR('',#32465,1.);
#9582=VECTOR('',#32466,1.);
#9583=VECTOR('',#32469,1.);
#9584=VECTOR('',#32472,1.);
#9585=VECTOR('',#32475,1.);
#9586=VECTOR('',#32476,1.);
#9587=VECTOR('',#32479,1.);
#9588=VECTOR('',#32480,1.);
#9589=VECTOR('',#32483,1.);
#9590=VECTOR('',#32486,1.);
#9591=VECTOR('',#32489,1.);
#9592=VECTOR('',#32492,1.);
#9593=VECTOR('',#32493,1.);
#9594=VECTOR('',#32496,1.);
#9595=VECTOR('',#32499,1.);
#9596=VECTOR('',#32502,1.);
#9597=VECTOR('',#32503,1.);
#9598=VECTOR('',#32506,1.);
#9599=VECTOR('',#32509,1.);
#9600=VECTOR('',#32512,1.);
#9601=VECTOR('',#32513,1.);
#9602=VECTOR('',#32516,1.);
#9603=VECTOR('',#32517,1.);
#9604=VECTOR('',#32520,1.);
#9605=VECTOR('',#32523,1.);
#9606=VECTOR('',#32526,1.);
#9607=VECTOR('',#32527,1.);
#9608=VECTOR('',#32530,1.);
#9609=VECTOR('',#32531,1.);
#9610=VECTOR('',#32534,1.);
#9611=VECTOR('',#32537,1.);
#9612=VECTOR('',#32540,1.);
#9613=VECTOR('',#32541,1.);
#9614=VECTOR('',#32544,1.);
#9615=VECTOR('',#32547,1.);
#9616=VECTOR('',#32550,1.);
#9617=VECTOR('',#32551,1.);
#9618=VECTOR('',#32554,1.);
#9619=VECTOR('',#32557,1.);
#9620=VECTOR('',#32560,1.);
#9621=VECTOR('',#32561,1.);
#9622=VECTOR('',#32564,1.);
#9623=VECTOR('',#32565,1.);
#9624=VECTOR('',#32568,1.);
#9625=VECTOR('',#32571,1.);
#9626=VECTOR('',#32572,1.);
#9627=VECTOR('',#32573,1.);
#9628=VECTOR('',#32574,1.);
#9629=VECTOR('',#32575,1.);
#9630=VECTOR('',#32576,1.);
#9631=VECTOR('',#32579,1.);
#9632=VECTOR('',#32580,1.);
#9633=VECTOR('',#32581,1.);
#9634=VECTOR('',#32584,1.);
#9635=VECTOR('',#32585,1.);
#9636=VECTOR('',#32586,1.);
#9637=VECTOR('',#32589,1.);
#9638=VECTOR('',#32590,1.);
#9639=VECTOR('',#32593,1.);
#9640=VECTOR('',#32594,1.);
#9641=VECTOR('',#32595,1.);
#9642=VECTOR('',#32596,1.);
#9643=VECTOR('',#32599,1.);
#9644=VECTOR('',#32600,1.);
#9645=VECTOR('',#32603,1.);
#9646=VECTOR('',#32604,1.);
#9647=VECTOR('',#32605,1.);
#9648=VECTOR('',#32606,1.);
#9649=VECTOR('',#32607,1.);
#9650=VECTOR('',#32608,1.);
#9651=VECTOR('',#32611,1.);
#9652=VECTOR('',#32612,1.);
#9653=VECTOR('',#32613,1.);
#9654=VECTOR('',#32616,1.);
#9655=VECTOR('',#32617,1.);
#9656=VECTOR('',#32618,1.);
#9657=VECTOR('',#32621,1.);
#9658=VECTOR('',#32622,1.);
#9659=VECTOR('',#32625,1.);
#9660=VECTOR('',#32626,1.);
#9661=VECTOR('',#32627,1.);
#9662=VECTOR('',#32628,1.);
#9663=VECTOR('',#32631,1.);
#9664=VECTOR('',#32632,1.);
#9665=VECTOR('',#32635,1.);
#9666=VECTOR('',#32636,1.);
#9667=VECTOR('',#32637,1.);
#9668=VECTOR('',#32638,1.);
#9669=VECTOR('',#32639,1.);
#9670=VECTOR('',#32640,1.);
#9671=VECTOR('',#32643,1.);
#9672=VECTOR('',#32644,1.);
#9673=VECTOR('',#32645,1.);
#9674=VECTOR('',#32648,1.);
#9675=VECTOR('',#32649,1.);
#9676=VECTOR('',#32650,1.);
#9677=VECTOR('',#32653,1.);
#9678=VECTOR('',#32654,1.);
#9679=VECTOR('',#32657,1.);
#9680=VECTOR('',#32658,1.);
#9681=VECTOR('',#32659,1.);
#9682=VECTOR('',#32660,1.);
#9683=VECTOR('',#32663,1.);
#9684=VECTOR('',#32664,1.);
#9685=VECTOR('',#32667,1.);
#9686=VECTOR('',#32668,1.);
#9687=VECTOR('',#32669,1.);
#9688=VECTOR('',#32670,1.);
#9689=VECTOR('',#32671,1.);
#9690=VECTOR('',#32672,1.);
#9691=VECTOR('',#32675,1.);
#9692=VECTOR('',#32676,1.);
#9693=VECTOR('',#32677,1.);
#9694=VECTOR('',#32680,1.);
#9695=VECTOR('',#32681,1.);
#9696=VECTOR('',#32682,1.);
#9697=VECTOR('',#32685,1.);
#9698=VECTOR('',#32686,1.);
#9699=VECTOR('',#32689,1.);
#9700=VECTOR('',#32690,1.);
#9701=VECTOR('',#32691,1.);
#9702=VECTOR('',#32692,1.);
#9703=VECTOR('',#32695,1.);
#9704=VECTOR('',#32696,1.);
#9705=VECTOR('',#32699,1.);
#9706=VECTOR('',#32700,1.);
#9707=VECTOR('',#32701,1.);
#9708=VECTOR('',#32702,1.);
#9709=VECTOR('',#32703,1.);
#9710=VECTOR('',#32704,1.);
#9711=VECTOR('',#32707,1.);
#9712=VECTOR('',#32708,1.);
#9713=VECTOR('',#32709,1.);
#9714=VECTOR('',#32712,1.);
#9715=VECTOR('',#32713,1.);
#9716=VECTOR('',#32714,1.);
#9717=VECTOR('',#32717,1.);
#9718=VECTOR('',#32718,1.);
#9719=VECTOR('',#32721,1.);
#9720=VECTOR('',#32722,1.);
#9721=VECTOR('',#32723,1.);
#9722=VECTOR('',#32724,1.);
#9723=VECTOR('',#32727,1.);
#9724=VECTOR('',#32728,1.);
#9725=VECTOR('',#32731,1.);
#9726=VECTOR('',#32732,1.);
#9727=VECTOR('',#32733,1.);
#9728=VECTOR('',#32734,1.);
#9729=VECTOR('',#32735,1.);
#9730=VECTOR('',#32736,1.);
#9731=VECTOR('',#32739,1.);
#9732=VECTOR('',#32740,1.);
#9733=VECTOR('',#32741,1.);
#9734=VECTOR('',#32744,1.);
#9735=VECTOR('',#32745,1.);
#9736=VECTOR('',#32746,1.);
#9737=VECTOR('',#32749,1.);
#9738=VECTOR('',#32750,1.);
#9739=VECTOR('',#32753,1.);
#9740=VECTOR('',#32754,1.);
#9741=VECTOR('',#32755,1.);
#9742=VECTOR('',#32756,1.);
#9743=VECTOR('',#32759,1.);
#9744=VECTOR('',#32760,1.);
#9745=VECTOR('',#32763,1.);
#9746=VECTOR('',#32764,1.);
#9747=VECTOR('',#32765,1.);
#9748=VECTOR('',#32766,1.);
#9749=VECTOR('',#32769,1.);
#9750=VECTOR('',#32770,1.);
#9751=VECTOR('',#32771,1.);
#9752=VECTOR('',#32772,1.);
#9753=VECTOR('',#32775,1.);
#9754=VECTOR('',#32776,1.);
#9755=VECTOR('',#32779,1.);
#9756=VECTOR('',#32782,1.);
#9757=VECTOR('',#32785,1.);
#9758=VECTOR('',#32786,1.);
#9759=VECTOR('',#32789,1.);
#9760=VECTOR('',#32792,1.);
#9761=VECTOR('',#32795,1.);
#9762=VECTOR('',#32796,1.);
#9763=VECTOR('',#32799,1.);
#9764=VECTOR('',#32800,1.);
#9765=VECTOR('',#32803,1.);
#9766=VECTOR('',#32806,1.);
#9767=VECTOR('',#32809,1.);
#9768=VECTOR('',#32810,1.);
#9769=VECTOR('',#32813,1.);
#9770=VECTOR('',#32814,1.);
#9771=VECTOR('',#32817,1.);
#9772=VECTOR('',#32820,1.);
#9773=VECTOR('',#32823,1.);
#9774=VECTOR('',#32824,1.);
#9775=VECTOR('',#32827,1.);
#9776=VECTOR('',#32828,1.);
#9777=VECTOR('',#32831,1.);
#9778=VECTOR('',#32834,1.);
#9779=VECTOR('',#32837,1.);
#9780=VECTOR('',#32838,1.);
#9781=VECTOR('',#32841,1.);
#9782=VECTOR('',#32842,1.);
#9783=VECTOR('',#32845,1.);
#9784=VECTOR('',#32848,1.);
#9785=VECTOR('',#32851,1.);
#9786=VECTOR('',#32852,1.);
#9787=VECTOR('',#32855,1.);
#9788=VECTOR('',#32856,1.);
#9789=VECTOR('',#32859,1.);
#9790=VECTOR('',#32862,1.);
#9791=VECTOR('',#32863,1.);
#9792=VECTOR('',#32866,1.);
#9793=VECTOR('',#32867,1.);
#9794=VECTOR('',#32870,1.);
#9795=VECTOR('',#32873,1.);
#9796=VECTOR('',#32876,1.);
#9797=VECTOR('',#32877,1.);
#9798=VECTOR('',#32878,1.);
#9799=VECTOR('',#32881,1.);
#9800=VECTOR('',#32882,1.);
#9801=VECTOR('',#32885,1.);
#9802=VECTOR('',#32886,1.);
#9803=VECTOR('',#32889,1.);
#9804=VECTOR('',#32890,1.);
#9805=VECTOR('',#32891,1.);
#9806=VECTOR('',#32892,1.);
#9807=VECTOR('',#32893,1.);
#9808=VECTOR('',#32894,1.);
#9809=VECTOR('',#32895,1.);
#9810=VECTOR('',#32896,1.);
#9811=VECTOR('',#32897,1.);
#9812=VECTOR('',#32898,1.);
#9813=VECTOR('',#32899,1.);
#9814=VECTOR('',#32900,1.);
#9815=VECTOR('',#32901,1.);
#9816=VECTOR('',#32902,1.);
#9817=VECTOR('',#32903,1.);
#9818=VECTOR('',#32904,1.);
#9819=VECTOR('',#32905,1.);
#9820=VECTOR('',#32906,1.);
#9821=VECTOR('',#32907,1.);
#9822=VECTOR('',#32908,1.);
#9823=VECTOR('',#32909,1.);
#9824=VECTOR('',#32910,1.);
#9825=VECTOR('',#32911,1.);
#9826=VECTOR('',#32912,1.);
#9827=VECTOR('',#32913,1.);
#9828=VECTOR('',#32914,1.);
#9829=VECTOR('',#32915,1.);
#9830=VECTOR('',#32916,1.);
#9831=VECTOR('',#32917,1.);
#9832=VECTOR('',#32918,1.);
#9833=VECTOR('',#32919,1.);
#9834=VECTOR('',#32920,1.);
#9835=VECTOR('',#32921,1.);
#9836=VECTOR('',#32922,1.);
#9837=VECTOR('',#32923,1.);
#9838=VECTOR('',#32924,1.);
#9839=VECTOR('',#32925,1.);
#9840=VECTOR('',#32926,1.);
#9841=VECTOR('',#32927,1.);
#9842=VECTOR('',#32928,1.);
#9843=VECTOR('',#32929,1.);
#9844=VECTOR('',#32930,1.);
#9845=VECTOR('',#32931,1.);
#9846=VECTOR('',#32932,1.);
#9847=VECTOR('',#32933,1.);
#9848=VECTOR('',#32934,1.);
#9849=VECTOR('',#32935,1.);
#9850=VECTOR('',#32936,1.);
#9851=VECTOR('',#32937,1.);
#9852=VECTOR('',#32938,1.);
#9853=VECTOR('',#32939,1.);
#9854=VECTOR('',#32940,1.);
#9855=VECTOR('',#32941,1.);
#9856=VECTOR('',#32942,1.);
#9857=VECTOR('',#32943,1.);
#9858=VECTOR('',#32944,1.);
#9859=VECTOR('',#32945,1.);
#9860=VECTOR('',#32946,1.);
#9861=VECTOR('',#32947,1.);
#9862=VECTOR('',#32948,1.);
#9863=VECTOR('',#32949,1.);
#9864=VECTOR('',#32950,1.);
#9865=VECTOR('',#32951,1.);
#9866=VECTOR('',#32952,1.);
#9867=VECTOR('',#32953,1.);
#9868=VECTOR('',#32954,1.);
#9869=VECTOR('',#32955,1.);
#9870=VECTOR('',#32956,1.);
#9871=VECTOR('',#32957,1.);
#9872=VECTOR('',#32958,1.);
#9873=VECTOR('',#32959,1.);
#9874=VECTOR('',#32960,1.);
#9875=VECTOR('',#32961,1.);
#9876=VECTOR('',#32962,1.);
#9877=VECTOR('',#32963,1.);
#9878=VECTOR('',#32964,1.);
#9879=VECTOR('',#32965,1.);
#9880=VECTOR('',#32966,1.);
#9881=VECTOR('',#32967,1.);
#9882=VECTOR('',#32968,1.);
#9883=VECTOR('',#32969,1.);
#9884=VECTOR('',#32970,1.);
#9885=VECTOR('',#32971,1.);
#9886=VECTOR('',#32972,1.);
#9887=VECTOR('',#32973,1.);
#9888=VECTOR('',#32974,1.);
#9889=VECTOR('',#32975,1.);
#9890=VECTOR('',#32976,1.);
#9891=VECTOR('',#32977,1.);
#9892=VECTOR('',#32978,1.);
#9893=VECTOR('',#32979,1.);
#9894=VECTOR('',#32980,1.);
#9895=VECTOR('',#32981,1.);
#9896=VECTOR('',#32982,1.);
#9897=VECTOR('',#32983,1.);
#9898=VECTOR('',#32984,1.);
#9899=VECTOR('',#32985,1.);
#9900=VECTOR('',#32986,1.);
#9901=VECTOR('',#32987,1.);
#9902=VECTOR('',#32988,1.);
#9903=VECTOR('',#32989,1.);
#9904=VECTOR('',#32990,1.);
#9905=VECTOR('',#32991,1.);
#9906=VECTOR('',#32992,1.);
#9907=VECTOR('',#32993,1.);
#9908=VECTOR('',#32994,1.);
#9909=VECTOR('',#32995,1.);
#9910=VECTOR('',#32996,1.);
#9911=VECTOR('',#32997,1.);
#9912=VECTOR('',#32998,1.);
#9913=VECTOR('',#32999,1.);
#9914=VECTOR('',#33000,1.);
#9915=VECTOR('',#33001,1.);
#9916=VECTOR('',#33002,1.);
#9917=VECTOR('',#33007,1.);
#9918=VECTOR('',#33010,1.);
#9919=VECTOR('',#33011,1.);
#9920=VECTOR('',#33014,1.);
#9921=VECTOR('',#33017,1.);
#9922=VECTOR('',#33022,1.);
#9923=VECTOR('',#33023,1.);
#9924=VECTOR('',#33026,1.);
#9925=VECTOR('',#33029,1.);
#9926=VECTOR('',#33034,1.);
#9927=VECTOR('',#33035,1.);
#9928=VECTOR('',#33038,1.);
#9929=VECTOR('',#33041,1.);
#9930=VECTOR('',#33046,1.);
#9931=VECTOR('',#33049,1.);
#9932=VECTOR('',#33052,1.);
#9933=VECTOR('',#33055,1.);
#9934=VECTOR('',#33056,1.);
#9935=VECTOR('',#33059,1.);
#9936=VECTOR('',#33062,1.);
#9937=VECTOR('',#33067,1.);
#9938=VECTOR('',#33068,1.);
#9939=VECTOR('',#33073,1.);
#9940=VECTOR('',#33076,1.);
#9941=VECTOR('',#33079,1.);
#9942=VECTOR('',#33080,1.);
#9943=VECTOR('',#33083,1.);
#9944=VECTOR('',#33086,1.);
#9945=VECTOR('',#33091,1.);
#9946=VECTOR('',#33092,1.);
#9947=VECTOR('',#33095,1.);
#9948=VECTOR('',#33098,1.);
#9949=VECTOR('',#33103,1.);
#9950=VECTOR('',#33104,1.);
#9951=VECTOR('',#33107,1.);
#9952=VECTOR('',#33110,1.);
#9953=VECTOR('',#33115,1.);
#9954=VECTOR('',#33116,1.);
#9955=VECTOR('',#33119,1.);
#9956=VECTOR('',#33122,1.);
#9957=VECTOR('',#33127,1.);
#9958=VECTOR('',#33128,1.);
#9959=VECTOR('',#33131,1.);
#9960=VECTOR('',#33134,1.);
#9961=VECTOR('',#33139,1.);
#9962=VECTOR('',#33140,1.);
#9963=VECTOR('',#33147,1.);
#9964=VECTOR('',#33148,1.);
#9965=VECTOR('',#33151,1.);
#9966=VECTOR('',#33154,1.);
#9967=VECTOR('',#33159,1.);
#9968=VECTOR('',#33160,1.);
#9969=VECTOR('',#33163,1.);
#9970=VECTOR('',#33166,1.);
#9971=VECTOR('',#33171,1.);
#9972=VECTOR('',#33174,1.);
#9973=VECTOR('',#33177,1.);
#9974=VECTOR('',#33180,1.);
#9975=VECTOR('',#33181,1.);
#9976=VECTOR('',#33184,1.);
#9977=VECTOR('',#33187,1.);
#9978=VECTOR('',#33192,1.);
#9979=VECTOR('',#33193,1.);
#9980=VECTOR('',#33196,1.);
#9981=VECTOR('',#33199,1.);
#9982=VECTOR('',#33204,1.);
#9983=VECTOR('',#33205,1.);
#9984=VECTOR('',#33208,1.);
#9985=VECTOR('',#33213,1.);
#9986=VECTOR('',#33216,1.);
#9987=VECTOR('',#33219,1.);
#9988=VECTOR('',#33220,1.);
#9989=VECTOR('',#33223,1.);
#9990=VECTOR('',#33226,1.);
#9991=VECTOR('',#33231,1.);
#9992=VECTOR('',#33232,1.);
#9993=VECTOR('',#33239,1.);
#9994=VECTOR('',#33240,1.);
#9995=VECTOR('',#33243,1.);
#9996=VECTOR('',#33246,1.);
#9997=VECTOR('',#33251,1.);
#9998=VECTOR('',#33252,1.);
#9999=VECTOR('',#33255,1.);
#10000=VECTOR('',#33258,1.);
#10001=VECTOR('',#33263,1.);
#10002=VECTOR('',#33266,1.);
#10003=VECTOR('',#33269,1.);
#10004=VECTOR('',#33272,1.);
#10005=VECTOR('',#33273,1.);
#10006=VECTOR('',#33276,1.);
#10007=VECTOR('',#33281,1.);
#10008=VECTOR('',#33284,1.);
#10009=VECTOR('',#33287,1.);
#10010=VECTOR('',#33288,1.);
#10011=VECTOR('',#33291,1.);
#10012=VECTOR('',#33294,1.);
#10013=VECTOR('',#33299,1.);
#10014=VECTOR('',#33300,1.);
#10015=VECTOR('',#33307,1.);
#10016=VECTOR('',#33308,1.);
#10017=VECTOR('',#33311,1.);
#10018=VECTOR('',#33312,1.);
#10019=VECTOR('',#33315,1.);
#10020=VECTOR('',#33318,1.);
#10021=VECTOR('',#33323,1.);
#10022=VECTOR('',#33324,1.);
#10023=VECTOR('',#33327,1.);
#10024=VECTOR('',#33332,1.);
#10025=VECTOR('',#33337,0.805);
#10026=VECTOR('',#33342,1.755);
#10027=VECTOR('',#33347,0.855000000000001);
#10028=VECTOR('',#33350,1.83);
#10029=VECTOR('',#33353,1.755);
#10030=VECTOR('',#33356,1.);
#10031=VECTOR('',#33357,1.);
#10032=VECTOR('',#33360,1.);
#10033=VECTOR('',#33363,1.);
#10034=VECTOR('',#33364,1.);
#10035=VECTOR('',#33379,1.);
#10036=VECTOR('',#33388,1.);
#10037=VECTOR('',#33389,1.);
#10038=VECTOR('',#33392,1.);
#10039=VECTOR('',#33395,1.);
#10876=CIRCLE('',#27911,1.905);
#10877=CIRCLE('',#28167,0.905000000000001);
#10878=CIRCLE('',#28279,0.805);
#10879=CIRCLE('',#28281,1.755);
#10880=CIRCLE('',#28282,1.755);
#12033=VERTEX_POINT('',#60848);
#12034=VERTEX_POINT('',#60849);
#12035=VERTEX_POINT('',#60851);
#12036=VERTEX_POINT('',#60853);
#12037=VERTEX_POINT('',#60855);
#12038=VERTEX_POINT('',#60857);
#12039=VERTEX_POINT('',#60861);
#12040=VERTEX_POINT('',#60863);
#12041=VERTEX_POINT('',#60865);
#12042=VERTEX_POINT('',#60869);
#12043=VERTEX_POINT('',#60873);
#12044=VERTEX_POINT('',#60875);
#12045=VERTEX_POINT('',#60879);
#12046=VERTEX_POINT('',#60880);
#12047=VERTEX_POINT('',#60882);
#12048=VERTEX_POINT('',#60884);
#12049=VERTEX_POINT('',#60886);
#12050=VERTEX_POINT('',#60888);
#12051=VERTEX_POINT('',#60892);
#12052=VERTEX_POINT('',#60894);
#12053=VERTEX_POINT('',#60896);
#12054=VERTEX_POINT('',#60900);
#12055=VERTEX_POINT('',#60904);
#12056=VERTEX_POINT('',#60906);
#12057=VERTEX_POINT('',#60910);
#12058=VERTEX_POINT('',#60911);
#12059=VERTEX_POINT('',#60913);
#12060=VERTEX_POINT('',#60915);
#12061=VERTEX_POINT('',#60917);
#12062=VERTEX_POINT('',#60919);
#12063=VERTEX_POINT('',#60923);
#12064=VERTEX_POINT('',#60925);
#12065=VERTEX_POINT('',#60929);
#12066=VERTEX_POINT('',#60931);
#12067=VERTEX_POINT('',#60935);
#12068=VERTEX_POINT('',#60937);
#12069=VERTEX_POINT('',#60939);
#12070=VERTEX_POINT('',#60943);
#12071=VERTEX_POINT('',#60944);
#12072=VERTEX_POINT('',#60946);
#12073=VERTEX_POINT('',#60948);
#12074=VERTEX_POINT('',#60950);
#12075=VERTEX_POINT('',#60952);
#12076=VERTEX_POINT('',#60956);
#12077=VERTEX_POINT('',#60958);
#12078=VERTEX_POINT('',#60960);
#12079=VERTEX_POINT('',#60964);
#12080=VERTEX_POINT('',#60968);
#12081=VERTEX_POINT('',#60970);
#12082=VERTEX_POINT('',#60974);
#12083=VERTEX_POINT('',#60975);
#12084=VERTEX_POINT('',#60977);
#12085=VERTEX_POINT('',#60979);
#12086=VERTEX_POINT('',#60981);
#12087=VERTEX_POINT('',#60983);
#12088=VERTEX_POINT('',#60987);
#12089=VERTEX_POINT('',#60989);
#12090=VERTEX_POINT('',#60993);
#12091=VERTEX_POINT('',#60995);
#12092=VERTEX_POINT('',#60997);
#12093=VERTEX_POINT('',#61001);
#12094=VERTEX_POINT('',#61003);
#12095=VERTEX_POINT('',#61007);
#12096=VERTEX_POINT('',#61008);
#12097=VERTEX_POINT('',#61010);
#12098=VERTEX_POINT('',#61012);
#12099=VERTEX_POINT('',#61014);
#12100=VERTEX_POINT('',#61016);
#12101=VERTEX_POINT('',#61020);
#12102=VERTEX_POINT('',#61022);
#12103=VERTEX_POINT('',#61024);
#12104=VERTEX_POINT('',#61028);
#12105=VERTEX_POINT('',#61030);
#12106=VERTEX_POINT('',#61032);
#12107=VERTEX_POINT('',#61036);
#12108=VERTEX_POINT('',#61040);
#12109=VERTEX_POINT('',#61042);
#12110=VERTEX_POINT('',#61044);
#12111=VERTEX_POINT('',#61048);
#12112=VERTEX_POINT('',#61050);
#12113=VERTEX_POINT('',#61054);
#12114=VERTEX_POINT('',#61055);
#12115=VERTEX_POINT('',#61057);
#12116=VERTEX_POINT('',#61059);
#12117=VERTEX_POINT('',#61061);
#12118=VERTEX_POINT('',#61063);
#12119=VERTEX_POINT('',#61067);
#12120=VERTEX_POINT('',#61069);
#12121=VERTEX_POINT('',#61073);
#12122=VERTEX_POINT('',#61075);
#12123=VERTEX_POINT('',#61082);
#12124=VERTEX_POINT('',#61083);
#12125=VERTEX_POINT('',#61085);
#12126=VERTEX_POINT('',#61087);
#12127=VERTEX_POINT('',#61089);
#12128=VERTEX_POINT('',#61091);
#12129=VERTEX_POINT('',#61095);
#12130=VERTEX_POINT('',#61097);
#12131=VERTEX_POINT('',#61101);
#12132=VERTEX_POINT('',#61103);
#12133=VERTEX_POINT('',#61105);
#12134=VERTEX_POINT('',#61109);
#12135=VERTEX_POINT('',#61111);
#12136=VERTEX_POINT('',#61115);
#12137=VERTEX_POINT('',#61116);
#12138=VERTEX_POINT('',#61118);
#12139=VERTEX_POINT('',#61120);
#12140=VERTEX_POINT('',#61122);
#12141=VERTEX_POINT('',#61124);
#12142=VERTEX_POINT('',#61128);
#12143=VERTEX_POINT('',#61130);
#12144=VERTEX_POINT('',#61132);
#12145=VERTEX_POINT('',#61136);
#12146=VERTEX_POINT('',#61138);
#12147=VERTEX_POINT('',#61140);
#12148=VERTEX_POINT('',#61144);
#12149=VERTEX_POINT('',#61148);
#12150=VERTEX_POINT('',#61150);
#12151=VERTEX_POINT('',#61152);
#12152=VERTEX_POINT('',#61156);
#12153=VERTEX_POINT('',#61158);
#12154=VERTEX_POINT('',#61162);
#12155=VERTEX_POINT('',#61163);
#12156=VERTEX_POINT('',#61165);
#12157=VERTEX_POINT('',#61167);
#12158=VERTEX_POINT('',#61169);
#12159=VERTEX_POINT('',#61171);
#12160=VERTEX_POINT('',#61175);
#12161=VERTEX_POINT('',#61177);
#12162=VERTEX_POINT('',#61181);
#12163=VERTEX_POINT('',#61183);
#12164=VERTEX_POINT('',#61190);
#12165=VERTEX_POINT('',#61191);
#12166=VERTEX_POINT('',#61193);
#12167=VERTEX_POINT('',#61195);
#12168=VERTEX_POINT('',#61197);
#12169=VERTEX_POINT('',#61199);
#12170=VERTEX_POINT('',#61203);
#12171=VERTEX_POINT('',#61205);
#12172=VERTEX_POINT('',#61207);
#12173=VERTEX_POINT('',#61211);
#12174=VERTEX_POINT('',#61213);
#12175=VERTEX_POINT('',#61215);
#12176=VERTEX_POINT('',#61219);
#12177=VERTEX_POINT('',#61223);
#12178=VERTEX_POINT('',#61225);
#12179=VERTEX_POINT('',#61227);
#12180=VERTEX_POINT('',#61231);
#12181=VERTEX_POINT('',#61233);
#12182=VERTEX_POINT('',#61237);
#12183=VERTEX_POINT('',#61238);
#12184=VERTEX_POINT('',#61240);
#12185=VERTEX_POINT('',#61242);
#12186=VERTEX_POINT('',#61244);
#12187=VERTEX_POINT('',#61246);
#12188=VERTEX_POINT('',#61250);
#12189=VERTEX_POINT('',#61252);
#12190=VERTEX_POINT('',#61256);
#12191=VERTEX_POINT('',#61258);
#12192=VERTEX_POINT('',#61262);
#12193=VERTEX_POINT('',#61264);
#12194=VERTEX_POINT('',#61266);
#12195=VERTEX_POINT('',#61270);
#12196=VERTEX_POINT('',#61272);
#12197=VERTEX_POINT('',#61274);
#12198=VERTEX_POINT('',#61276);
#12199=VERTEX_POINT('',#61280);
#12200=VERTEX_POINT('',#61282);
#12201=VERTEX_POINT('',#61286);
#12202=VERTEX_POINT('',#61288);
#12203=VERTEX_POINT('',#61292);
#12204=VERTEX_POINT('',#61297);
#12205=VERTEX_POINT('',#61298);
#12206=VERTEX_POINT('',#61300);
#12207=VERTEX_POINT('',#61302);
#12208=VERTEX_POINT('',#61304);
#12209=VERTEX_POINT('',#61306);
#12210=VERTEX_POINT('',#61310);
#12211=VERTEX_POINT('',#61312);
#12212=VERTEX_POINT('',#61314);
#12213=VERTEX_POINT('',#61318);
#12214=VERTEX_POINT('',#61320);
#12215=VERTEX_POINT('',#61322);
#12216=VERTEX_POINT('',#61326);
#12217=VERTEX_POINT('',#61330);
#12218=VERTEX_POINT('',#61332);
#12219=VERTEX_POINT('',#61334);
#12220=VERTEX_POINT('',#61338);
#12221=VERTEX_POINT('',#61340);
#12222=VERTEX_POINT('',#61344);
#12223=VERTEX_POINT('',#61345);
#12224=VERTEX_POINT('',#61347);
#12225=VERTEX_POINT('',#61349);
#12226=VERTEX_POINT('',#61351);
#12227=VERTEX_POINT('',#61353);
#12228=VERTEX_POINT('',#61357);
#12229=VERTEX_POINT('',#61359);
#12230=VERTEX_POINT('',#61361);
#12231=VERTEX_POINT('',#61365);
#12232=VERTEX_POINT('',#61367);
#12233=VERTEX_POINT('',#61369);
#12234=VERTEX_POINT('',#61373);
#12235=VERTEX_POINT('',#61377);
#12236=VERTEX_POINT('',#61379);
#12237=VERTEX_POINT('',#61381);
#12238=VERTEX_POINT('',#61385);
#12239=VERTEX_POINT('',#61387);
#12240=VERTEX_POINT('',#61391);
#12241=VERTEX_POINT('',#61392);
#12242=VERTEX_POINT('',#61394);
#12243=VERTEX_POINT('',#61396);
#12244=VERTEX_POINT('',#61398);
#12245=VERTEX_POINT('',#61400);
#12246=VERTEX_POINT('',#61404);
#12247=VERTEX_POINT('',#61406);
#12248=VERTEX_POINT('',#61408);
#12249=VERTEX_POINT('',#61412);
#12250=VERTEX_POINT('',#61416);
#12251=VERTEX_POINT('',#61418);
#12252=VERTEX_POINT('',#61422);
#12253=VERTEX_POINT('',#61423);
#12254=VERTEX_POINT('',#61425);
#12255=VERTEX_POINT('',#61427);
#12256=VERTEX_POINT('',#61429);
#12257=VERTEX_POINT('',#61431);
#12258=VERTEX_POINT('',#61435);
#12259=VERTEX_POINT('',#61437);
#12260=VERTEX_POINT('',#61439);
#12261=VERTEX_POINT('',#61443);
#12262=VERTEX_POINT('',#61445);
#12263=VERTEX_POINT('',#61447);
#12264=VERTEX_POINT('',#61451);
#12265=VERTEX_POINT('',#61455);
#12266=VERTEX_POINT('',#61457);
#12267=VERTEX_POINT('',#61459);
#12268=VERTEX_POINT('',#61463);
#12269=VERTEX_POINT('',#61465);
#12270=VERTEX_POINT('',#61469);
#12271=VERTEX_POINT('',#61470);
#12272=VERTEX_POINT('',#61472);
#12273=VERTEX_POINT('',#61474);
#12274=VERTEX_POINT('',#61476);
#12275=VERTEX_POINT('',#61478);
#12276=VERTEX_POINT('',#61482);
#12277=VERTEX_POINT('',#61484);
#12278=VERTEX_POINT('',#61486);
#12279=VERTEX_POINT('',#61490);
#12280=VERTEX_POINT('',#61492);
#12281=VERTEX_POINT('',#61494);
#12282=VERTEX_POINT('',#61498);
#12283=VERTEX_POINT('',#61502);
#12284=VERTEX_POINT('',#61504);
#12285=VERTEX_POINT('',#61506);
#12286=VERTEX_POINT('',#61510);
#12287=VERTEX_POINT('',#61512);
#12288=VERTEX_POINT('',#61516);
#12289=VERTEX_POINT('',#61518);
#12290=VERTEX_POINT('',#61520);
#12291=VERTEX_POINT('',#61522);
#12292=VERTEX_POINT('',#61526);
#12293=VERTEX_POINT('',#61528);
#12294=VERTEX_POINT('',#61532);
#12295=VERTEX_POINT('',#61536);
#12296=VERTEX_POINT('',#61538);
#12297=VERTEX_POINT('',#61542);
#12298=VERTEX_POINT('',#61543);
#12299=VERTEX_POINT('',#61545);
#12300=VERTEX_POINT('',#61547);
#12301=VERTEX_POINT('',#61551);
#12302=VERTEX_POINT('',#61553);
#12303=VERTEX_POINT('',#61556);
#12304=VERTEX_POINT('',#61559);
#12305=VERTEX_POINT('',#61561);
#12306=VERTEX_POINT('',#61563);
#12307=VERTEX_POINT('',#61567);
#12308=VERTEX_POINT('',#61568);
#12309=VERTEX_POINT('',#61571);
#12310=VERTEX_POINT('',#61573);
#12311=VERTEX_POINT('',#61575);
#12312=VERTEX_POINT('',#61579);
#12313=VERTEX_POINT('',#61583);
#12314=VERTEX_POINT('',#61585);
#12315=VERTEX_POINT('',#61587);
#12316=VERTEX_POINT('',#61589);
#12317=VERTEX_POINT('',#61593);
#12318=VERTEX_POINT('',#61595);
#12319=VERTEX_POINT('',#61597);
#12320=VERTEX_POINT('',#61603);
#12321=VERTEX_POINT('',#61604);
#12322=VERTEX_POINT('',#61606);
#12323=VERTEX_POINT('',#61608);
#12324=VERTEX_POINT('',#61610);
#12325=VERTEX_POINT('',#61612);
#12326=VERTEX_POINT('',#61616);
#12327=VERTEX_POINT('',#61619);
#12328=VERTEX_POINT('',#61623);
#12329=VERTEX_POINT('',#61625);
#12330=VERTEX_POINT('',#61627);
#12331=VERTEX_POINT('',#61631);
#12332=VERTEX_POINT('',#61635);
#12333=VERTEX_POINT('',#61636);
#12334=VERTEX_POINT('',#61638);
#12335=VERTEX_POINT('',#61640);
#12336=VERTEX_POINT('',#61642);
#12337=VERTEX_POINT('',#61644);
#12338=VERTEX_POINT('',#61648);
#12339=VERTEX_POINT('',#61650);
#12340=VERTEX_POINT('',#61652);
#12341=VERTEX_POINT('',#61656);
#12342=VERTEX_POINT('',#61658);
#12343=VERTEX_POINT('',#61660);
#12344=VERTEX_POINT('',#61664);
#12345=VERTEX_POINT('',#61668);
#12346=VERTEX_POINT('',#61670);
#12347=VERTEX_POINT('',#61672);
#12348=VERTEX_POINT('',#61676);
#12349=VERTEX_POINT('',#61678);
#12350=VERTEX_POINT('',#61682);
#12351=VERTEX_POINT('',#61683);
#12352=VERTEX_POINT('',#61685);
#12353=VERTEX_POINT('',#61687);
#12354=VERTEX_POINT('',#61689);
#12355=VERTEX_POINT('',#61691);
#12356=VERTEX_POINT('',#61695);
#12357=VERTEX_POINT('',#61697);
#12358=VERTEX_POINT('',#61699);
#12359=VERTEX_POINT('',#61703);
#12360=VERTEX_POINT('',#61705);
#12361=VERTEX_POINT('',#61707);
#12362=VERTEX_POINT('',#61711);
#12363=VERTEX_POINT('',#61715);
#12364=VERTEX_POINT('',#61717);
#12365=VERTEX_POINT('',#61719);
#12366=VERTEX_POINT('',#61723);
#12367=VERTEX_POINT('',#61725);
#12368=VERTEX_POINT('',#61729);
#12369=VERTEX_POINT('',#61730);
#12370=VERTEX_POINT('',#61732);
#12371=VERTEX_POINT('',#61734);
#12372=VERTEX_POINT('',#61736);
#12373=VERTEX_POINT('',#61738);
#12374=VERTEX_POINT('',#61742);
#12375=VERTEX_POINT('',#61744);
#12376=VERTEX_POINT('',#61746);
#12377=VERTEX_POINT('',#61750);
#12378=VERTEX_POINT('',#61752);
#12379=VERTEX_POINT('',#61754);
#12380=VERTEX_POINT('',#61758);
#12381=VERTEX_POINT('',#61762);
#12382=VERTEX_POINT('',#61764);
#12383=VERTEX_POINT('',#61766);
#12384=VERTEX_POINT('',#61770);
#12385=VERTEX_POINT('',#61772);
#12386=VERTEX_POINT('',#61776);
#12387=VERTEX_POINT('',#61777);
#12388=VERTEX_POINT('',#61779);
#12389=VERTEX_POINT('',#61781);
#12390=VERTEX_POINT('',#61783);
#12391=VERTEX_POINT('',#61785);
#12392=VERTEX_POINT('',#61789);
#12393=VERTEX_POINT('',#61791);
#12394=VERTEX_POINT('',#61793);
#12395=VERTEX_POINT('',#61797);
#12396=VERTEX_POINT('',#61799);
#12397=VERTEX_POINT('',#61801);
#12398=VERTEX_POINT('',#61805);
#12399=VERTEX_POINT('',#61809);
#12400=VERTEX_POINT('',#61811);
#12401=VERTEX_POINT('',#61813);
#12402=VERTEX_POINT('',#61817);
#12403=VERTEX_POINT('',#61819);
#12404=VERTEX_POINT('',#61823);
#12405=VERTEX_POINT('',#61824);
#12406=VERTEX_POINT('',#61826);
#12407=VERTEX_POINT('',#61828);
#12408=VERTEX_POINT('',#61830);
#12409=VERTEX_POINT('',#61832);
#12410=VERTEX_POINT('',#61836);
#12411=VERTEX_POINT('',#61838);
#12412=VERTEX_POINT('',#61842);
#12413=VERTEX_POINT('',#61844);
#12414=VERTEX_POINT('',#61854);
#12415=VERTEX_POINT('',#61863);
#12416=VERTEX_POINT('',#61867);
#12417=VERTEX_POINT('',#61876);
#12418=VERTEX_POINT('',#61882);
#12419=VERTEX_POINT('',#61884);
#12420=VERTEX_POINT('',#61886);
#12421=VERTEX_POINT('',#61888);
#12422=VERTEX_POINT('',#61890);
#12423=VERTEX_POINT('',#61892);
#12424=VERTEX_POINT('',#61894);
#12425=VERTEX_POINT('',#61896);
#12426=VERTEX_POINT('',#61898);
#12427=VERTEX_POINT('',#61900);
#12428=VERTEX_POINT('',#61902);
#12429=VERTEX_POINT('',#61904);
#12430=VERTEX_POINT('',#61906);
#12431=VERTEX_POINT('',#61908);
#12432=VERTEX_POINT('',#61910);
#12433=VERTEX_POINT('',#61912);
#12434=VERTEX_POINT('',#61914);
#12435=VERTEX_POINT('',#61916);
#12436=VERTEX_POINT('',#61918);
#12437=VERTEX_POINT('',#61920);
#12438=VERTEX_POINT('',#61922);
#12439=VERTEX_POINT('',#61924);
#12440=VERTEX_POINT('',#61926);
#12441=VERTEX_POINT('',#61928);
#12442=VERTEX_POINT('',#61930);
#12443=VERTEX_POINT('',#61932);
#12444=VERTEX_POINT('',#61934);
#12445=VERTEX_POINT('',#61939);
#12446=VERTEX_POINT('',#61941);
#12447=VERTEX_POINT('',#61943);
#12448=VERTEX_POINT('',#61945);
#12449=VERTEX_POINT('',#61947);
#12450=VERTEX_POINT('',#61949);
#12451=VERTEX_POINT('',#61951);
#12452=VERTEX_POINT('',#61953);
#12453=VERTEX_POINT('',#61955);
#12454=VERTEX_POINT('',#61957);
#12455=VERTEX_POINT('',#61959);
#12456=VERTEX_POINT('',#61961);
#12457=VERTEX_POINT('',#61963);
#12458=VERTEX_POINT('',#61965);
#12459=VERTEX_POINT('',#61967);
#12460=VERTEX_POINT('',#61969);
#12461=VERTEX_POINT('',#61971);
#12462=VERTEX_POINT('',#61973);
#12463=VERTEX_POINT('',#61975);
#12464=VERTEX_POINT('',#61977);
#12465=VERTEX_POINT('',#61979);
#12466=VERTEX_POINT('',#61981);
#12467=VERTEX_POINT('',#61983);
#12468=VERTEX_POINT('',#61985);
#12469=VERTEX_POINT('',#61987);
#12470=VERTEX_POINT('',#61994);
#12471=VERTEX_POINT('',#62000);
#12472=VERTEX_POINT('',#62002);
#12473=VERTEX_POINT('',#62004);
#12474=VERTEX_POINT('',#62006);
#12475=VERTEX_POINT('',#62008);
#12476=VERTEX_POINT('',#62018);
#12477=VERTEX_POINT('',#62026);
#12478=VERTEX_POINT('',#62030);
#12479=VERTEX_POINT('',#62038);
#12480=VERTEX_POINT('',#62042);
#12481=VERTEX_POINT('',#62050);
#12482=VERTEX_POINT('',#62054);
#12483=VERTEX_POINT('',#62060);
#12484=VERTEX_POINT('',#62064);
#12485=VERTEX_POINT('',#62068);
#12486=VERTEX_POINT('',#62072);
#12487=VERTEX_POINT('',#62073);
#12488=VERTEX_POINT('',#62075);
#12489=VERTEX_POINT('',#62077);
#12490=VERTEX_POINT('',#62081);
#12491=VERTEX_POINT('',#62084);
#12492=VERTEX_POINT('',#62091);
#12493=VERTEX_POINT('',#62093);
#12494=VERTEX_POINT('',#62097);
#12495=VERTEX_POINT('',#62099);
#12496=VERTEX_POINT('',#62103);
#12497=VERTEX_POINT('',#62108);
#12498=VERTEX_POINT('',#62110);
#12499=VERTEX_POINT('',#62112);
#12500=VERTEX_POINT('',#62116);
#12501=VERTEX_POINT('',#62120);
#12502=VERTEX_POINT('',#62121);
#12503=VERTEX_POINT('',#62123);
#12504=VERTEX_POINT('',#62125);
#12505=VERTEX_POINT('',#62127);
#12506=VERTEX_POINT('',#62129);
#12507=VERTEX_POINT('',#62134);
#12508=VERTEX_POINT('',#62138);
#12509=VERTEX_POINT('',#62140);
#12510=VERTEX_POINT('',#62144);
#12511=VERTEX_POINT('',#62148);
#12512=VERTEX_POINT('',#62150);
#12513=VERTEX_POINT('',#62152);
#12514=VERTEX_POINT('',#62162);
#12515=VERTEX_POINT('',#62166);
#12516=VERTEX_POINT('',#62174);
#12517=VERTEX_POINT('',#62182);
#12518=VERTEX_POINT('',#62186);
#12519=VERTEX_POINT('',#62196);
#12520=VERTEX_POINT('',#62204);
#12521=VERTEX_POINT('',#62212);
#12522=VERTEX_POINT('',#62220);
#12523=VERTEX_POINT('',#62228);
#12524=VERTEX_POINT('',#62232);
#12525=VERTEX_POINT('',#62238);
#12526=VERTEX_POINT('',#62239);
#12527=VERTEX_POINT('',#62241);
#12528=VERTEX_POINT('',#62243);
#12529=VERTEX_POINT('',#62245);
#12530=VERTEX_POINT('',#62247);
#12531=VERTEX_POINT('',#62252);
#12532=VERTEX_POINT('',#62256);
#12533=VERTEX_POINT('',#62258);
#12534=VERTEX_POINT('',#62262);
#12535=VERTEX_POINT('',#62266);
#12536=VERTEX_POINT('',#62268);
#12537=VERTEX_POINT('',#62270);
#12538=VERTEX_POINT('',#62274);
#12539=VERTEX_POINT('',#62278);
#12540=VERTEX_POINT('',#62279);
#12541=VERTEX_POINT('',#62281);
#12542=VERTEX_POINT('',#62283);
#12543=VERTEX_POINT('',#62285);
#12544=VERTEX_POINT('',#62287);
#12545=VERTEX_POINT('',#62292);
#12546=VERTEX_POINT('',#62296);
#12547=VERTEX_POINT('',#62298);
#12548=VERTEX_POINT('',#62302);
#12549=VERTEX_POINT('',#62306);
#12550=VERTEX_POINT('',#62308);
#12551=VERTEX_POINT('',#62310);
#12552=VERTEX_POINT('',#62314);
#12553=VERTEX_POINT('',#62318);
#12554=VERTEX_POINT('',#62319);
#12555=VERTEX_POINT('',#62321);
#12556=VERTEX_POINT('',#62323);
#12557=VERTEX_POINT('',#62325);
#12558=VERTEX_POINT('',#62327);
#12559=VERTEX_POINT('',#62332);
#12560=VERTEX_POINT('',#62336);
#12561=VERTEX_POINT('',#62338);
#12562=VERTEX_POINT('',#62342);
#12563=VERTEX_POINT('',#62346);
#12564=VERTEX_POINT('',#62348);
#12565=VERTEX_POINT('',#62350);
#12566=VERTEX_POINT('',#62354);
#12567=VERTEX_POINT('',#62358);
#12568=VERTEX_POINT('',#62359);
#12569=VERTEX_POINT('',#62361);
#12570=VERTEX_POINT('',#62363);
#12571=VERTEX_POINT('',#62365);
#12572=VERTEX_POINT('',#62367);
#12573=VERTEX_POINT('',#62371);
#12574=VERTEX_POINT('',#62373);
#12575=VERTEX_POINT('',#62380);
#12576=VERTEX_POINT('',#62382);
#12577=VERTEX_POINT('',#62386);
#12578=VERTEX_POINT('',#62388);
#12579=VERTEX_POINT('',#62390);
#12580=VERTEX_POINT('',#62392);
#12581=VERTEX_POINT('',#62396);
#12582=VERTEX_POINT('',#62398);
#12583=VERTEX_POINT('',#62402);
#12584=VERTEX_POINT('',#62404);
#12585=VERTEX_POINT('',#62408);
#12586=VERTEX_POINT('',#62413);
#12587=VERTEX_POINT('',#62414);
#12588=VERTEX_POINT('',#62416);
#12589=VERTEX_POINT('',#62418);
#12590=VERTEX_POINT('',#62420);
#12591=VERTEX_POINT('',#62422);
#12592=VERTEX_POINT('',#62427);
#12593=VERTEX_POINT('',#62431);
#12594=VERTEX_POINT('',#62433);
#12595=VERTEX_POINT('',#62437);
#12596=VERTEX_POINT('',#62441);
#12597=VERTEX_POINT('',#62443);
#12598=VERTEX_POINT('',#62445);
#12599=VERTEX_POINT('',#62449);
#12600=VERTEX_POINT('',#62453);
#12601=VERTEX_POINT('',#62454);
#12602=VERTEX_POINT('',#62456);
#12603=VERTEX_POINT('',#62458);
#12604=VERTEX_POINT('',#62460);
#12605=VERTEX_POINT('',#62462);
#12606=VERTEX_POINT('',#62467);
#12607=VERTEX_POINT('',#62471);
#12608=VERTEX_POINT('',#62473);
#12609=VERTEX_POINT('',#62477);
#12610=VERTEX_POINT('',#62481);
#12611=VERTEX_POINT('',#62483);
#12612=VERTEX_POINT('',#62485);
#12613=VERTEX_POINT('',#62489);
#12614=VERTEX_POINT('',#62493);
#12615=VERTEX_POINT('',#62495);
#12616=VERTEX_POINT('',#62497);
#12617=VERTEX_POINT('',#62501);
#12618=VERTEX_POINT('',#62503);
#12619=VERTEX_POINT('',#62505);
#12620=VERTEX_POINT('',#62509);
#12621=VERTEX_POINT('',#62517);
#12622=VERTEX_POINT('',#62525);
#12623=VERTEX_POINT('',#62529);
#12624=VERTEX_POINT('',#62539);
#12625=VERTEX_POINT('',#62547);
#12626=VERTEX_POINT('',#62555);
#12627=VERTEX_POINT('',#62559);
#12628=VERTEX_POINT('',#62567);
#12629=VERTEX_POINT('',#62571);
#12630=VERTEX_POINT('',#62579);
#12631=VERTEX_POINT('',#62587);
#12632=VERTEX_POINT('',#62595);
#12633=VERTEX_POINT('',#62599);
#12634=VERTEX_POINT('',#62605);
#12635=VERTEX_POINT('',#62606);
#12636=VERTEX_POINT('',#62608);
#12637=VERTEX_POINT('',#62610);
#12638=VERTEX_POINT('',#62612);
#12639=VERTEX_POINT('',#62614);
#12640=VERTEX_POINT('',#62619);
#12641=VERTEX_POINT('',#62623);
#12642=VERTEX_POINT('',#62625);
#12643=VERTEX_POINT('',#62629);
#12644=VERTEX_POINT('',#62633);
#12645=VERTEX_POINT('',#62635);
#12646=VERTEX_POINT('',#62637);
#12647=VERTEX_POINT('',#62641);
#12648=VERTEX_POINT('',#62645);
#12649=VERTEX_POINT('',#62646);
#12650=VERTEX_POINT('',#62648);
#12651=VERTEX_POINT('',#62650);
#12652=VERTEX_POINT('',#62652);
#12653=VERTEX_POINT('',#62654);
#12654=VERTEX_POINT('',#62659);
#12655=VERTEX_POINT('',#62663);
#12656=VERTEX_POINT('',#62665);
#12657=VERTEX_POINT('',#62669);
#12658=VERTEX_POINT('',#62673);
#12659=VERTEX_POINT('',#62675);
#12660=VERTEX_POINT('',#62677);
#12661=VERTEX_POINT('',#62681);
#12662=VERTEX_POINT('',#62685);
#12663=VERTEX_POINT('',#62686);
#12664=VERTEX_POINT('',#62688);
#12665=VERTEX_POINT('',#62690);
#12666=VERTEX_POINT('',#62692);
#12667=VERTEX_POINT('',#62694);
#12668=VERTEX_POINT('',#62699);
#12669=VERTEX_POINT('',#62703);
#12670=VERTEX_POINT('',#62705);
#12671=VERTEX_POINT('',#62709);
#12672=VERTEX_POINT('',#62713);
#12673=VERTEX_POINT('',#62715);
#12674=VERTEX_POINT('',#62717);
#12675=VERTEX_POINT('',#62721);
#12676=VERTEX_POINT('',#62725);
#12677=VERTEX_POINT('',#62726);
#12678=VERTEX_POINT('',#62728);
#12679=VERTEX_POINT('',#62730);
#12680=VERTEX_POINT('',#62732);
#12681=VERTEX_POINT('',#62734);
#12682=VERTEX_POINT('',#62739);
#12683=VERTEX_POINT('',#62743);
#12684=VERTEX_POINT('',#62745);
#12685=VERTEX_POINT('',#62749);
#12686=VERTEX_POINT('',#62753);
#12687=VERTEX_POINT('',#62755);
#12688=VERTEX_POINT('',#62757);
#12689=VERTEX_POINT('',#62761);
#12690=VERTEX_POINT('',#62765);
#12691=VERTEX_POINT('',#62766);
#12692=VERTEX_POINT('',#62768);
#12693=VERTEX_POINT('',#62770);
#12694=VERTEX_POINT('',#62772);
#12695=VERTEX_POINT('',#62774);
#12696=VERTEX_POINT('',#62779);
#12697=VERTEX_POINT('',#62783);
#12698=VERTEX_POINT('',#62785);
#12699=VERTEX_POINT('',#62789);
#12700=VERTEX_POINT('',#62793);
#12701=VERTEX_POINT('',#62795);
#12702=VERTEX_POINT('',#62797);
#12703=VERTEX_POINT('',#62801);
#12704=VERTEX_POINT('',#62805);
#12705=VERTEX_POINT('',#62806);
#12706=VERTEX_POINT('',#62808);
#12707=VERTEX_POINT('',#62810);
#12708=VERTEX_POINT('',#62812);
#12709=VERTEX_POINT('',#62814);
#12710=VERTEX_POINT('',#62819);
#12711=VERTEX_POINT('',#62823);
#12712=VERTEX_POINT('',#62825);
#12713=VERTEX_POINT('',#62829);
#12714=VERTEX_POINT('',#62833);
#12715=VERTEX_POINT('',#62835);
#12716=VERTEX_POINT('',#62837);
#12717=VERTEX_POINT('',#62841);
#12718=VERTEX_POINT('',#62845);
#12719=VERTEX_POINT('',#62847);
#12720=VERTEX_POINT('',#62849);
#12721=VERTEX_POINT('',#62853);
#12722=VERTEX_POINT('',#62855);
#12723=VERTEX_POINT('',#62857);
#12724=VERTEX_POINT('',#62861);
#12725=VERTEX_POINT('',#62869);
#12726=VERTEX_POINT('',#62877);
#12727=VERTEX_POINT('',#62881);
#12728=VERTEX_POINT('',#62889);
#12729=VERTEX_POINT('',#62893);
#12730=VERTEX_POINT('',#62901);
#12731=VERTEX_POINT('',#62905);
#12732=VERTEX_POINT('',#62913);
#12733=VERTEX_POINT('',#62917);
#12734=VERTEX_POINT('',#62925);
#12735=VERTEX_POINT('',#62929);
#12736=VERTEX_POINT('',#62938);
#12737=VERTEX_POINT('',#62946);
#12738=VERTEX_POINT('',#62948);
#12739=VERTEX_POINT('',#62952);
#12740=VERTEX_POINT('',#62956);
#12741=VERTEX_POINT('',#62960);
#12742=VERTEX_POINT('',#62962);
#12743=VERTEX_POINT('',#62964);
#12744=VERTEX_POINT('',#62966);
#12745=VERTEX_POINT('',#62968);
#12746=VERTEX_POINT('',#62970);
#12747=VERTEX_POINT('',#62972);
#12748=VERTEX_POINT('',#62974);
#12749=VERTEX_POINT('',#62977);
#12750=VERTEX_POINT('',#62980);
#12751=VERTEX_POINT('',#62982);
#12752=VERTEX_POINT('',#62984);
#12753=VERTEX_POINT('',#62986);
#12754=VERTEX_POINT('',#62988);
#12755=VERTEX_POINT('',#62990);
#12756=VERTEX_POINT('',#62992);
#12757=VERTEX_POINT('',#62994);
#12758=VERTEX_POINT('',#62997);
#12759=VERTEX_POINT('',#62999);
#12760=VERTEX_POINT('',#63001);
#12761=VERTEX_POINT('',#63003);
#12762=VERTEX_POINT('',#63005);
#12763=VERTEX_POINT('',#63008);
#12764=VERTEX_POINT('',#63010);
#12765=VERTEX_POINT('',#63012);
#12766=VERTEX_POINT('',#63014);
#12767=VERTEX_POINT('',#63016);
#12768=VERTEX_POINT('',#63018);
#12769=VERTEX_POINT('',#63020);
#12770=VERTEX_POINT('',#63022);
#12771=VERTEX_POINT('',#63025);
#12772=VERTEX_POINT('',#63027);
#12773=VERTEX_POINT('',#63029);
#12774=VERTEX_POINT('',#63031);
#12775=VERTEX_POINT('',#63033);
#12776=VERTEX_POINT('',#63035);
#12777=VERTEX_POINT('',#63037);
#12778=VERTEX_POINT('',#63039);
#12779=VERTEX_POINT('',#63042);
#12780=VERTEX_POINT('',#63044);
#12781=VERTEX_POINT('',#63046);
#12782=VERTEX_POINT('',#63048);
#12783=VERTEX_POINT('',#63050);
#12784=VERTEX_POINT('',#63052);
#12785=VERTEX_POINT('',#63054);
#12786=VERTEX_POINT('',#63056);
#12787=VERTEX_POINT('',#63058);
#12788=VERTEX_POINT('',#63060);
#12789=VERTEX_POINT('',#63062);
#12790=VERTEX_POINT('',#63064);
#12791=VERTEX_POINT('',#63066);
#12792=VERTEX_POINT('',#63069);
#12793=VERTEX_POINT('',#63071);
#12794=VERTEX_POINT('',#63073);
#12795=VERTEX_POINT('',#63075);
#12796=VERTEX_POINT('',#63077);
#12797=VERTEX_POINT('',#63079);
#12798=VERTEX_POINT('',#63081);
#12799=VERTEX_POINT('',#63083);
#12800=VERTEX_POINT('',#63086);
#12801=VERTEX_POINT('',#63088);
#12802=VERTEX_POINT('',#63090);
#12803=VERTEX_POINT('',#63092);
#12804=VERTEX_POINT('',#63094);
#12805=VERTEX_POINT('',#63096);
#12806=VERTEX_POINT('',#63098);
#12807=VERTEX_POINT('',#63100);
#12808=VERTEX_POINT('',#63102);
#12809=VERTEX_POINT('',#63104);
#12810=VERTEX_POINT('',#63106);
#12811=VERTEX_POINT('',#63108);
#12812=VERTEX_POINT('',#63110);
#12813=VERTEX_POINT('',#63112);
#12814=VERTEX_POINT('',#63114);
#12815=VERTEX_POINT('',#63116);
#12816=VERTEX_POINT('',#63118);
#12817=VERTEX_POINT('',#63120);
#12818=VERTEX_POINT('',#63122);
#12819=VERTEX_POINT('',#63124);
#12820=VERTEX_POINT('',#63126);
#12821=VERTEX_POINT('',#63128);
#12822=VERTEX_POINT('',#63130);
#12823=VERTEX_POINT('',#63132);
#12824=VERTEX_POINT('',#63135);
#12825=VERTEX_POINT('',#63137);
#12826=VERTEX_POINT('',#63139);
#12827=VERTEX_POINT('',#63141);
#12828=VERTEX_POINT('',#63143);
#12829=VERTEX_POINT('',#63145);
#12830=VERTEX_POINT('',#63147);
#12831=VERTEX_POINT('',#63149);
#12832=VERTEX_POINT('',#63152);
#12833=VERTEX_POINT('',#63154);
#12834=VERTEX_POINT('',#63156);
#12835=VERTEX_POINT('',#63158);
#12836=VERTEX_POINT('',#63160);
#12837=VERTEX_POINT('',#63162);
#12838=VERTEX_POINT('',#63164);
#12839=VERTEX_POINT('',#63166);
#12840=VERTEX_POINT('',#63168);
#12841=VERTEX_POINT('',#63170);
#12842=VERTEX_POINT('',#63172);
#12843=VERTEX_POINT('',#63174);
#12844=VERTEX_POINT('',#63177);
#12845=VERTEX_POINT('',#63379);
#12846=VERTEX_POINT('',#63557);
#12847=VERTEX_POINT('',#63558);
#12848=VERTEX_POINT('',#63560);
#12849=VERTEX_POINT('',#63646);
#12850=VERTEX_POINT('',#63650);
#12851=VERTEX_POINT('',#63652);
#12852=VERTEX_POINT('',#63660);
#12853=VERTEX_POINT('',#63663);
#12854=VERTEX_POINT('',#63669);
#12855=VERTEX_POINT('',#63684);
#15023=EDGE_CURVE('',#12033,#12034,#6249,.T.);
#15024=EDGE_CURVE('',#12034,#12035,#6250,.T.);
#15025=EDGE_CURVE('',#12035,#12036,#6251,.T.);
#15026=EDGE_CURVE('',#12036,#12037,#6252,.T.);
#15027=EDGE_CURVE('',#12037,#12038,#6253,.T.);
#15028=EDGE_CURVE('',#12038,#12033,#6254,.T.);
#15029=EDGE_CURVE('',#12038,#12039,#6255,.T.);
#15030=EDGE_CURVE('',#12040,#12039,#6256,.F.);
#15031=EDGE_CURVE('',#12040,#12041,#6257,.T.);
#15032=EDGE_CURVE('',#12041,#12033,#6258,.T.);
#15033=EDGE_CURVE('',#12042,#12037,#6259,.T.);
#15034=EDGE_CURVE('',#12042,#12039,#6260,.T.);
#15035=EDGE_CURVE('',#12036,#12043,#6261,.T.);
#15036=EDGE_CURVE('',#12043,#12044,#6262,.T.);
#15037=EDGE_CURVE('',#12044,#12042,#6263,.T.);
#15038=EDGE_CURVE('',#12045,#12046,#6264,.T.);
#15039=EDGE_CURVE('',#12046,#12047,#6265,.T.);
#15040=EDGE_CURVE('',#12047,#12048,#6266,.T.);
#15041=EDGE_CURVE('',#12048,#12049,#6267,.T.);
#15042=EDGE_CURVE('',#12049,#12050,#6268,.T.);
#15043=EDGE_CURVE('',#12050,#12045,#6269,.T.);
#15044=EDGE_CURVE('',#12050,#12051,#6270,.T.);
#15045=EDGE_CURVE('',#12052,#12051,#6271,.F.);
#15046=EDGE_CURVE('',#12052,#12053,#6272,.T.);
#15047=EDGE_CURVE('',#12053,#12045,#6273,.T.);
#15048=EDGE_CURVE('',#12054,#12049,#6274,.T.);
#15049=EDGE_CURVE('',#12054,#12051,#6275,.T.);
#15050=EDGE_CURVE('',#12048,#12055,#6276,.T.);
#15051=EDGE_CURVE('',#12055,#12056,#6277,.T.);
#15052=EDGE_CURVE('',#12056,#12054,#6278,.T.);
#15053=EDGE_CURVE('',#12057,#12058,#6279,.T.);
#15054=EDGE_CURVE('',#12058,#12059,#6280,.T.);
#15055=EDGE_CURVE('',#12059,#12060,#6281,.T.);
#15056=EDGE_CURVE('',#12060,#12061,#6282,.T.);
#15057=EDGE_CURVE('',#12061,#12062,#6283,.T.);
#15058=EDGE_CURVE('',#12062,#12057,#6284,.T.);
#15059=EDGE_CURVE('',#12063,#12061,#6285,.T.);
#15060=EDGE_CURVE('',#12063,#12064,#6286,.T.);
#15061=EDGE_CURVE('',#12062,#12064,#6287,.T.);
#15062=EDGE_CURVE('',#12060,#12065,#6288,.T.);
#15063=EDGE_CURVE('',#12065,#12066,#6289,.T.);
#15064=EDGE_CURVE('',#12066,#12063,#6290,.T.);
#15065=EDGE_CURVE('',#12059,#12067,#6291,.T.);
#15066=EDGE_CURVE('',#12068,#12067,#6292,.T.);
#15067=EDGE_CURVE('',#12069,#12068,#6293,.T.);
#15068=EDGE_CURVE('',#12069,#12065,#6294,.T.);
#15069=EDGE_CURVE('',#12070,#12071,#6295,.T.);
#15070=EDGE_CURVE('',#12071,#12072,#6296,.T.);
#15071=EDGE_CURVE('',#12072,#12073,#6297,.T.);
#15072=EDGE_CURVE('',#12073,#12074,#6298,.T.);
#15073=EDGE_CURVE('',#12074,#12075,#6299,.T.);
#15074=EDGE_CURVE('',#12075,#12070,#6300,.T.);
#15075=EDGE_CURVE('',#12075,#12076,#6301,.T.);
#15076=EDGE_CURVE('',#12077,#12076,#6302,.F.);
#15077=EDGE_CURVE('',#12077,#12078,#6303,.T.);
#15078=EDGE_CURVE('',#12078,#12070,#6304,.T.);
#15079=EDGE_CURVE('',#12079,#12074,#6305,.T.);
#15080=EDGE_CURVE('',#12079,#12076,#6306,.T.);
#15081=EDGE_CURVE('',#12073,#12080,#6307,.T.);
#15082=EDGE_CURVE('',#12080,#12081,#6308,.T.);
#15083=EDGE_CURVE('',#12081,#12079,#6309,.T.);
#15084=EDGE_CURVE('',#12082,#12083,#6310,.T.);
#15085=EDGE_CURVE('',#12083,#12084,#6311,.T.);
#15086=EDGE_CURVE('',#12084,#12085,#6312,.T.);
#15087=EDGE_CURVE('',#12085,#12086,#6313,.T.);
#15088=EDGE_CURVE('',#12086,#12087,#6314,.T.);
#15089=EDGE_CURVE('',#12087,#12082,#6315,.T.);
#15090=EDGE_CURVE('',#12088,#12083,#6316,.T.);
#15091=EDGE_CURVE('',#12089,#12088,#6317,.T.);
#15092=EDGE_CURVE('',#12084,#12089,#6318,.T.);
#15093=EDGE_CURVE('',#12090,#12082,#6319,.T.);
#15094=EDGE_CURVE('',#12090,#12091,#6320,.T.);
#15095=EDGE_CURVE('',#12092,#12091,#6321,.T.);
#15096=EDGE_CURVE('',#12088,#12092,#6322,.T.);
#15097=EDGE_CURVE('',#12087,#12093,#6323,.T.);
#15098=EDGE_CURVE('',#12093,#12094,#6324,.T.);
#15099=EDGE_CURVE('',#12094,#12090,#6325,.T.);
#15100=EDGE_CURVE('',#12095,#12096,#6326,.T.);
#15101=EDGE_CURVE('',#12096,#12097,#6327,.T.);
#15102=EDGE_CURVE('',#12097,#12098,#6328,.T.);
#15103=EDGE_CURVE('',#12098,#12099,#6329,.T.);
#15104=EDGE_CURVE('',#12099,#12100,#6330,.T.);
#15105=EDGE_CURVE('',#12100,#12095,#6331,.T.);
#15106=EDGE_CURVE('',#12098,#12101,#6332,.T.);
#15107=EDGE_CURVE('',#12101,#12102,#6333,.T.);
#15108=EDGE_CURVE('',#12103,#12102,#6334,.T.);
#15109=EDGE_CURVE('',#12103,#12099,#6335,.T.);
#15110=EDGE_CURVE('',#12097,#12104,#6336,.T.);
#15111=EDGE_CURVE('',#12105,#12104,#6337,.T.);
#15112=EDGE_CURVE('',#12106,#12105,#6338,.T.);
#15113=EDGE_CURVE('',#12106,#12101,#6339,.T.);
#15114=EDGE_CURVE('',#12107,#12096,#6340,.T.);
#15115=EDGE_CURVE('',#12104,#12107,#6341,.T.);
#15116=EDGE_CURVE('',#12107,#12108,#6342,.T.);
#15117=EDGE_CURVE('',#12108,#12109,#6343,.T.);
#15118=EDGE_CURVE('',#12109,#12110,#6344,.T.);
#15119=EDGE_CURVE('',#12110,#12105,#6345,.T.);
#15120=EDGE_CURVE('',#12110,#12111,#6346,.T.);
#15121=EDGE_CURVE('',#12111,#12112,#6347,.T.);
#15122=EDGE_CURVE('',#12112,#12106,#6348,.T.);
#15123=EDGE_CURVE('',#12113,#12114,#6349,.T.);
#15124=EDGE_CURVE('',#12114,#12115,#6350,.T.);
#15125=EDGE_CURVE('',#12115,#12116,#6351,.T.);
#15126=EDGE_CURVE('',#12116,#12117,#6352,.T.);
#15127=EDGE_CURVE('',#12117,#12118,#6353,.T.);
#15128=EDGE_CURVE('',#12118,#12113,#6354,.T.);
#15129=EDGE_CURVE('',#12119,#12117,#6355,.T.);
#15130=EDGE_CURVE('',#12120,#12119,#6356,.T.);
#15131=EDGE_CURVE('',#12118,#12120,#6357,.T.);
#15132=EDGE_CURVE('',#12116,#12121,#6358,.T.);
#15133=EDGE_CURVE('',#12121,#12122,#6359,.T.);
#15134=EDGE_CURVE('',#12119,#12122,#6360,.T.);
#15135=EDGE_CURVE('',#12053,#12121,#6361,.T.);
#15136=EDGE_CURVE('',#12115,#12046,#6362,.T.);
#15137=EDGE_CURVE('',#12123,#12124,#6363,.T.);
#15138=EDGE_CURVE('',#12124,#12125,#6364,.T.);
#15139=EDGE_CURVE('',#12125,#12126,#6365,.T.);
#15140=EDGE_CURVE('',#12126,#12127,#6366,.T.);
#15141=EDGE_CURVE('',#12127,#12128,#6367,.T.);
#15142=EDGE_CURVE('',#12128,#12123,#6368,.T.);
#15143=EDGE_CURVE('',#12129,#12124,#6369,.T.);
#15144=EDGE_CURVE('',#12130,#12129,#6370,.T.);
#15145=EDGE_CURVE('',#12125,#12130,#6371,.T.);
#15146=EDGE_CURVE('',#12131,#12123,#6372,.T.);
#15147=EDGE_CURVE('',#12131,#12132,#6373,.T.);
#15148=EDGE_CURVE('',#12133,#12132,#6374,.T.);
#15149=EDGE_CURVE('',#12129,#12133,#6375,.T.);
#15150=EDGE_CURVE('',#12128,#12134,#6376,.T.);
#15151=EDGE_CURVE('',#12134,#12135,#6377,.T.);
#15152=EDGE_CURVE('',#12135,#12131,#6378,.T.);
#15153=EDGE_CURVE('',#12136,#12137,#6379,.T.);
#15154=EDGE_CURVE('',#12137,#12138,#6380,.T.);
#15155=EDGE_CURVE('',#12138,#12139,#6381,.T.);
#15156=EDGE_CURVE('',#12139,#12140,#6382,.T.);
#15157=EDGE_CURVE('',#12140,#12141,#6383,.T.);
#15158=EDGE_CURVE('',#12141,#12136,#6384,.T.);
#15159=EDGE_CURVE('',#12139,#12142,#6385,.T.);
#15160=EDGE_CURVE('',#12142,#12143,#6386,.T.);
#15161=EDGE_CURVE('',#12144,#12143,#6387,.T.);
#15162=EDGE_CURVE('',#12144,#12140,#6388,.T.);
#15163=EDGE_CURVE('',#12138,#12145,#6389,.T.);
#15164=EDGE_CURVE('',#12146,#12145,#6390,.T.);
#15165=EDGE_CURVE('',#12147,#12146,#6391,.T.);
#15166=EDGE_CURVE('',#12147,#12142,#6392,.T.);
#15167=EDGE_CURVE('',#12148,#12137,#6393,.T.);
#15168=EDGE_CURVE('',#12145,#12148,#6394,.T.);
#15169=EDGE_CURVE('',#12148,#12149,#6395,.T.);
#15170=EDGE_CURVE('',#12149,#12150,#6396,.T.);
#15171=EDGE_CURVE('',#12150,#12151,#6397,.T.);
#15172=EDGE_CURVE('',#12151,#12146,#6398,.T.);
#15173=EDGE_CURVE('',#12151,#12152,#6399,.T.);
#15174=EDGE_CURVE('',#12152,#12153,#6400,.T.);
#15175=EDGE_CURVE('',#12153,#12147,#6401,.T.);
#15176=EDGE_CURVE('',#12154,#12155,#6402,.T.);
#15177=EDGE_CURVE('',#12155,#12156,#6403,.T.);
#15178=EDGE_CURVE('',#12156,#12157,#6404,.T.);
#15179=EDGE_CURVE('',#12157,#12158,#6405,.T.);
#15180=EDGE_CURVE('',#12158,#12159,#6406,.T.);
#15181=EDGE_CURVE('',#12159,#12154,#6407,.T.);
#15182=EDGE_CURVE('',#12160,#12158,#6408,.T.);
#15183=EDGE_CURVE('',#12161,#12160,#6409,.T.);
#15184=EDGE_CURVE('',#12159,#12161,#6410,.T.);
#15185=EDGE_CURVE('',#12157,#12162,#6411,.T.);
#15186=EDGE_CURVE('',#12162,#12163,#6412,.T.);
#15187=EDGE_CURVE('',#12160,#12163,#6413,.T.);
#15188=EDGE_CURVE('',#12041,#12162,#6414,.T.);
#15189=EDGE_CURVE('',#12156,#12034,#6415,.T.);
#15190=EDGE_CURVE('',#12164,#12165,#6416,.T.);
#15191=EDGE_CURVE('',#12165,#12166,#6417,.T.);
#15192=EDGE_CURVE('',#12166,#12167,#6418,.T.);
#15193=EDGE_CURVE('',#12167,#12168,#6419,.T.);
#15194=EDGE_CURVE('',#12168,#12169,#6420,.T.);
#15195=EDGE_CURVE('',#12169,#12164,#6421,.T.);
#15196=EDGE_CURVE('',#12167,#12170,#6422,.T.);
#15197=EDGE_CURVE('',#12170,#12171,#6423,.T.);
#15198=EDGE_CURVE('',#12172,#12171,#6424,.T.);
#15199=EDGE_CURVE('',#12172,#12168,#6425,.T.);
#15200=EDGE_CURVE('',#12166,#12173,#6426,.T.);
#15201=EDGE_CURVE('',#12174,#12173,#6427,.T.);
#15202=EDGE_CURVE('',#12175,#12174,#6428,.T.);
#15203=EDGE_CURVE('',#12175,#12170,#6429,.T.);
#15204=EDGE_CURVE('',#12176,#12165,#6430,.T.);
#15205=EDGE_CURVE('',#12173,#12176,#6431,.T.);
#15206=EDGE_CURVE('',#12176,#12177,#6432,.T.);
#15207=EDGE_CURVE('',#12177,#12178,#6433,.T.);
#15208=EDGE_CURVE('',#12178,#12179,#6434,.T.);
#15209=EDGE_CURVE('',#12179,#12174,#6435,.T.);
#15210=EDGE_CURVE('',#12179,#12180,#6436,.T.);
#15211=EDGE_CURVE('',#12180,#12181,#6437,.T.);
#15212=EDGE_CURVE('',#12181,#12175,#6438,.T.);
#15213=EDGE_CURVE('',#12182,#12183,#6439,.T.);
#15214=EDGE_CURVE('',#12183,#12184,#6440,.T.);
#15215=EDGE_CURVE('',#12184,#12185,#6441,.T.);
#15216=EDGE_CURVE('',#12185,#12186,#6442,.T.);
#15217=EDGE_CURVE('',#12186,#12187,#6443,.T.);
#15218=EDGE_CURVE('',#12187,#12182,#6444,.T.);
#15219=EDGE_CURVE('',#12188,#12186,#6445,.T.);
#15220=EDGE_CURVE('',#12189,#12188,#6446,.T.);
#15221=EDGE_CURVE('',#12187,#12189,#6447,.T.);
#15222=EDGE_CURVE('',#12185,#12190,#6448,.T.);
#15223=EDGE_CURVE('',#12190,#12191,#6449,.T.);
#15224=EDGE_CURVE('',#12188,#12191,#6450,.T.);
#15225=EDGE_CURVE('',#12184,#12192,#6451,.T.);
#15226=EDGE_CURVE('',#12193,#12192,#6452,.T.);
#15227=EDGE_CURVE('',#12194,#12193,#6453,.T.);
#15228=EDGE_CURVE('',#12194,#12190,#6454,.T.);
#15229=EDGE_CURVE('',#12192,#12195,#6455,.T.);
#15230=EDGE_CURVE('',#12195,#12196,#6456,.T.);
#15231=EDGE_CURVE('',#12196,#12197,#6457,.T.);
#15232=EDGE_CURVE('',#12197,#12198,#6458,.T.);
#15233=EDGE_CURVE('',#12198,#12193,#6459,.T.);
#15234=EDGE_CURVE('',#12199,#12197,#6460,.T.);
#15235=EDGE_CURVE('',#12199,#12200,#6461,.T.);
#15236=EDGE_CURVE('',#12198,#12200,#6462,.T.);
#15237=EDGE_CURVE('',#12196,#12201,#6463,.T.);
#15238=EDGE_CURVE('',#12201,#12202,#6464,.T.);
#15239=EDGE_CURVE('',#12202,#12199,#6465,.T.);
#15240=EDGE_CURVE('',#12203,#12182,#6466,.T.);
#15241=EDGE_CURVE('',#12203,#12201,#6467,.T.);
#15242=EDGE_CURVE('',#12195,#12183,#6468,.T.);
#15243=EDGE_CURVE('',#12204,#12205,#6469,.T.);
#15244=EDGE_CURVE('',#12205,#12206,#6470,.T.);
#15245=EDGE_CURVE('',#12206,#12207,#6471,.T.);
#15246=EDGE_CURVE('',#12207,#12208,#6472,.T.);
#15247=EDGE_CURVE('',#12208,#12209,#6473,.T.);
#15248=EDGE_CURVE('',#12209,#12204,#6474,.T.);
#15249=EDGE_CURVE('',#12207,#12210,#6475,.T.);
#15250=EDGE_CURVE('',#12210,#12211,#6476,.T.);
#15251=EDGE_CURVE('',#12212,#12211,#6477,.T.);
#15252=EDGE_CURVE('',#12212,#12208,#6478,.T.);
#15253=EDGE_CURVE('',#12206,#12213,#6479,.T.);
#15254=EDGE_CURVE('',#12214,#12213,#6480,.T.);
#15255=EDGE_CURVE('',#12215,#12214,#6481,.T.);
#15256=EDGE_CURVE('',#12215,#12210,#6482,.T.);
#15257=EDGE_CURVE('',#12216,#12205,#6483,.T.);
#15258=EDGE_CURVE('',#12213,#12216,#6484,.T.);
#15259=EDGE_CURVE('',#12216,#12217,#6485,.T.);
#15260=EDGE_CURVE('',#12217,#12218,#6486,.T.);
#15261=EDGE_CURVE('',#12218,#12219,#6487,.T.);
#15262=EDGE_CURVE('',#12219,#12214,#6488,.T.);
#15263=EDGE_CURVE('',#12219,#12220,#6489,.T.);
#15264=EDGE_CURVE('',#12220,#12221,#6490,.T.);
#15265=EDGE_CURVE('',#12221,#12215,#6491,.T.);
#15266=EDGE_CURVE('',#12222,#12223,#6492,.T.);
#15267=EDGE_CURVE('',#12223,#12224,#6493,.T.);
#15268=EDGE_CURVE('',#12224,#12225,#6494,.T.);
#15269=EDGE_CURVE('',#12225,#12226,#6495,.T.);
#15270=EDGE_CURVE('',#12226,#12227,#6496,.T.);
#15271=EDGE_CURVE('',#12227,#12222,#6497,.T.);
#15272=EDGE_CURVE('',#12225,#12228,#6498,.T.);
#15273=EDGE_CURVE('',#12228,#12229,#6499,.T.);
#15274=EDGE_CURVE('',#12230,#12229,#6500,.T.);
#15275=EDGE_CURVE('',#12230,#12226,#6501,.T.);
#15276=EDGE_CURVE('',#12224,#12231,#6502,.T.);
#15277=EDGE_CURVE('',#12232,#12231,#6503,.T.);
#15278=EDGE_CURVE('',#12233,#12232,#6504,.T.);
#15279=EDGE_CURVE('',#12233,#12228,#6505,.T.);
#15280=EDGE_CURVE('',#12234,#12223,#6506,.T.);
#15281=EDGE_CURVE('',#12231,#12234,#6507,.T.);
#15282=EDGE_CURVE('',#12234,#12235,#6508,.T.);
#15283=EDGE_CURVE('',#12235,#12236,#6509,.T.);
#15284=EDGE_CURVE('',#12236,#12237,#6510,.T.);
#15285=EDGE_CURVE('',#12237,#12232,#6511,.T.);
#15286=EDGE_CURVE('',#12237,#12238,#6512,.T.);
#15287=EDGE_CURVE('',#12238,#12239,#6513,.T.);
#15288=EDGE_CURVE('',#12239,#12233,#6514,.T.);
#15289=EDGE_CURVE('',#12240,#12241,#6515,.T.);
#15290=EDGE_CURVE('',#12241,#12242,#6516,.T.);
#15291=EDGE_CURVE('',#12242,#12243,#6517,.T.);
#15292=EDGE_CURVE('',#12243,#12244,#6518,.T.);
#15293=EDGE_CURVE('',#12244,#12245,#6519,.T.);
#15294=EDGE_CURVE('',#12245,#12240,#6520,.T.);
#15295=EDGE_CURVE('',#12245,#12246,#6521,.T.);
#15296=EDGE_CURVE('',#12247,#12246,#6522,.T.);
#15297=EDGE_CURVE('',#12247,#12248,#6523,.T.);
#15298=EDGE_CURVE('',#12248,#12240,#6524,.T.);
#15299=EDGE_CURVE('',#12249,#12244,#6525,.T.);
#15300=EDGE_CURVE('',#12246,#12249,#6526,.T.);
#15301=EDGE_CURVE('',#12243,#12250,#6527,.T.);
#15302=EDGE_CURVE('',#12250,#12251,#6528,.T.);
#15303=EDGE_CURVE('',#12249,#12251,#6529,.T.);
#15304=EDGE_CURVE('',#12252,#12253,#6530,.T.);
#15305=EDGE_CURVE('',#12253,#12254,#6531,.T.);
#15306=EDGE_CURVE('',#12254,#12255,#6532,.T.);
#15307=EDGE_CURVE('',#12255,#12256,#6533,.T.);
#15308=EDGE_CURVE('',#12256,#12257,#6534,.T.);
#15309=EDGE_CURVE('',#12257,#12252,#6535,.T.);
#15310=EDGE_CURVE('',#12255,#12258,#6536,.T.);
#15311=EDGE_CURVE('',#12258,#12259,#6537,.T.);
#15312=EDGE_CURVE('',#12260,#12259,#6538,.T.);
#15313=EDGE_CURVE('',#12260,#12256,#6539,.T.);
#15314=EDGE_CURVE('',#12254,#12261,#6540,.T.);
#15315=EDGE_CURVE('',#12262,#12261,#6541,.T.);
#15316=EDGE_CURVE('',#12263,#12262,#6542,.T.);
#15317=EDGE_CURVE('',#12263,#12258,#6543,.T.);
#15318=EDGE_CURVE('',#12264,#12253,#6544,.T.);
#15319=EDGE_CURVE('',#12261,#12264,#6545,.T.);
#15320=EDGE_CURVE('',#12264,#12265,#6546,.T.);
#15321=EDGE_CURVE('',#12265,#12266,#6547,.T.);
#15322=EDGE_CURVE('',#12266,#12267,#6548,.T.);
#15323=EDGE_CURVE('',#12267,#12262,#6549,.T.);
#15324=EDGE_CURVE('',#12267,#12268,#6550,.T.);
#15325=EDGE_CURVE('',#12268,#12269,#6551,.T.);
#15326=EDGE_CURVE('',#12269,#12263,#6552,.T.);
#15327=EDGE_CURVE('',#12270,#12271,#6553,.T.);
#15328=EDGE_CURVE('',#12271,#12272,#6554,.T.);
#15329=EDGE_CURVE('',#12272,#12273,#6555,.T.);
#15330=EDGE_CURVE('',#12273,#12274,#6556,.T.);
#15331=EDGE_CURVE('',#12274,#12275,#6557,.T.);
#15332=EDGE_CURVE('',#12275,#12270,#6558,.T.);
#15333=EDGE_CURVE('',#12273,#12276,#6559,.T.);
#15334=EDGE_CURVE('',#12276,#12277,#6560,.T.);
#15335=EDGE_CURVE('',#12278,#12277,#6561,.T.);
#15336=EDGE_CURVE('',#12278,#12274,#6562,.T.);
#15337=EDGE_CURVE('',#12272,#12279,#6563,.T.);
#15338=EDGE_CURVE('',#12280,#12279,#6564,.T.);
#15339=EDGE_CURVE('',#12281,#12280,#6565,.T.);
#15340=EDGE_CURVE('',#12281,#12276,#6566,.T.);
#15341=EDGE_CURVE('',#12282,#12271,#6567,.T.);
#15342=EDGE_CURVE('',#12279,#12282,#6568,.T.);
#15343=EDGE_CURVE('',#12282,#12283,#6569,.T.);
#15344=EDGE_CURVE('',#12283,#12284,#6570,.T.);
#15345=EDGE_CURVE('',#12284,#12285,#6571,.T.);
#15346=EDGE_CURVE('',#12285,#12280,#6572,.T.);
#15347=EDGE_CURVE('',#12285,#12286,#6573,.T.);
#15348=EDGE_CURVE('',#12286,#12287,#6574,.T.);
#15349=EDGE_CURVE('',#12287,#12281,#6575,.T.);
#15350=EDGE_CURVE('',#12067,#12288,#6576,.T.);
#15351=EDGE_CURVE('',#12288,#12289,#6577,.T.);
#15352=EDGE_CURVE('',#12289,#12290,#6578,.T.);
#15353=EDGE_CURVE('',#12290,#12291,#6579,.T.);
#15354=EDGE_CURVE('',#12291,#12068,#6580,.T.);
#15355=EDGE_CURVE('',#12291,#12292,#6581,.T.);
#15356=EDGE_CURVE('',#12293,#12292,#6582,.T.);
#15357=EDGE_CURVE('',#12293,#12069,#6583,.T.);
#15358=EDGE_CURVE('',#12294,#12290,#6584,.T.);
#15359=EDGE_CURVE('',#12292,#12294,#6585,.T.);
#15360=EDGE_CURVE('',#12289,#12295,#6586,.T.);
#15361=EDGE_CURVE('',#12295,#12296,#6587,.T.);
#15362=EDGE_CURVE('',#12294,#12296,#6588,.T.);
#15363=EDGE_CURVE('',#12297,#12298,#6589,.T.);
#15364=EDGE_CURVE('',#12298,#12299,#6590,.T.);
#15365=EDGE_CURVE('',#12299,#12300,#6591,.T.);
#15366=EDGE_CURVE('',#12300,#12297,#6592,.T.);
#15367=EDGE_CURVE('',#12301,#12300,#6593,.T.);
#15368=EDGE_CURVE('',#12302,#12301,#6594,.T.);
#15369=EDGE_CURVE('',#12297,#12302,#6595,.T.);
#15370=EDGE_CURVE('',#12303,#12303,#10876,.T.);
#15371=EDGE_CURVE('',#12299,#12304,#6596,.T.);
#15372=EDGE_CURVE('',#12305,#12304,#6597,.T.);
#15373=EDGE_CURVE('',#12306,#12305,#6598,.T.);
#15374=EDGE_CURVE('',#12301,#12306,#6599,.T.);
#15375=EDGE_CURVE('',#12307,#12308,#6600,.T.);
#15376=EDGE_CURVE('',#12308,#12305,#6601,.T.);
#15377=EDGE_CURVE('',#12305,#12309,#6602,.T.);
#15378=EDGE_CURVE('',#12309,#12310,#6603,.T.);
#15379=EDGE_CURVE('',#12310,#12311,#6604,.T.);
#15380=EDGE_CURVE('',#12311,#12307,#6605,.T.);
#15381=EDGE_CURVE('',#12308,#12312,#6606,.T.);
#15382=EDGE_CURVE('',#12306,#12312,#6607,.T.);
#15383=EDGE_CURVE('',#12307,#12313,#6608,.T.);
#15384=EDGE_CURVE('',#12313,#12314,#6609,.T.);
#15385=EDGE_CURVE('',#12314,#12315,#6610,.T.);
#15386=EDGE_CURVE('',#12315,#12316,#6611,.T.);
#15387=EDGE_CURVE('',#12316,#12308,#6612,.T.);
#15388=EDGE_CURVE('',#12311,#12317,#6613,.T.);
#15389=EDGE_CURVE('',#12318,#12317,#6614,.T.);
#15390=EDGE_CURVE('',#12319,#12318,#6615,.T.);
#15391=EDGE_CURVE('',#12319,#12313,#6616,.T.);
#15392=EDGE_CURVE('',#12312,#12302,#6617,.T.);
#15393=EDGE_CURVE('',#12320,#12321,#6618,.T.);
#15394=EDGE_CURVE('',#12321,#12322,#6619,.T.);
#15395=EDGE_CURVE('',#12322,#12323,#6620,.T.);
#15396=EDGE_CURVE('',#12323,#12324,#6621,.T.);
#15397=EDGE_CURVE('',#12324,#12325,#6622,.T.);
#15398=EDGE_CURVE('',#12325,#12320,#6623,.T.);
#15399=EDGE_CURVE('',#12320,#12326,#6624,.T.);
#15400=EDGE_CURVE('',#12326,#12319,#6625,.T.);
#15401=EDGE_CURVE('',#12327,#12318,#6626,.T.);
#15402=EDGE_CURVE('',#12327,#12321,#6627,.T.);
#15403=EDGE_CURVE('',#12325,#12328,#6628,.T.);
#15404=EDGE_CURVE('',#12329,#12328,#6629,.T.);
#15405=EDGE_CURVE('',#12330,#12329,#6630,.T.);
#15406=EDGE_CURVE('',#12330,#12326,#6631,.T.);
#15407=EDGE_CURVE('',#12331,#12324,#6632,.T.);
#15408=EDGE_CURVE('',#12328,#12331,#6633,.T.);
#15409=EDGE_CURVE('',#12332,#12333,#6634,.T.);
#15410=EDGE_CURVE('',#12333,#12334,#6635,.T.);
#15411=EDGE_CURVE('',#12334,#12335,#6636,.T.);
#15412=EDGE_CURVE('',#12335,#12336,#6637,.T.);
#15413=EDGE_CURVE('',#12336,#12337,#6638,.T.);
#15414=EDGE_CURVE('',#12337,#12332,#6639,.T.);
#15415=EDGE_CURVE('',#12335,#12338,#6640,.T.);
#15416=EDGE_CURVE('',#12338,#12339,#6641,.T.);
#15417=EDGE_CURVE('',#12340,#12339,#6642,.T.);
#15418=EDGE_CURVE('',#12340,#12336,#6643,.T.);
#15419=EDGE_CURVE('',#12334,#12341,#6644,.T.);
#15420=EDGE_CURVE('',#12342,#12341,#6645,.T.);
#15421=EDGE_CURVE('',#12343,#12342,#6646,.T.);
#15422=EDGE_CURVE('',#12343,#12338,#6647,.T.);
#15423=EDGE_CURVE('',#12344,#12333,#6648,.T.);
#15424=EDGE_CURVE('',#12341,#12344,#6649,.T.);
#15425=EDGE_CURVE('',#12344,#12345,#6650,.T.);
#15426=EDGE_CURVE('',#12345,#12346,#6651,.T.);
#15427=EDGE_CURVE('',#12346,#12347,#6652,.T.);
#15428=EDGE_CURVE('',#12347,#12342,#6653,.T.);
#15429=EDGE_CURVE('',#12347,#12348,#6654,.T.);
#15430=EDGE_CURVE('',#12348,#12349,#6655,.T.);
#15431=EDGE_CURVE('',#12349,#12343,#6656,.T.);
#15432=EDGE_CURVE('',#12350,#12351,#6657,.T.);
#15433=EDGE_CURVE('',#12351,#12352,#6658,.T.);
#15434=EDGE_CURVE('',#12352,#12353,#6659,.T.);
#15435=EDGE_CURVE('',#12353,#12354,#6660,.T.);
#15436=EDGE_CURVE('',#12354,#12355,#6661,.T.);
#15437=EDGE_CURVE('',#12355,#12350,#6662,.T.);
#15438=EDGE_CURVE('',#12353,#12356,#6663,.T.);
#15439=EDGE_CURVE('',#12356,#12357,#6664,.T.);
#15440=EDGE_CURVE('',#12358,#12357,#6665,.T.);
#15441=EDGE_CURVE('',#12358,#12354,#6666,.T.);
#15442=EDGE_CURVE('',#12352,#12359,#6667,.T.);
#15443=EDGE_CURVE('',#12360,#12359,#6668,.T.);
#15444=EDGE_CURVE('',#12361,#12360,#6669,.T.);
#15445=EDGE_CURVE('',#12361,#12356,#6670,.T.);
#15446=EDGE_CURVE('',#12362,#12351,#6671,.T.);
#15447=EDGE_CURVE('',#12359,#12362,#6672,.T.);
#15448=EDGE_CURVE('',#12362,#12363,#6673,.T.);
#15449=EDGE_CURVE('',#12363,#12364,#6674,.T.);
#15450=EDGE_CURVE('',#12364,#12365,#6675,.T.);
#15451=EDGE_CURVE('',#12365,#12360,#6676,.T.);
#15452=EDGE_CURVE('',#12365,#12366,#6677,.T.);
#15453=EDGE_CURVE('',#12366,#12367,#6678,.T.);
#15454=EDGE_CURVE('',#12367,#12361,#6679,.T.);
#15455=EDGE_CURVE('',#12368,#12369,#6680,.T.);
#15456=EDGE_CURVE('',#12369,#12370,#6681,.T.);
#15457=EDGE_CURVE('',#12370,#12371,#6682,.T.);
#15458=EDGE_CURVE('',#12371,#12372,#6683,.T.);
#15459=EDGE_CURVE('',#12372,#12373,#6684,.T.);
#15460=EDGE_CURVE('',#12373,#12368,#6685,.T.);
#15461=EDGE_CURVE('',#12371,#12374,#6686,.T.);
#15462=EDGE_CURVE('',#12374,#12375,#6687,.T.);
#15463=EDGE_CURVE('',#12376,#12375,#6688,.T.);
#15464=EDGE_CURVE('',#12376,#12372,#6689,.T.);
#15465=EDGE_CURVE('',#12370,#12377,#6690,.T.);
#15466=EDGE_CURVE('',#12378,#12377,#6691,.T.);
#15467=EDGE_CURVE('',#12379,#12378,#6692,.T.);
#15468=EDGE_CURVE('',#12379,#12374,#6693,.T.);
#15469=EDGE_CURVE('',#12380,#12369,#6694,.T.);
#15470=EDGE_CURVE('',#12377,#12380,#6695,.T.);
#15471=EDGE_CURVE('',#12380,#12381,#6696,.T.);
#15472=EDGE_CURVE('',#12381,#12382,#6697,.T.);
#15473=EDGE_CURVE('',#12382,#12383,#6698,.T.);
#15474=EDGE_CURVE('',#12383,#12378,#6699,.T.);
#15475=EDGE_CURVE('',#12383,#12384,#6700,.T.);
#15476=EDGE_CURVE('',#12384,#12385,#6701,.T.);
#15477=EDGE_CURVE('',#12385,#12379,#6702,.T.);
#15478=EDGE_CURVE('',#12386,#12387,#6703,.T.);
#15479=EDGE_CURVE('',#12387,#12388,#6704,.T.);
#15480=EDGE_CURVE('',#12388,#12389,#6705,.T.);
#15481=EDGE_CURVE('',#12389,#12390,#6706,.T.);
#15482=EDGE_CURVE('',#12390,#12391,#6707,.T.);
#15483=EDGE_CURVE('',#12391,#12386,#6708,.T.);
#15484=EDGE_CURVE('',#12389,#12392,#6709,.T.);
#15485=EDGE_CURVE('',#12392,#12393,#6710,.T.);
#15486=EDGE_CURVE('',#12394,#12393,#6711,.T.);
#15487=EDGE_CURVE('',#12394,#12390,#6712,.T.);
#15488=EDGE_CURVE('',#12388,#12395,#6713,.T.);
#15489=EDGE_CURVE('',#12396,#12395,#6714,.T.);
#15490=EDGE_CURVE('',#12397,#12396,#6715,.T.);
#15491=EDGE_CURVE('',#12397,#12392,#6716,.T.);
#15492=EDGE_CURVE('',#12398,#12387,#6717,.T.);
#15493=EDGE_CURVE('',#12395,#12398,#6718,.T.);
#15494=EDGE_CURVE('',#12398,#12399,#6719,.T.);
#15495=EDGE_CURVE('',#12399,#12400,#6720,.T.);
#15496=EDGE_CURVE('',#12400,#12401,#6721,.T.);
#15497=EDGE_CURVE('',#12401,#12396,#6722,.T.);
#15498=EDGE_CURVE('',#12401,#12402,#6723,.T.);
#15499=EDGE_CURVE('',#12402,#12403,#6724,.T.);
#15500=EDGE_CURVE('',#12403,#12397,#6725,.T.);
#15501=EDGE_CURVE('',#12404,#12405,#6726,.T.);
#15502=EDGE_CURVE('',#12405,#12406,#6727,.T.);
#15503=EDGE_CURVE('',#12406,#12407,#6728,.T.);
#15504=EDGE_CURVE('',#12407,#12408,#6729,.T.);
#15505=EDGE_CURVE('',#12408,#12409,#6730,.T.);
#15506=EDGE_CURVE('',#12409,#12404,#6731,.T.);
#15507=EDGE_CURVE('',#12410,#12408,#6732,.T.);
#15508=EDGE_CURVE('',#12411,#12410,#6733,.T.);
#15509=EDGE_CURVE('',#12409,#12411,#6734,.T.);
#15510=EDGE_CURVE('',#12407,#12412,#6735,.T.);
#15511=EDGE_CURVE('',#12412,#12413,#6736,.T.);
#15512=EDGE_CURVE('',#12410,#12413,#6737,.T.);
#15513=EDGE_CURVE('',#12078,#12412,#6738,.T.);
#15514=EDGE_CURVE('',#12406,#12071,#6739,.T.);
#15515=EDGE_CURVE('',#12296,#12287,#6740,.T.);
#15516=EDGE_CURVE('',#12286,#12294,#6741,.T.);
#15517=EDGE_CURVE('',#12414,#12286,#6742,.T.);
#15518=EDGE_CURVE('',#12292,#12414,#6743,.T.);
#15519=EDGE_CURVE('',#12414,#12284,#6744,.T.);
#15520=EDGE_CURVE('',#12277,#12269,#6745,.T.);
#15521=EDGE_CURVE('',#12268,#12278,#6746,.T.);
#15522=EDGE_CURVE('',#12415,#12278,#6747,.T.);
#15523=EDGE_CURVE('',#12275,#12415,#6748,.T.);
#15524=EDGE_CURVE('',#12416,#12268,#6749,.T.);
#15525=EDGE_CURVE('',#12415,#12416,#6750,.T.);
#15526=EDGE_CURVE('',#12416,#12266,#6751,.T.);
#15527=EDGE_CURVE('',#12259,#12077,#6752,.T.);
#15528=EDGE_CURVE('',#12076,#12260,#6753,.T.);
#15529=EDGE_CURVE('',#12417,#12260,#6754,.T.);
#15530=EDGE_CURVE('',#12257,#12417,#6755,.T.);
#15531=EDGE_CURVE('',#12417,#12079,#6756,.T.);
#15532=EDGE_CURVE('',#12418,#12295,#6757,.T.);
#15533=EDGE_CURVE('',#12419,#12418,#6758,.T.);
#15534=EDGE_CURVE('',#12420,#12419,#6759,.T.);
#15535=EDGE_CURVE('',#12421,#12420,#6760,.T.);
#15536=EDGE_CURVE('',#12422,#12421,#6761,.T.);
#15537=EDGE_CURVE('',#12423,#12422,#6762,.T.);
#15538=EDGE_CURVE('',#12424,#12423,#6763,.T.);
#15539=EDGE_CURVE('',#12425,#12424,#6764,.T.);
#15540=EDGE_CURVE('',#12426,#12425,#6765,.T.);
#15541=EDGE_CURVE('',#12427,#12426,#6766,.T.);
#15542=EDGE_CURVE('',#12428,#12427,#6767,.T.);
#15543=EDGE_CURVE('',#12429,#12428,#6768,.T.);
#15544=EDGE_CURVE('',#12430,#12429,#6769,.T.);
#15545=EDGE_CURVE('',#12431,#12430,#6770,.T.);
#15546=EDGE_CURVE('',#12432,#12431,#6771,.T.);
#15547=EDGE_CURVE('',#12433,#12432,#6772,.T.);
#15548=EDGE_CURVE('',#12434,#12433,#6773,.T.);
#15549=EDGE_CURVE('',#12435,#12434,#6774,.T.);
#15550=EDGE_CURVE('',#12436,#12435,#6775,.T.);
#15551=EDGE_CURVE('',#12437,#12436,#6776,.T.);
#15552=EDGE_CURVE('',#12438,#12437,#6777,.T.);
#15553=EDGE_CURVE('',#12439,#12438,#6778,.T.);
#15554=EDGE_CURVE('',#12440,#12439,#6779,.T.);
#15555=EDGE_CURVE('',#12441,#12440,#6780,.T.);
#15556=EDGE_CURVE('',#12442,#12441,#6781,.T.);
#15557=EDGE_CURVE('',#12443,#12442,#6782,.T.);
#15558=EDGE_CURVE('',#12444,#12443,#6783,.T.);
#15559=EDGE_CURVE('',#12091,#12444,#6784,.T.);
#15560=EDGE_CURVE('',#12102,#12094,#6785,.T.);
#15561=EDGE_CURVE('',#12122,#12112,#6786,.T.);
#15562=EDGE_CURVE('',#12445,#12052,#6787,.T.);
#15563=EDGE_CURVE('',#12446,#12445,#6788,.T.);
#15564=EDGE_CURVE('',#12447,#12446,#6789,.T.);
#15565=EDGE_CURVE('',#12448,#12447,#6790,.T.);
#15566=EDGE_CURVE('',#12449,#12448,#6791,.T.);
#15567=EDGE_CURVE('',#12450,#12449,#6792,.T.);
#15568=EDGE_CURVE('',#12451,#12450,#6793,.T.);
#15569=EDGE_CURVE('',#12452,#12451,#6794,.T.);
#15570=EDGE_CURVE('',#12453,#12452,#6795,.T.);
#15571=EDGE_CURVE('',#12454,#12453,#6796,.T.);
#15572=EDGE_CURVE('',#12455,#12454,#6797,.T.);
#15573=EDGE_CURVE('',#12456,#12455,#6798,.T.);
#15574=EDGE_CURVE('',#12457,#12456,#6799,.T.);
#15575=EDGE_CURVE('',#12458,#12457,#6800,.T.);
#15576=EDGE_CURVE('',#12459,#12458,#6801,.T.);
#15577=EDGE_CURVE('',#12460,#12459,#6802,.T.);
#15578=EDGE_CURVE('',#12461,#12460,#6803,.T.);
#15579=EDGE_CURVE('',#12462,#12461,#6804,.T.);
#15580=EDGE_CURVE('',#12463,#12462,#6805,.T.);
#15581=EDGE_CURVE('',#12464,#12463,#6806,.T.);
#15582=EDGE_CURVE('',#12465,#12464,#6807,.T.);
#15583=EDGE_CURVE('',#12466,#12465,#6808,.T.);
#15584=EDGE_CURVE('',#12467,#12466,#6809,.T.);
#15585=EDGE_CURVE('',#12468,#12467,#6810,.T.);
#15586=EDGE_CURVE('',#12469,#12468,#6811,.T.);
#15587=EDGE_CURVE('',#12132,#12469,#6812,.T.);
#15588=EDGE_CURVE('',#12143,#12135,#6813,.T.);
#15589=EDGE_CURVE('',#12163,#12153,#6814,.T.);
#15590=EDGE_CURVE('',#12171,#12040,#6815,.T.);
#15591=EDGE_CURVE('',#12191,#12181,#6816,.T.);
#15592=EDGE_CURVE('',#12470,#12194,#6817,.T.);
#15593=EDGE_CURVE('',#12211,#12470,#6818,.T.);
#15594=EDGE_CURVE('',#12229,#12221,#6819,.T.);
#15595=EDGE_CURVE('',#12251,#12239,#6820,.T.);
#15596=EDGE_CURVE('',#12314,#12250,#6821,.T.);
#15597=EDGE_CURVE('',#12471,#12330,#6822,.T.);
#15598=EDGE_CURVE('',#12472,#12471,#6823,.T.);
#15599=EDGE_CURVE('',#12473,#12472,#6824,.T.);
#15600=EDGE_CURVE('',#12474,#12473,#6825,.T.);
#15601=EDGE_CURVE('',#12475,#12474,#6826,.T.);
#15602=EDGE_CURVE('',#12339,#12475,#6827,.T.);
#15603=EDGE_CURVE('',#12357,#12349,#6828,.T.);
#15604=EDGE_CURVE('',#12375,#12367,#6829,.T.);
#15605=EDGE_CURVE('',#12393,#12385,#6830,.T.);
#15606=EDGE_CURVE('',#12413,#12403,#6831,.T.);
#15607=EDGE_CURVE('',#12402,#12410,#6832,.T.);
#15608=EDGE_CURVE('',#12476,#12402,#6833,.T.);
#15609=EDGE_CURVE('',#12411,#12476,#6834,.T.);
#15610=EDGE_CURVE('',#12476,#12400,#6835,.T.);
#15611=EDGE_CURVE('',#12384,#12394,#6836,.T.);
#15612=EDGE_CURVE('',#12477,#12394,#6837,.T.);
#15613=EDGE_CURVE('',#12391,#12477,#6838,.T.);
#15614=EDGE_CURVE('',#12478,#12384,#6839,.T.);
#15615=EDGE_CURVE('',#12477,#12478,#6840,.T.);
#15616=EDGE_CURVE('',#12478,#12382,#6841,.T.);
#15617=EDGE_CURVE('',#12366,#12376,#6842,.T.);
#15618=EDGE_CURVE('',#12479,#12376,#6843,.T.);
#15619=EDGE_CURVE('',#12373,#12479,#6844,.T.);
#15620=EDGE_CURVE('',#12480,#12366,#6845,.T.);
#15621=EDGE_CURVE('',#12479,#12480,#6846,.T.);
#15622=EDGE_CURVE('',#12480,#12364,#6847,.T.);
#15623=EDGE_CURVE('',#12348,#12358,#6848,.T.);
#15624=EDGE_CURVE('',#12481,#12358,#6849,.T.);
#15625=EDGE_CURVE('',#12355,#12481,#6850,.T.);
#15626=EDGE_CURVE('',#12482,#12348,#6851,.T.);
#15627=EDGE_CURVE('',#12481,#12482,#6852,.T.);
#15628=EDGE_CURVE('',#12482,#12346,#6853,.T.);
#15629=EDGE_CURVE('',#12475,#12483,#6854,.F.);
#15630=EDGE_CURVE('',#12483,#12340,#6855,.T.);
#15631=EDGE_CURVE('',#12484,#12340,#6856,.T.);
#15632=EDGE_CURVE('',#12337,#12484,#6857,.T.);
#15633=EDGE_CURVE('',#12485,#12483,#6858,.T.);
#15634=EDGE_CURVE('',#12484,#12485,#6859,.T.);
#15635=EDGE_CURVE('',#12486,#12487,#6860,.T.);
#15636=EDGE_CURVE('',#12487,#12488,#6861,.T.);
#15637=EDGE_CURVE('',#12488,#12489,#6862,.T.);
#15638=EDGE_CURVE('',#12489,#12486,#6863,.T.);
#15639=EDGE_CURVE('',#12488,#12490,#6864,.T.);
#15640=EDGE_CURVE('',#12322,#12490,#6865,.T.);
#15641=EDGE_CURVE('',#12491,#12322,#6866,.T.);
#15642=EDGE_CURVE('',#12491,#12489,#6867,.T.);
#15643=EDGE_CURVE('',#12487,#12327,#6868,.T.);
#15644=EDGE_CURVE('',#12490,#12327,#6869,.T.);
#15645=EDGE_CURVE('',#12492,#12490,#6870,.T.);
#15646=EDGE_CURVE('',#12317,#12493,#6871,.T.);
#15647=EDGE_CURVE('',#12493,#12492,#6872,.T.);
#15648=EDGE_CURVE('',#12492,#12494,#6873,.T.);
#15649=EDGE_CURVE('',#12494,#12495,#6874,.T.);
#15650=EDGE_CURVE('',#12495,#12323,#6875,.T.);
#15651=EDGE_CURVE('',#12496,#12309,#6876,.T.);
#15652=EDGE_CURVE('',#12496,#12494,#6877,.T.);
#15653=EDGE_CURVE('',#12493,#12310,#6878,.T.);
#15654=EDGE_CURVE('',#12331,#12497,#6879,.T.);
#15655=EDGE_CURVE('',#12497,#12498,#6880,.T.);
#15656=EDGE_CURVE('',#12498,#12499,#6881,.T.);
#15657=EDGE_CURVE('',#12499,#12329,#6882,.T.);
#15658=EDGE_CURVE('',#12499,#12500,#6883,.T.);
#15659=EDGE_CURVE('',#12500,#12471,#6884,.T.);
#15660=EDGE_CURVE('',#12501,#12502,#6885,.T.);
#15661=EDGE_CURVE('',#12502,#12503,#6886,.T.);
#15662=EDGE_CURVE('',#12503,#12504,#6887,.T.);
#15663=EDGE_CURVE('',#12504,#12505,#6888,.T.);
#15664=EDGE_CURVE('',#12505,#12506,#6889,.T.);
#15665=EDGE_CURVE('',#12506,#12501,#6890,.T.);
#15666=EDGE_CURVE('',#12504,#12473,#6891,.T.);
#15667=EDGE_CURVE('',#12507,#12472,#6892,.T.);
#15668=EDGE_CURVE('',#12507,#12505,#6893,.T.);
#15669=EDGE_CURVE('',#12503,#12508,#6894,.T.);
#15670=EDGE_CURVE('',#12509,#12508,#6895,.T.);
#15671=EDGE_CURVE('',#12474,#12509,#6896,.T.);
#15672=EDGE_CURVE('',#12510,#12502,#6897,.T.);
#15673=EDGE_CURVE('',#12508,#12510,#6898,.T.);
#15674=EDGE_CURVE('',#12510,#12511,#6899,.T.);
#15675=EDGE_CURVE('',#12511,#12512,#6900,.T.);
#15676=EDGE_CURVE('',#12512,#12513,#6901,.T.);
#15677=EDGE_CURVE('',#12513,#12509,#6902,.T.);
#15678=EDGE_CURVE('',#12513,#12483,#6903,.T.);
#15679=EDGE_CURVE('',#12485,#12512,#6904,.T.);
#15680=EDGE_CURVE('',#12500,#12507,#6905,.T.);
#15681=EDGE_CURVE('',#12514,#12507,#6906,.T.);
#15682=EDGE_CURVE('',#12506,#12514,#6907,.T.);
#15683=EDGE_CURVE('',#12515,#12500,#6908,.T.);
#15684=EDGE_CURVE('',#12514,#12515,#6909,.T.);
#15685=EDGE_CURVE('',#12515,#12498,#6910,.T.);
#15686=EDGE_CURVE('',#12238,#12249,#6911,.T.);
#15687=EDGE_CURVE('',#12516,#12238,#6912,.T.);
#15688=EDGE_CURVE('',#12246,#12516,#6913,.T.);
#15689=EDGE_CURVE('',#12516,#12236,#6914,.T.);
#15690=EDGE_CURVE('',#12220,#12230,#6915,.T.);
#15691=EDGE_CURVE('',#12517,#12230,#6916,.T.);
#15692=EDGE_CURVE('',#12227,#12517,#6917,.T.);
#15693=EDGE_CURVE('',#12518,#12220,#6918,.T.);
#15694=EDGE_CURVE('',#12517,#12518,#6919,.T.);
#15695=EDGE_CURVE('',#12518,#12218,#6920,.T.);
#15696=EDGE_CURVE('',#12200,#12470,#6921,.T.);
#15697=EDGE_CURVE('',#12200,#12212,#6922,.T.);
#15698=EDGE_CURVE('',#12519,#12212,#6923,.T.);
#15699=EDGE_CURVE('',#12209,#12519,#6924,.T.);
#15700=EDGE_CURVE('',#12519,#12199,#6925,.T.);
#15701=EDGE_CURVE('',#12180,#12188,#6926,.T.);
#15702=EDGE_CURVE('',#12520,#12180,#6927,.T.);
#15703=EDGE_CURVE('',#12189,#12520,#6928,.T.);
#15704=EDGE_CURVE('',#12520,#12178,#6929,.T.);
#15705=EDGE_CURVE('',#12039,#12172,#6930,.T.);
#15706=EDGE_CURVE('',#12521,#12172,#6931,.T.);
#15707=EDGE_CURVE('',#12169,#12521,#6932,.T.);
#15708=EDGE_CURVE('',#12521,#12042,#6933,.T.);
#15709=EDGE_CURVE('',#12152,#12160,#6934,.T.);
#15710=EDGE_CURVE('',#12522,#12152,#6935,.T.);
#15711=EDGE_CURVE('',#12161,#12522,#6936,.T.);
#15712=EDGE_CURVE('',#12522,#12150,#6937,.T.);
#15713=EDGE_CURVE('',#12134,#12144,#6938,.T.);
#15714=EDGE_CURVE('',#12523,#12144,#6939,.T.);
#15715=EDGE_CURVE('',#12141,#12523,#6940,.T.);
#15716=EDGE_CURVE('',#12524,#12134,#6941,.T.);
#15717=EDGE_CURVE('',#12523,#12524,#6942,.T.);
#15718=EDGE_CURVE('',#12524,#12127,#6943,.T.);
#15719=EDGE_CURVE('',#12525,#12526,#6944,.T.);
#15720=EDGE_CURVE('',#12526,#12527,#6945,.T.);
#15721=EDGE_CURVE('',#12527,#12528,#6946,.T.);
#15722=EDGE_CURVE('',#12528,#12529,#6947,.T.);
#15723=EDGE_CURVE('',#12529,#12530,#6948,.T.);
#15724=EDGE_CURVE('',#12530,#12525,#6949,.T.);
#15725=EDGE_CURVE('',#12528,#12446,#6950,.T.);
#15726=EDGE_CURVE('',#12531,#12445,#6951,.T.);
#15727=EDGE_CURVE('',#12531,#12529,#6952,.T.);
#15728=EDGE_CURVE('',#12527,#12532,#6953,.T.);
#15729=EDGE_CURVE('',#12533,#12532,#6954,.T.);
#15730=EDGE_CURVE('',#12447,#12533,#6955,.T.);
#15731=EDGE_CURVE('',#12534,#12526,#6956,.T.);
#15732=EDGE_CURVE('',#12532,#12534,#6957,.T.);
#15733=EDGE_CURVE('',#12534,#12535,#6958,.T.);
#15734=EDGE_CURVE('',#12535,#12536,#6959,.T.);
#15735=EDGE_CURVE('',#12536,#12537,#6960,.T.);
#15736=EDGE_CURVE('',#12537,#12533,#6961,.T.);
#15737=EDGE_CURVE('',#12537,#12538,#6962,.T.);
#15738=EDGE_CURVE('',#12538,#12448,#6963,.T.);
#15739=EDGE_CURVE('',#12539,#12540,#6964,.T.);
#15740=EDGE_CURVE('',#12540,#12541,#6965,.T.);
#15741=EDGE_CURVE('',#12541,#12542,#6966,.T.);
#15742=EDGE_CURVE('',#12542,#12543,#6967,.T.);
#15743=EDGE_CURVE('',#12543,#12544,#6968,.T.);
#15744=EDGE_CURVE('',#12544,#12539,#6969,.T.);
#15745=EDGE_CURVE('',#12542,#12450,#6970,.T.);
#15746=EDGE_CURVE('',#12545,#12449,#6971,.T.);
#15747=EDGE_CURVE('',#12545,#12543,#6972,.T.);
#15748=EDGE_CURVE('',#12541,#12546,#6973,.T.);
#15749=EDGE_CURVE('',#12547,#12546,#6974,.T.);
#15750=EDGE_CURVE('',#12451,#12547,#6975,.T.);
#15751=EDGE_CURVE('',#12548,#12540,#6976,.T.);
#15752=EDGE_CURVE('',#12546,#12548,#6977,.T.);
#15753=EDGE_CURVE('',#12548,#12549,#6978,.T.);
#15754=EDGE_CURVE('',#12549,#12550,#6979,.T.);
#15755=EDGE_CURVE('',#12550,#12551,#6980,.T.);
#15756=EDGE_CURVE('',#12551,#12547,#6981,.T.);
#15757=EDGE_CURVE('',#12551,#12552,#6982,.T.);
#15758=EDGE_CURVE('',#12552,#12452,#6983,.T.);
#15759=EDGE_CURVE('',#12553,#12554,#6984,.T.);
#15760=EDGE_CURVE('',#12554,#12555,#6985,.T.);
#15761=EDGE_CURVE('',#12555,#12556,#6986,.T.);
#15762=EDGE_CURVE('',#12556,#12557,#6987,.T.);
#15763=EDGE_CURVE('',#12557,#12558,#6988,.T.);
#15764=EDGE_CURVE('',#12558,#12553,#6989,.T.);
#15765=EDGE_CURVE('',#12556,#12454,#6990,.T.);
#15766=EDGE_CURVE('',#12559,#12453,#6991,.T.);
#15767=EDGE_CURVE('',#12559,#12557,#6992,.T.);
#15768=EDGE_CURVE('',#12555,#12560,#6993,.T.);
#15769=EDGE_CURVE('',#12561,#12560,#6994,.T.);
#15770=EDGE_CURVE('',#12455,#12561,#6995,.T.);
#15771=EDGE_CURVE('',#12562,#12554,#6996,.T.);
#15772=EDGE_CURVE('',#12560,#12562,#6997,.T.);
#15773=EDGE_CURVE('',#12562,#12563,#6998,.T.);
#15774=EDGE_CURVE('',#12563,#12564,#6999,.T.);
#15775=EDGE_CURVE('',#12564,#12565,#7000,.T.);
#15776=EDGE_CURVE('',#12565,#12561,#7001,.T.);
#15777=EDGE_CURVE('',#12565,#12566,#7002,.T.);
#15778=EDGE_CURVE('',#12566,#12456,#7003,.T.);
#15779=EDGE_CURVE('',#12567,#12568,#7004,.T.);
#15780=EDGE_CURVE('',#12568,#12569,#7005,.T.);
#15781=EDGE_CURVE('',#12569,#12570,#7006,.T.);
#15782=EDGE_CURVE('',#12570,#12571,#7007,.T.);
#15783=EDGE_CURVE('',#12571,#12572,#7008,.T.);
#15784=EDGE_CURVE('',#12572,#12567,#7009,.T.);
#15785=EDGE_CURVE('',#12573,#12571,#7010,.T.);
#15786=EDGE_CURVE('',#12574,#12573,#7011,.T.);
#15787=EDGE_CURVE('',#12572,#12574,#7012,.T.);
#15788=EDGE_CURVE('',#12570,#12458,#7013,.T.);
#15789=EDGE_CURVE('',#12573,#12457,#7014,.T.);
#15790=EDGE_CURVE('',#12569,#12575,#7015,.T.);
#15791=EDGE_CURVE('',#12576,#12575,#7016,.T.);
#15792=EDGE_CURVE('',#12459,#12576,#7017,.T.);
#15793=EDGE_CURVE('',#12575,#12577,#7018,.T.);
#15794=EDGE_CURVE('',#12577,#12578,#7019,.T.);
#15795=EDGE_CURVE('',#12578,#12579,#7020,.T.);
#15796=EDGE_CURVE('',#12579,#12580,#7021,.T.);
#15797=EDGE_CURVE('',#12580,#12576,#7022,.T.);
#15798=EDGE_CURVE('',#12581,#12579,#7023,.T.);
#15799=EDGE_CURVE('',#12581,#12582,#7024,.T.);
#15800=EDGE_CURVE('',#12580,#12582,#7025,.T.);
#15801=EDGE_CURVE('',#12578,#12583,#7026,.T.);
#15802=EDGE_CURVE('',#12583,#12584,#7027,.T.);
#15803=EDGE_CURVE('',#12584,#12581,#7028,.T.);
#15804=EDGE_CURVE('',#12585,#12567,#7029,.T.);
#15805=EDGE_CURVE('',#12585,#12583,#7030,.T.);
#15806=EDGE_CURVE('',#12577,#12568,#7031,.T.);
#15807=EDGE_CURVE('',#12586,#12587,#7032,.T.);
#15808=EDGE_CURVE('',#12587,#12588,#7033,.T.);
#15809=EDGE_CURVE('',#12588,#12589,#7034,.T.);
#15810=EDGE_CURVE('',#12589,#12590,#7035,.T.);
#15811=EDGE_CURVE('',#12590,#12591,#7036,.T.);
#15812=EDGE_CURVE('',#12591,#12586,#7037,.T.);
#15813=EDGE_CURVE('',#12589,#12462,#7038,.T.);
#15814=EDGE_CURVE('',#12592,#12461,#7039,.T.);
#15815=EDGE_CURVE('',#12592,#12590,#7040,.T.);
#15816=EDGE_CURVE('',#12588,#12593,#7041,.T.);
#15817=EDGE_CURVE('',#12594,#12593,#7042,.T.);
#15818=EDGE_CURVE('',#12463,#12594,#7043,.T.);
#15819=EDGE_CURVE('',#12595,#12587,#7044,.T.);
#15820=EDGE_CURVE('',#12593,#12595,#7045,.T.);
#15821=EDGE_CURVE('',#12595,#12596,#7046,.T.);
#15822=EDGE_CURVE('',#12596,#12597,#7047,.T.);
#15823=EDGE_CURVE('',#12597,#12598,#7048,.T.);
#15824=EDGE_CURVE('',#12598,#12594,#7049,.T.);
#15825=EDGE_CURVE('',#12598,#12599,#7050,.T.);
#15826=EDGE_CURVE('',#12599,#12464,#7051,.T.);
#15827=EDGE_CURVE('',#12600,#12601,#7052,.T.);
#15828=EDGE_CURVE('',#12601,#12602,#7053,.T.);
#15829=EDGE_CURVE('',#12602,#12603,#7054,.T.);
#15830=EDGE_CURVE('',#12603,#12604,#7055,.T.);
#15831=EDGE_CURVE('',#12604,#12605,#7056,.T.);
#15832=EDGE_CURVE('',#12605,#12600,#7057,.T.);
#15833=EDGE_CURVE('',#12603,#12466,#7058,.T.);
#15834=EDGE_CURVE('',#12606,#12465,#7059,.T.);
#15835=EDGE_CURVE('',#12606,#12604,#7060,.T.);
#15836=EDGE_CURVE('',#12602,#12607,#7061,.T.);
#15837=EDGE_CURVE('',#12608,#12607,#7062,.T.);
#15838=EDGE_CURVE('',#12467,#12608,#7063,.T.);
#15839=EDGE_CURVE('',#12609,#12601,#7064,.T.);
#15840=EDGE_CURVE('',#12607,#12609,#7065,.T.);
#15841=EDGE_CURVE('',#12609,#12610,#7066,.T.);
#15842=EDGE_CURVE('',#12610,#12611,#7067,.T.);
#15843=EDGE_CURVE('',#12611,#12612,#7068,.T.);
#15844=EDGE_CURVE('',#12612,#12608,#7069,.T.);
#15845=EDGE_CURVE('',#12612,#12613,#7070,.T.);
#15846=EDGE_CURVE('',#12613,#12468,#7071,.T.);
#15847=EDGE_CURVE('',#12614,#12130,#7072,.T.);
#15848=EDGE_CURVE('',#12133,#12615,#7073,.T.);
#15849=EDGE_CURVE('',#12615,#12616,#7074,.T.);
#15850=EDGE_CURVE('',#12616,#12614,#7075,.T.);
#15851=EDGE_CURVE('',#12616,#12617,#7076,.T.);
#15852=EDGE_CURVE('',#12618,#12617,#7077,.T.);
#15853=EDGE_CURVE('',#12618,#12619,#7078,.T.);
#15854=EDGE_CURVE('',#12619,#12614,#7079,.T.);
#15855=EDGE_CURVE('',#12620,#12615,#7080,.T.);
#15856=EDGE_CURVE('',#12617,#12620,#7081,.T.);
#15857=EDGE_CURVE('',#12620,#12469,#7082,.T.);
#15858=EDGE_CURVE('',#12613,#12620,#7083,.T.);
#15859=EDGE_CURVE('',#12621,#12613,#7084,.T.);
#15860=EDGE_CURVE('',#12617,#12621,#7085,.T.);
#15861=EDGE_CURVE('',#12621,#12611,#7086,.T.);
#15862=EDGE_CURVE('',#12599,#12606,#7087,.T.);
#15863=EDGE_CURVE('',#12622,#12606,#7088,.T.);
#15864=EDGE_CURVE('',#12605,#12622,#7089,.T.);
#15865=EDGE_CURVE('',#12623,#12599,#7090,.T.);
#15866=EDGE_CURVE('',#12622,#12623,#7091,.T.);
#15867=EDGE_CURVE('',#12623,#12597,#7092,.T.);
#15868=EDGE_CURVE('',#12582,#12460,#7093,.T.);
#15869=EDGE_CURVE('',#12582,#12592,#7094,.T.);
#15870=EDGE_CURVE('',#12624,#12592,#7095,.T.);
#15871=EDGE_CURVE('',#12591,#12624,#7096,.T.);
#15872=EDGE_CURVE('',#12624,#12581,#7097,.T.);
#15873=EDGE_CURVE('',#12566,#12573,#7098,.T.);
#15874=EDGE_CURVE('',#12625,#12566,#7099,.T.);
#15875=EDGE_CURVE('',#12574,#12625,#7100,.T.);
#15876=EDGE_CURVE('',#12625,#12564,#7101,.T.);
#15877=EDGE_CURVE('',#12552,#12559,#7102,.T.);
#15878=EDGE_CURVE('',#12626,#12559,#7103,.T.);
#15879=EDGE_CURVE('',#12558,#12626,#7104,.T.);
#15880=EDGE_CURVE('',#12627,#12552,#7105,.T.);
#15881=EDGE_CURVE('',#12626,#12627,#7106,.T.);
#15882=EDGE_CURVE('',#12627,#12550,#7107,.T.);
#15883=EDGE_CURVE('',#12538,#12545,#7108,.T.);
#15884=EDGE_CURVE('',#12628,#12545,#7109,.T.);
#15885=EDGE_CURVE('',#12544,#12628,#7110,.T.);
#15886=EDGE_CURVE('',#12629,#12538,#7111,.T.);
#15887=EDGE_CURVE('',#12628,#12629,#7112,.T.);
#15888=EDGE_CURVE('',#12629,#12536,#7113,.T.);
#15889=EDGE_CURVE('',#12051,#12531,#7114,.T.);
#15890=EDGE_CURVE('',#12630,#12531,#7115,.T.);
#15891=EDGE_CURVE('',#12530,#12630,#7116,.T.);
#15892=EDGE_CURVE('',#12630,#12054,#7117,.T.);
#15893=EDGE_CURVE('',#12111,#12119,#7118,.T.);
#15894=EDGE_CURVE('',#12631,#12111,#7119,.T.);
#15895=EDGE_CURVE('',#12120,#12631,#7120,.T.);
#15896=EDGE_CURVE('',#12631,#12109,#7121,.T.);
#15897=EDGE_CURVE('',#12093,#12103,#7122,.T.);
#15898=EDGE_CURVE('',#12632,#12103,#7123,.T.);
#15899=EDGE_CURVE('',#12100,#12632,#7124,.T.);
#15900=EDGE_CURVE('',#12633,#12093,#7125,.T.);
#15901=EDGE_CURVE('',#12632,#12633,#7126,.T.);
#15902=EDGE_CURVE('',#12633,#12086,#7127,.T.);
#15903=EDGE_CURVE('',#12634,#12635,#7128,.T.);
#15904=EDGE_CURVE('',#12635,#12636,#7129,.T.);
#15905=EDGE_CURVE('',#12636,#12637,#7130,.T.);
#15906=EDGE_CURVE('',#12637,#12638,#7131,.T.);
#15907=EDGE_CURVE('',#12638,#12639,#7132,.T.);
#15908=EDGE_CURVE('',#12639,#12634,#7133,.T.);
#15909=EDGE_CURVE('',#12637,#12421,#7134,.T.);
#15910=EDGE_CURVE('',#12640,#12420,#7135,.T.);
#15911=EDGE_CURVE('',#12640,#12638,#7136,.T.);
#15912=EDGE_CURVE('',#12636,#12641,#7137,.T.);
#15913=EDGE_CURVE('',#12642,#12641,#7138,.T.);
#15914=EDGE_CURVE('',#12422,#12642,#7139,.T.);
#15915=EDGE_CURVE('',#12643,#12635,#7140,.T.);
#15916=EDGE_CURVE('',#12641,#12643,#7141,.T.);
#15917=EDGE_CURVE('',#12643,#12644,#7142,.T.);
#15918=EDGE_CURVE('',#12644,#12645,#7143,.T.);
#15919=EDGE_CURVE('',#12645,#12646,#7144,.T.);
#15920=EDGE_CURVE('',#12646,#12642,#7145,.T.);
#15921=EDGE_CURVE('',#12646,#12647,#7146,.T.);
#15922=EDGE_CURVE('',#12647,#12423,#7147,.T.);
#15923=EDGE_CURVE('',#12648,#12649,#7148,.T.);
#15924=EDGE_CURVE('',#12649,#12650,#7149,.T.);
#15925=EDGE_CURVE('',#12650,#12651,#7150,.T.);
#15926=EDGE_CURVE('',#12651,#12652,#7151,.T.);
#15927=EDGE_CURVE('',#12652,#12653,#7152,.T.);
#15928=EDGE_CURVE('',#12653,#12648,#7153,.T.);
#15929=EDGE_CURVE('',#12651,#12425,#7154,.T.);
#15930=EDGE_CURVE('',#12654,#12424,#7155,.T.);
#15931=EDGE_CURVE('',#12654,#12652,#7156,.T.);
#15932=EDGE_CURVE('',#12650,#12655,#7157,.T.);
#15933=EDGE_CURVE('',#12656,#12655,#7158,.T.);
#15934=EDGE_CURVE('',#12426,#12656,#7159,.T.);
#15935=EDGE_CURVE('',#12657,#12649,#7160,.T.);
#15936=EDGE_CURVE('',#12655,#12657,#7161,.T.);
#15937=EDGE_CURVE('',#12657,#12658,#7162,.T.);
#15938=EDGE_CURVE('',#12658,#12659,#7163,.T.);
#15939=EDGE_CURVE('',#12659,#12660,#7164,.T.);
#15940=EDGE_CURVE('',#12660,#12656,#7165,.T.);
#15941=EDGE_CURVE('',#12660,#12661,#7166,.T.);
#15942=EDGE_CURVE('',#12661,#12427,#7167,.T.);
#15943=EDGE_CURVE('',#12662,#12663,#7168,.T.);
#15944=EDGE_CURVE('',#12663,#12664,#7169,.T.);
#15945=EDGE_CURVE('',#12664,#12665,#7170,.T.);
#15946=EDGE_CURVE('',#12665,#12666,#7171,.T.);
#15947=EDGE_CURVE('',#12666,#12667,#7172,.T.);
#15948=EDGE_CURVE('',#12667,#12662,#7173,.T.);
#15949=EDGE_CURVE('',#12665,#12429,#7174,.T.);
#15950=EDGE_CURVE('',#12668,#12428,#7175,.T.);
#15951=EDGE_CURVE('',#12668,#12666,#7176,.T.);
#15952=EDGE_CURVE('',#12664,#12669,#7177,.T.);
#15953=EDGE_CURVE('',#12670,#12669,#7178,.T.);
#15954=EDGE_CURVE('',#12430,#12670,#7179,.T.);
#15955=EDGE_CURVE('',#12671,#12663,#7180,.T.);
#15956=EDGE_CURVE('',#12669,#12671,#7181,.T.);
#15957=EDGE_CURVE('',#12671,#12672,#7182,.T.);
#15958=EDGE_CURVE('',#12672,#12673,#7183,.T.);
#15959=EDGE_CURVE('',#12673,#12674,#7184,.T.);
#15960=EDGE_CURVE('',#12674,#12670,#7185,.T.);
#15961=EDGE_CURVE('',#12674,#12675,#7186,.T.);
#15962=EDGE_CURVE('',#12675,#12431,#7187,.T.);
#15963=EDGE_CURVE('',#12676,#12677,#7188,.T.);
#15964=EDGE_CURVE('',#12677,#12678,#7189,.T.);
#15965=EDGE_CURVE('',#12678,#12679,#7190,.T.);
#15966=EDGE_CURVE('',#12679,#12680,#7191,.T.);
#15967=EDGE_CURVE('',#12680,#12681,#7192,.T.);
#15968=EDGE_CURVE('',#12681,#12676,#7193,.T.);
#15969=EDGE_CURVE('',#12679,#12433,#7194,.T.);
#15970=EDGE_CURVE('',#12682,#12432,#7195,.T.);
#15971=EDGE_CURVE('',#12682,#12680,#7196,.T.);
#15972=EDGE_CURVE('',#12678,#12683,#7197,.T.);
#15973=EDGE_CURVE('',#12684,#12683,#7198,.T.);
#15974=EDGE_CURVE('',#12434,#12684,#7199,.T.);
#15975=EDGE_CURVE('',#12685,#12677,#7200,.T.);
#15976=EDGE_CURVE('',#12683,#12685,#7201,.T.);
#15977=EDGE_CURVE('',#12685,#12686,#7202,.T.);
#15978=EDGE_CURVE('',#12686,#12687,#7203,.T.);
#15979=EDGE_CURVE('',#12687,#12688,#7204,.T.);
#15980=EDGE_CURVE('',#12688,#12684,#7205,.T.);
#15981=EDGE_CURVE('',#12688,#12689,#7206,.T.);
#15982=EDGE_CURVE('',#12689,#12435,#7207,.T.);
#15983=EDGE_CURVE('',#12690,#12691,#7208,.T.);
#15984=EDGE_CURVE('',#12691,#12692,#7209,.T.);
#15985=EDGE_CURVE('',#12692,#12693,#7210,.T.);
#15986=EDGE_CURVE('',#12693,#12694,#7211,.T.);
#15987=EDGE_CURVE('',#12694,#12695,#7212,.T.);
#15988=EDGE_CURVE('',#12695,#12690,#7213,.T.);
#15989=EDGE_CURVE('',#12693,#12437,#7214,.T.);
#15990=EDGE_CURVE('',#12696,#12436,#7215,.T.);
#15991=EDGE_CURVE('',#12696,#12694,#7216,.T.);
#15992=EDGE_CURVE('',#12692,#12697,#7217,.T.);
#15993=EDGE_CURVE('',#12698,#12697,#7218,.T.);
#15994=EDGE_CURVE('',#12438,#12698,#7219,.T.);
#15995=EDGE_CURVE('',#12699,#12691,#7220,.T.);
#15996=EDGE_CURVE('',#12697,#12699,#7221,.T.);
#15997=EDGE_CURVE('',#12699,#12700,#7222,.T.);
#15998=EDGE_CURVE('',#12700,#12701,#7223,.T.);
#15999=EDGE_CURVE('',#12701,#12702,#7224,.T.);
#16000=EDGE_CURVE('',#12702,#12698,#7225,.T.);
#16001=EDGE_CURVE('',#12702,#12703,#7226,.T.);
#16002=EDGE_CURVE('',#12703,#12439,#7227,.T.);
#16003=EDGE_CURVE('',#12704,#12705,#7228,.T.);
#16004=EDGE_CURVE('',#12705,#12706,#7229,.T.);
#16005=EDGE_CURVE('',#12706,#12707,#7230,.T.);
#16006=EDGE_CURVE('',#12707,#12708,#7231,.T.);
#16007=EDGE_CURVE('',#12708,#12709,#7232,.T.);
#16008=EDGE_CURVE('',#12709,#12704,#7233,.T.);
#16009=EDGE_CURVE('',#12707,#12441,#7234,.T.);
#16010=EDGE_CURVE('',#12710,#12440,#7235,.T.);
#16011=EDGE_CURVE('',#12710,#12708,#7236,.T.);
#16012=EDGE_CURVE('',#12706,#12711,#7237,.T.);
#16013=EDGE_CURVE('',#12712,#12711,#7238,.T.);
#16014=EDGE_CURVE('',#12442,#12712,#7239,.T.);
#16015=EDGE_CURVE('',#12713,#12705,#7240,.T.);
#16016=EDGE_CURVE('',#12711,#12713,#7241,.T.);
#16017=EDGE_CURVE('',#12713,#12714,#7242,.T.);
#16018=EDGE_CURVE('',#12714,#12715,#7243,.T.);
#16019=EDGE_CURVE('',#12715,#12716,#7244,.T.);
#16020=EDGE_CURVE('',#12716,#12712,#7245,.T.);
#16021=EDGE_CURVE('',#12716,#12717,#7246,.T.);
#16022=EDGE_CURVE('',#12717,#12443,#7247,.T.);
#16023=EDGE_CURVE('',#12718,#12089,#7248,.T.);
#16024=EDGE_CURVE('',#12092,#12719,#7249,.T.);
#16025=EDGE_CURVE('',#12719,#12720,#7250,.T.);
#16026=EDGE_CURVE('',#12720,#12718,#7251,.T.);
#16027=EDGE_CURVE('',#12720,#12721,#7252,.T.);
#16028=EDGE_CURVE('',#12722,#12721,#7253,.T.);
#16029=EDGE_CURVE('',#12722,#12723,#7254,.T.);
#16030=EDGE_CURVE('',#12723,#12718,#7255,.T.);
#16031=EDGE_CURVE('',#12724,#12719,#7256,.T.);
#16032=EDGE_CURVE('',#12721,#12724,#7257,.T.);
#16033=EDGE_CURVE('',#12724,#12444,#7258,.T.);
#16034=EDGE_CURVE('',#12717,#12724,#7259,.T.);
#16035=EDGE_CURVE('',#12725,#12717,#7260,.T.);
#16036=EDGE_CURVE('',#12721,#12725,#7261,.T.);
#16037=EDGE_CURVE('',#12725,#12715,#7262,.T.);
#16038=EDGE_CURVE('',#12703,#12710,#7263,.T.);
#16039=EDGE_CURVE('',#12726,#12710,#7264,.T.);
#16040=EDGE_CURVE('',#12709,#12726,#7265,.T.);
#16041=EDGE_CURVE('',#12727,#12703,#7266,.T.);
#16042=EDGE_CURVE('',#12726,#12727,#7267,.T.);
#16043=EDGE_CURVE('',#12727,#12701,#7268,.T.);
#16044=EDGE_CURVE('',#12689,#12696,#7269,.T.);
#16045=EDGE_CURVE('',#12728,#12696,#7270,.T.);
#16046=EDGE_CURVE('',#12695,#12728,#7271,.T.);
#16047=EDGE_CURVE('',#12729,#12689,#7272,.T.);
#16048=EDGE_CURVE('',#12728,#12729,#7273,.T.);
#16049=EDGE_CURVE('',#12729,#12687,#7274,.T.);
#16050=EDGE_CURVE('',#12675,#12682,#7275,.T.);
#16051=EDGE_CURVE('',#12730,#12682,#7276,.T.);
#16052=EDGE_CURVE('',#12681,#12730,#7277,.T.);
#16053=EDGE_CURVE('',#12731,#12675,#7278,.T.);
#16054=EDGE_CURVE('',#12730,#12731,#7279,.T.);
#16055=EDGE_CURVE('',#12731,#12673,#7280,.T.);
#16056=EDGE_CURVE('',#12661,#12668,#7281,.T.);
#16057=EDGE_CURVE('',#12732,#12668,#7282,.T.);
#16058=EDGE_CURVE('',#12667,#12732,#7283,.T.);
#16059=EDGE_CURVE('',#12733,#12661,#7284,.T.);
#16060=EDGE_CURVE('',#12732,#12733,#7285,.T.);
#16061=EDGE_CURVE('',#12733,#12659,#7286,.T.);
#16062=EDGE_CURVE('',#12647,#12654,#7287,.T.);
#16063=EDGE_CURVE('',#12734,#12654,#7288,.T.);
#16064=EDGE_CURVE('',#12653,#12734,#7289,.T.);
#16065=EDGE_CURVE('',#12735,#12647,#7290,.T.);
#16066=EDGE_CURVE('',#12734,#12735,#7291,.T.);
#16067=EDGE_CURVE('',#12735,#12645,#7292,.T.);
#16068=EDGE_CURVE('',#12419,#12064,#7293,.F.);
#16069=EDGE_CURVE('',#12064,#12640,#7294,.T.);
#16070=EDGE_CURVE('',#12736,#12640,#7295,.T.);
#16071=EDGE_CURVE('',#12639,#12736,#7296,.T.);
#16072=EDGE_CURVE('',#12736,#12063,#7297,.T.);
#16073=EDGE_CURVE('',#12418,#12057,#7298,.T.);
#16074=EDGE_CURVE('',#12345,#12737,#7299,.T.);
#16075=EDGE_CURVE('',#12737,#12738,#7300,.T.);
#16076=EDGE_CURVE('',#12738,#12482,#7301,.T.);
#16077=EDGE_CURVE('',#12738,#12739,#7302,.T.);
#16078=EDGE_CURVE('',#12739,#12481,#7303,.T.);
#16079=EDGE_CURVE('',#12739,#12740,#7304,.T.);
#16080=EDGE_CURVE('',#12740,#12350,#7305,.T.);
#16081=EDGE_CURVE('',#12741,#12737,#7306,.T.);
#16082=EDGE_CURVE('',#12742,#12741,#7307,.T.);
#16083=EDGE_CURVE('',#12743,#12742,#7308,.T.);
#16084=EDGE_CURVE('',#12744,#12743,#7309,.T.);
#16085=EDGE_CURVE('',#12745,#12744,#7310,.T.);
#16086=EDGE_CURVE('',#12746,#12745,#7311,.T.);
#16087=EDGE_CURVE('',#12747,#12746,#7312,.T.);
#16088=EDGE_CURVE('',#12748,#12747,#7313,.T.);
#16089=EDGE_CURVE('',#12495,#12748,#7314,.T.);
#16090=EDGE_CURVE('',#12749,#12496,#7315,.T.);
#16091=EDGE_CURVE('',#12248,#12749,#7316,.T.);
#16092=EDGE_CURVE('',#12750,#12247,#7317,.T.);
#16093=EDGE_CURVE('',#12751,#12750,#7318,.T.);
#16094=EDGE_CURVE('',#12752,#12751,#7319,.T.);
#16095=EDGE_CURVE('',#12753,#12752,#7320,.T.);
#16096=EDGE_CURVE('',#12754,#12753,#7321,.T.);
#16097=EDGE_CURVE('',#12755,#12754,#7322,.T.);
#16098=EDGE_CURVE('',#12756,#12755,#7323,.T.);
#16099=EDGE_CURVE('',#12757,#12756,#7324,.T.);
#16100=EDGE_CURVE('',#12202,#12757,#7325,.T.);
#16101=EDGE_CURVE('',#12758,#12203,#7326,.T.);
#16102=EDGE_CURVE('',#12759,#12758,#7327,.T.);
#16103=EDGE_CURVE('',#12760,#12759,#7328,.T.);
#16104=EDGE_CURVE('',#12761,#12760,#7329,.T.);
#16105=EDGE_CURVE('',#12762,#12761,#7330,.T.);
#16106=EDGE_CURVE('',#12044,#12762,#7331,.T.);
#16107=EDGE_CURVE('',#12763,#12043,#7332,.T.);
#16108=EDGE_CURVE('',#12764,#12763,#7333,.T.);
#16109=EDGE_CURVE('',#12765,#12764,#7334,.T.);
#16110=EDGE_CURVE('',#12766,#12765,#7335,.T.);
#16111=EDGE_CURVE('',#12767,#12766,#7336,.T.);
#16112=EDGE_CURVE('',#12768,#12767,#7337,.T.);
#16113=EDGE_CURVE('',#12769,#12768,#7338,.T.);
#16114=EDGE_CURVE('',#12770,#12769,#7339,.T.);
#16115=EDGE_CURVE('',#12619,#12770,#7340,.T.);
#16116=EDGE_CURVE('',#12771,#12618,#7341,.T.);
#16117=EDGE_CURVE('',#12772,#12771,#7342,.T.);
#16118=EDGE_CURVE('',#12773,#12772,#7343,.T.);
#16119=EDGE_CURVE('',#12774,#12773,#7344,.T.);
#16120=EDGE_CURVE('',#12775,#12774,#7345,.T.);
#16121=EDGE_CURVE('',#12776,#12775,#7346,.T.);
#16122=EDGE_CURVE('',#12777,#12776,#7347,.T.);
#16123=EDGE_CURVE('',#12778,#12777,#7348,.T.);
#16124=EDGE_CURVE('',#12584,#12778,#7349,.T.);
#16125=EDGE_CURVE('',#12779,#12585,#7350,.T.);
#16126=EDGE_CURVE('',#12780,#12779,#7351,.T.);
#16127=EDGE_CURVE('',#12781,#12780,#7352,.T.);
#16128=EDGE_CURVE('',#12782,#12781,#7353,.T.);
#16129=EDGE_CURVE('',#12783,#12782,#7354,.T.);
#16130=EDGE_CURVE('',#12784,#12783,#7355,.T.);
#16131=EDGE_CURVE('',#12785,#12784,#7356,.T.);
#16132=EDGE_CURVE('',#12786,#12785,#7357,.T.);
#16133=EDGE_CURVE('',#12787,#12786,#7358,.T.);
#16134=EDGE_CURVE('',#12788,#12787,#7359,.T.);
#16135=EDGE_CURVE('',#12789,#12788,#7360,.T.);
#16136=EDGE_CURVE('',#12790,#12789,#7361,.T.);
#16137=EDGE_CURVE('',#12791,#12790,#7362,.T.);
#16138=EDGE_CURVE('',#12056,#12791,#7363,.T.);
#16139=EDGE_CURVE('',#12792,#12055,#7364,.T.);
#16140=EDGE_CURVE('',#12793,#12792,#7365,.T.);
#16141=EDGE_CURVE('',#12794,#12793,#7366,.T.);
#16142=EDGE_CURVE('',#12795,#12794,#7367,.T.);
#16143=EDGE_CURVE('',#12796,#12795,#7368,.T.);
#16144=EDGE_CURVE('',#12797,#12796,#7369,.T.);
#16145=EDGE_CURVE('',#12798,#12797,#7370,.T.);
#16146=EDGE_CURVE('',#12799,#12798,#7371,.T.);
#16147=EDGE_CURVE('',#12723,#12799,#7372,.T.);
#16148=EDGE_CURVE('',#12800,#12722,#7373,.T.);
#16149=EDGE_CURVE('',#12801,#12800,#7374,.T.);
#16150=EDGE_CURVE('',#12802,#12801,#7375,.T.);
#16151=EDGE_CURVE('',#12803,#12802,#7376,.T.);
#16152=EDGE_CURVE('',#12804,#12803,#7377,.T.);
#16153=EDGE_CURVE('',#12805,#12804,#7378,.T.);
#16154=EDGE_CURVE('',#12806,#12805,#7379,.T.);
#16155=EDGE_CURVE('',#12807,#12806,#7380,.T.);
#16156=EDGE_CURVE('',#12808,#12807,#7381,.T.);
#16157=EDGE_CURVE('',#12809,#12808,#7382,.T.);
#16158=EDGE_CURVE('',#12810,#12809,#7383,.T.);
#16159=EDGE_CURVE('',#12811,#12810,#7384,.T.);
#16160=EDGE_CURVE('',#12812,#12811,#7385,.T.);
#16161=EDGE_CURVE('',#12813,#12812,#7386,.T.);
#16162=EDGE_CURVE('',#12814,#12813,#7387,.T.);
#16163=EDGE_CURVE('',#12815,#12814,#7388,.T.);
#16164=EDGE_CURVE('',#12816,#12815,#7389,.T.);
#16165=EDGE_CURVE('',#12817,#12816,#7390,.T.);
#16166=EDGE_CURVE('',#12818,#12817,#7391,.T.);
#16167=EDGE_CURVE('',#12819,#12818,#7392,.T.);
#16168=EDGE_CURVE('',#12820,#12819,#7393,.T.);
#16169=EDGE_CURVE('',#12821,#12820,#7394,.T.);
#16170=EDGE_CURVE('',#12822,#12821,#7395,.T.);
#16171=EDGE_CURVE('',#12823,#12822,#7396,.T.);
#16172=EDGE_CURVE('',#12066,#12823,#7397,.T.);
#16173=EDGE_CURVE('',#12824,#12293,#7398,.T.);
#16174=EDGE_CURVE('',#12825,#12824,#7399,.T.);
#16175=EDGE_CURVE('',#12826,#12825,#7400,.T.);
#16176=EDGE_CURVE('',#12827,#12826,#7401,.T.);
#16177=EDGE_CURVE('',#12828,#12827,#7402,.T.);
#16178=EDGE_CURVE('',#12829,#12828,#7403,.T.);
#16179=EDGE_CURVE('',#12830,#12829,#7404,.T.);
#16180=EDGE_CURVE('',#12831,#12830,#7405,.T.);
#16181=EDGE_CURVE('',#12081,#12831,#7406,.T.);
#16182=EDGE_CURVE('',#12832,#12080,#7407,.T.);
#16183=EDGE_CURVE('',#12833,#12832,#7408,.T.);
#16184=EDGE_CURVE('',#12834,#12833,#7409,.T.);
#16185=EDGE_CURVE('',#12835,#12834,#7410,.T.);
#16186=EDGE_CURVE('',#12836,#12835,#7411,.T.);
#16187=EDGE_CURVE('',#12837,#12836,#7412,.T.);
#16188=EDGE_CURVE('',#12838,#12837,#7413,.T.);
#16189=EDGE_CURVE('',#12839,#12838,#7414,.T.);
#16190=EDGE_CURVE('',#12840,#12839,#7415,.T.);
#16191=EDGE_CURVE('',#12841,#12840,#7416,.T.);
#16192=EDGE_CURVE('',#12842,#12841,#7417,.T.);
#16193=EDGE_CURVE('',#12843,#12842,#7418,.T.);
#16194=EDGE_CURVE('',#12740,#12843,#7419,.T.);
#16195=EDGE_CURVE('',#12844,#12844,#10877,.T.);
#16196=EDGE_CURVE('',#12741,#12332,#7420,.T.);
#16197=EDGE_CURVE('',#12363,#12843,#7421,.T.);
#16198=EDGE_CURVE('',#12842,#12480,#7422,.T.);
#16199=EDGE_CURVE('',#12841,#12479,#7423,.T.);
#16200=EDGE_CURVE('',#12840,#12368,#7424,.T.);
#16201=EDGE_CURVE('',#12381,#12839,#7425,.T.);
#16202=EDGE_CURVE('',#12838,#12478,#7426,.T.);
#16203=EDGE_CURVE('',#12837,#12477,#7427,.T.);
#16204=EDGE_CURVE('',#12836,#12386,#7428,.T.);
#16205=EDGE_CURVE('',#12399,#12835,#7429,.T.);
#16206=EDGE_CURVE('',#12834,#12476,#7430,.T.);
#16207=EDGE_CURVE('',#12833,#12411,#7431,.T.);
#16208=EDGE_CURVE('',#12832,#12404,#7432,.T.);
#16209=EDGE_CURVE('',#12831,#12417,#7433,.T.);
#16210=EDGE_CURVE('',#12830,#12252,#7434,.T.);
#16211=EDGE_CURVE('',#12072,#12405,#7435,.T.);
#16212=EDGE_CURVE('',#12265,#12829,#7436,.T.);
#16213=EDGE_CURVE('',#12828,#12416,#7437,.T.);
#16214=EDGE_CURVE('',#12827,#12415,#7438,.T.);
#16215=EDGE_CURVE('',#12826,#12270,#7439,.T.);
#16216=EDGE_CURVE('',#12283,#12825,#7440,.T.);
#16217=EDGE_CURVE('',#12824,#12414,#7441,.F.);
#16218=EDGE_CURVE('',#12823,#12736,#7442,.T.);
#16219=EDGE_CURVE('',#12822,#12634,#7443,.T.);
#16220=EDGE_CURVE('',#12644,#12821,#7444,.T.);
#16221=EDGE_CURVE('',#12820,#12735,#7445,.T.);
#16222=EDGE_CURVE('',#12819,#12734,#7446,.T.);
#16223=EDGE_CURVE('',#12818,#12648,#7447,.T.);
#16224=EDGE_CURVE('',#12658,#12817,#7448,.T.);
#16225=EDGE_CURVE('',#12816,#12733,#7449,.T.);
#16226=EDGE_CURVE('',#12815,#12732,#7450,.T.);
#16227=EDGE_CURVE('',#12814,#12662,#7451,.T.);
#16228=EDGE_CURVE('',#12672,#12813,#7452,.T.);
#16229=EDGE_CURVE('',#12812,#12731,#7453,.T.);
#16230=EDGE_CURVE('',#12811,#12730,#7454,.T.);
#16231=EDGE_CURVE('',#12810,#12676,#7455,.T.);
#16232=EDGE_CURVE('',#12686,#12809,#7456,.T.);
#16233=EDGE_CURVE('',#12808,#12729,#7457,.T.);
#16234=EDGE_CURVE('',#12807,#12728,#7458,.T.);
#16235=EDGE_CURVE('',#12806,#12690,#7459,.T.);
#16236=EDGE_CURVE('',#12700,#12805,#7460,.T.);
#16237=EDGE_CURVE('',#12804,#12727,#7461,.T.);
#16238=EDGE_CURVE('',#12803,#12726,#7462,.T.);
#16239=EDGE_CURVE('',#12802,#12704,#7463,.T.);
#16240=EDGE_CURVE('',#12714,#12801,#7464,.T.);
#16241=EDGE_CURVE('',#12800,#12725,#7465,.T.);
#16242=EDGE_CURVE('',#12085,#12799,#7466,.T.);
#16243=EDGE_CURVE('',#12798,#12633,#7467,.T.);
#16244=EDGE_CURVE('',#12797,#12632,#7468,.T.);
#16245=EDGE_CURVE('',#12796,#12095,#7469,.T.);
#16246=EDGE_CURVE('',#12108,#12795,#7470,.T.);
#16247=EDGE_CURVE('',#12794,#12631,#7471,.T.);
#16248=EDGE_CURVE('',#12793,#12120,#7472,.T.);
#16249=EDGE_CURVE('',#12792,#12113,#7473,.T.);
#16250=EDGE_CURVE('',#12791,#12630,#7474,.T.);
#16251=EDGE_CURVE('',#12790,#12525,#7475,.T.);
#16252=EDGE_CURVE('',#12047,#12114,#7476,.T.);
#16253=EDGE_CURVE('',#12535,#12789,#7477,.T.);
#16254=EDGE_CURVE('',#12788,#12629,#7478,.T.);
#16255=EDGE_CURVE('',#12787,#12628,#7479,.T.);
#16256=EDGE_CURVE('',#12786,#12539,#7480,.T.);
#16257=EDGE_CURVE('',#12549,#12785,#7481,.T.);
#16258=EDGE_CURVE('',#12784,#12627,#7482,.T.);
#16259=EDGE_CURVE('',#12783,#12626,#7483,.T.);
#16260=EDGE_CURVE('',#12782,#12553,#7484,.T.);
#16261=EDGE_CURVE('',#12563,#12781,#7485,.T.);
#16262=EDGE_CURVE('',#12780,#12625,#7486,.T.);
#16263=EDGE_CURVE('',#12779,#12574,#7487,.F.);
#16264=EDGE_CURVE('',#12778,#12624,#7488,.T.);
#16265=EDGE_CURVE('',#12777,#12586,#7489,.T.);
#16266=EDGE_CURVE('',#12596,#12776,#7490,.T.);
#16267=EDGE_CURVE('',#12775,#12623,#7491,.T.);
#16268=EDGE_CURVE('',#12774,#12622,#7492,.T.);
#16269=EDGE_CURVE('',#12773,#12600,#7493,.T.);
#16270=EDGE_CURVE('',#12610,#12772,#7494,.T.);
#16271=EDGE_CURVE('',#12771,#12621,#7495,.T.);
#16272=EDGE_CURVE('',#12126,#12770,#7496,.T.);
#16273=EDGE_CURVE('',#12769,#12524,#7497,.T.);
#16274=EDGE_CURVE('',#12768,#12523,#7498,.T.);
#16275=EDGE_CURVE('',#12767,#12136,#7499,.T.);
#16276=EDGE_CURVE('',#12149,#12766,#7500,.T.);
#16277=EDGE_CURVE('',#12765,#12522,#7501,.T.);
#16278=EDGE_CURVE('',#12764,#12161,#7502,.T.);
#16279=EDGE_CURVE('',#12763,#12154,#7503,.T.);
#16280=EDGE_CURVE('',#12762,#12521,#7504,.T.);
#16281=EDGE_CURVE('',#12761,#12164,#7505,.T.);
#16282=EDGE_CURVE('',#12035,#12155,#7506,.T.);
#16283=EDGE_CURVE('',#12177,#12760,#7507,.T.);
#16284=EDGE_CURVE('',#12759,#12520,#7508,.F.);
#16285=EDGE_CURVE('',#12758,#12189,#7509,.T.);
#16286=EDGE_CURVE('',#12757,#12519,#7510,.T.);
#16287=EDGE_CURVE('',#12756,#12204,#7511,.T.);
#16288=EDGE_CURVE('',#12217,#12755,#7512,.T.);
#16289=EDGE_CURVE('',#12754,#12518,#7513,.T.);
#16290=EDGE_CURVE('',#12753,#12517,#7514,.T.);
#16291=EDGE_CURVE('',#12752,#12222,#7515,.T.);
#16292=EDGE_CURVE('',#12235,#12751,#7516,.T.);
#16293=EDGE_CURVE('',#12750,#12516,#7517,.T.);
#16294=EDGE_CURVE('',#12304,#12845,#7518,.T.);
#16295=EDGE_CURVE('',#12845,#12749,#7519,.T.);
#16296=EDGE_CURVE('',#12497,#12748,#7520,.T.);
#16297=EDGE_CURVE('',#12747,#12515,#7521,.T.);
#16298=EDGE_CURVE('',#12746,#12514,#7522,.T.);
#16299=EDGE_CURVE('',#12745,#12501,#7523,.T.);
#16300=EDGE_CURVE('',#12511,#12744,#7524,.T.);
#16301=EDGE_CURVE('',#12743,#12485,#7525,.T.);
#16302=EDGE_CURVE('',#12742,#12484,#7526,.T.);
#16303=EDGE_CURVE('',#12846,#12847,#7527,.T.);
#16304=EDGE_CURVE('',#12847,#12848,#1395,.T.);
#16305=EDGE_CURVE('',#12848,#12847,#1396,.T.);
#16306=EDGE_CURVE('',#12846,#12846,#1397,.T.);
#16307=EDGE_CURVE('',#12849,#12849,#10878,.T.);
#16308=EDGE_CURVE('',#12849,#12848,#7528,.T.);
#16309=EDGE_CURVE('',#12850,#12850,#10879,.T.);
#16310=EDGE_CURVE('',#12850,#12851,#7529,.T.);
#16311=EDGE_CURVE('',#12851,#12851,#10880,.T.);
#16312=EDGE_CURVE('',#12844,#12849,#7530,.T.);
#16313=EDGE_CURVE('',#12303,#12850,#7531,.T.);
#16314=EDGE_CURVE('',#12851,#12852,#7532,.T.);
#16315=EDGE_CURVE('',#12242,#12853,#7533,.T.);
#16316=EDGE_CURVE('',#12853,#12315,#7534,.T.);
#16317=EDGE_CURVE('',#12288,#12058,#7535,.T.);
#16318=EDGE_CURVE('',#12854,#12241,#7536,.T.);
#16319=EDGE_CURVE('',#12853,#12854,#7537,.T.);
#16320=EDGE_CURVE('',#12845,#12854,#7538,.T.);
#16321=EDGE_CURVE('',#12486,#12855,#7539,.T.);
#16322=EDGE_CURVE('',#12855,#12321,#7540,.T.);
#16323=EDGE_CURVE('',#12298,#12316,#7541,.T.);
#16324=EDGE_CURVE('',#12855,#12491,#7542,.T.);
#20340=ORIENTED_EDGE('',*,*,#15023,.T.);
#20341=ORIENTED_EDGE('',*,*,#15024,.T.);
#20342=ORIENTED_EDGE('',*,*,#15025,.T.);
#20343=ORIENTED_EDGE('',*,*,#15026,.T.);
#20344=ORIENTED_EDGE('',*,*,#15027,.T.);
#20345=ORIENTED_EDGE('',*,*,#15028,.T.);
#20346=ORIENTED_EDGE('',*,*,#15028,.F.);
#20347=ORIENTED_EDGE('',*,*,#15029,.T.);
#20348=ORIENTED_EDGE('',*,*,#15030,.F.);
#20349=ORIENTED_EDGE('',*,*,#15031,.T.);
#20350=ORIENTED_EDGE('',*,*,#15032,.T.);
#20351=ORIENTED_EDGE('',*,*,#15027,.F.);
#20352=ORIENTED_EDGE('',*,*,#15033,.F.);
#20353=ORIENTED_EDGE('',*,*,#15034,.T.);
#20354=ORIENTED_EDGE('',*,*,#15029,.F.);
#20355=ORIENTED_EDGE('',*,*,#15026,.F.);
#20356=ORIENTED_EDGE('',*,*,#15035,.T.);
#20357=ORIENTED_EDGE('',*,*,#15036,.T.);
#20358=ORIENTED_EDGE('',*,*,#15037,.T.);
#20359=ORIENTED_EDGE('',*,*,#15033,.T.);
#20360=ORIENTED_EDGE('',*,*,#15038,.T.);
#20361=ORIENTED_EDGE('',*,*,#15039,.T.);
#20362=ORIENTED_EDGE('',*,*,#15040,.T.);
#20363=ORIENTED_EDGE('',*,*,#15041,.T.);
#20364=ORIENTED_EDGE('',*,*,#15042,.T.);
#20365=ORIENTED_EDGE('',*,*,#15043,.T.);
#20366=ORIENTED_EDGE('',*,*,#15043,.F.);
#20367=ORIENTED_EDGE('',*,*,#15044,.T.);
#20368=ORIENTED_EDGE('',*,*,#15045,.F.);
#20369=ORIENTED_EDGE('',*,*,#15046,.T.);
#20370=ORIENTED_EDGE('',*,*,#15047,.T.);
#20371=ORIENTED_EDGE('',*,*,#15042,.F.);
#20372=ORIENTED_EDGE('',*,*,#15048,.F.);
#20373=ORIENTED_EDGE('',*,*,#15049,.T.);
#20374=ORIENTED_EDGE('',*,*,#15044,.F.);
#20375=ORIENTED_EDGE('',*,*,#15041,.F.);
#20376=ORIENTED_EDGE('',*,*,#15050,.T.);
#20377=ORIENTED_EDGE('',*,*,#15051,.T.);
#20378=ORIENTED_EDGE('',*,*,#15052,.T.);
#20379=ORIENTED_EDGE('',*,*,#15048,.T.);
#20380=ORIENTED_EDGE('',*,*,#15053,.T.);
#20381=ORIENTED_EDGE('',*,*,#15054,.T.);
#20382=ORIENTED_EDGE('',*,*,#15055,.T.);
#20383=ORIENTED_EDGE('',*,*,#15056,.T.);
#20384=ORIENTED_EDGE('',*,*,#15057,.T.);
#20385=ORIENTED_EDGE('',*,*,#15058,.T.);
#20386=ORIENTED_EDGE('',*,*,#15057,.F.);
#20387=ORIENTED_EDGE('',*,*,#15059,.F.);
#20388=ORIENTED_EDGE('',*,*,#15060,.T.);
#20389=ORIENTED_EDGE('',*,*,#15061,.F.);
#20390=ORIENTED_EDGE('',*,*,#15056,.F.);
#20391=ORIENTED_EDGE('',*,*,#15062,.T.);
#20392=ORIENTED_EDGE('',*,*,#15063,.T.);
#20393=ORIENTED_EDGE('',*,*,#15064,.T.);
#20394=ORIENTED_EDGE('',*,*,#15059,.T.);
#20395=ORIENTED_EDGE('',*,*,#15055,.F.);
#20396=ORIENTED_EDGE('',*,*,#15065,.T.);
#20397=ORIENTED_EDGE('',*,*,#15066,.F.);
#20398=ORIENTED_EDGE('',*,*,#15067,.F.);
#20399=ORIENTED_EDGE('',*,*,#15068,.T.);
#20400=ORIENTED_EDGE('',*,*,#15062,.F.);
#20401=ORIENTED_EDGE('',*,*,#15069,.T.);
#20402=ORIENTED_EDGE('',*,*,#15070,.T.);
#20403=ORIENTED_EDGE('',*,*,#15071,.T.);
#20404=ORIENTED_EDGE('',*,*,#15072,.T.);
#20405=ORIENTED_EDGE('',*,*,#15073,.T.);
#20406=ORIENTED_EDGE('',*,*,#15074,.T.);
#20407=ORIENTED_EDGE('',*,*,#15074,.F.);
#20408=ORIENTED_EDGE('',*,*,#15075,.T.);
#20409=ORIENTED_EDGE('',*,*,#15076,.F.);
#20410=ORIENTED_EDGE('',*,*,#15077,.T.);
#20411=ORIENTED_EDGE('',*,*,#15078,.T.);
#20412=ORIENTED_EDGE('',*,*,#15073,.F.);
#20413=ORIENTED_EDGE('',*,*,#15079,.F.);
#20414=ORIENTED_EDGE('',*,*,#15080,.T.);
#20415=ORIENTED_EDGE('',*,*,#15075,.F.);
#20416=ORIENTED_EDGE('',*,*,#15072,.F.);
#20417=ORIENTED_EDGE('',*,*,#15081,.T.);
#20418=ORIENTED_EDGE('',*,*,#15082,.T.);
#20419=ORIENTED_EDGE('',*,*,#15083,.T.);
#20420=ORIENTED_EDGE('',*,*,#15079,.T.);
#20421=ORIENTED_EDGE('',*,*,#15084,.T.);
#20422=ORIENTED_EDGE('',*,*,#15085,.T.);
#20423=ORIENTED_EDGE('',*,*,#15086,.T.);
#20424=ORIENTED_EDGE('',*,*,#15087,.T.);
#20425=ORIENTED_EDGE('',*,*,#15088,.T.);
#20426=ORIENTED_EDGE('',*,*,#15089,.T.);
#20427=ORIENTED_EDGE('',*,*,#15085,.F.);
#20428=ORIENTED_EDGE('',*,*,#15090,.F.);
#20429=ORIENTED_EDGE('',*,*,#15091,.F.);
#20430=ORIENTED_EDGE('',*,*,#15092,.F.);
#20431=ORIENTED_EDGE('',*,*,#15084,.F.);
#20432=ORIENTED_EDGE('',*,*,#15093,.F.);
#20433=ORIENTED_EDGE('',*,*,#15094,.T.);
#20434=ORIENTED_EDGE('',*,*,#15095,.F.);
#20435=ORIENTED_EDGE('',*,*,#15096,.F.);
#20436=ORIENTED_EDGE('',*,*,#15090,.T.);
#20437=ORIENTED_EDGE('',*,*,#15089,.F.);
#20438=ORIENTED_EDGE('',*,*,#15097,.T.);
#20439=ORIENTED_EDGE('',*,*,#15098,.T.);
#20440=ORIENTED_EDGE('',*,*,#15099,.T.);
#20441=ORIENTED_EDGE('',*,*,#15093,.T.);
#20442=ORIENTED_EDGE('',*,*,#15100,.T.);
#20443=ORIENTED_EDGE('',*,*,#15101,.T.);
#20444=ORIENTED_EDGE('',*,*,#15102,.T.);
#20445=ORIENTED_EDGE('',*,*,#15103,.T.);
#20446=ORIENTED_EDGE('',*,*,#15104,.T.);
#20447=ORIENTED_EDGE('',*,*,#15105,.T.);
#20448=ORIENTED_EDGE('',*,*,#15103,.F.);
#20449=ORIENTED_EDGE('',*,*,#15106,.T.);
#20450=ORIENTED_EDGE('',*,*,#15107,.T.);
#20451=ORIENTED_EDGE('',*,*,#15108,.F.);
#20452=ORIENTED_EDGE('',*,*,#15109,.T.);
#20453=ORIENTED_EDGE('',*,*,#15102,.F.);
#20454=ORIENTED_EDGE('',*,*,#15110,.T.);
#20455=ORIENTED_EDGE('',*,*,#15111,.F.);
#20456=ORIENTED_EDGE('',*,*,#15112,.F.);
#20457=ORIENTED_EDGE('',*,*,#15113,.T.);
#20458=ORIENTED_EDGE('',*,*,#15106,.F.);
#20459=ORIENTED_EDGE('',*,*,#15101,.F.);
#20460=ORIENTED_EDGE('',*,*,#15114,.F.);
#20461=ORIENTED_EDGE('',*,*,#15115,.F.);
#20462=ORIENTED_EDGE('',*,*,#15110,.F.);
#20463=ORIENTED_EDGE('',*,*,#15111,.T.);
#20464=ORIENTED_EDGE('',*,*,#15115,.T.);
#20465=ORIENTED_EDGE('',*,*,#15116,.T.);
#20466=ORIENTED_EDGE('',*,*,#15117,.T.);
#20467=ORIENTED_EDGE('',*,*,#15118,.T.);
#20468=ORIENTED_EDGE('',*,*,#15119,.T.);
#20469=ORIENTED_EDGE('',*,*,#15119,.F.);
#20470=ORIENTED_EDGE('',*,*,#15120,.T.);
#20471=ORIENTED_EDGE('',*,*,#15121,.T.);
#20472=ORIENTED_EDGE('',*,*,#15122,.T.);
#20473=ORIENTED_EDGE('',*,*,#15112,.T.);
#20474=ORIENTED_EDGE('',*,*,#15123,.T.);
#20475=ORIENTED_EDGE('',*,*,#15124,.T.);
#20476=ORIENTED_EDGE('',*,*,#15125,.T.);
#20477=ORIENTED_EDGE('',*,*,#15126,.T.);
#20478=ORIENTED_EDGE('',*,*,#15127,.T.);
#20479=ORIENTED_EDGE('',*,*,#15128,.T.);
#20480=ORIENTED_EDGE('',*,*,#15127,.F.);
#20481=ORIENTED_EDGE('',*,*,#15129,.F.);
#20482=ORIENTED_EDGE('',*,*,#15130,.F.);
#20483=ORIENTED_EDGE('',*,*,#15131,.F.);
#20484=ORIENTED_EDGE('',*,*,#15126,.F.);
#20485=ORIENTED_EDGE('',*,*,#15132,.T.);
#20486=ORIENTED_EDGE('',*,*,#15133,.T.);
#20487=ORIENTED_EDGE('',*,*,#15134,.F.);
#20488=ORIENTED_EDGE('',*,*,#15129,.T.);
#20489=ORIENTED_EDGE('',*,*,#15038,.F.);
#20490=ORIENTED_EDGE('',*,*,#15047,.F.);
#20491=ORIENTED_EDGE('',*,*,#15135,.T.);
#20492=ORIENTED_EDGE('',*,*,#15132,.F.);
#20493=ORIENTED_EDGE('',*,*,#15125,.F.);
#20494=ORIENTED_EDGE('',*,*,#15136,.T.);
#20495=ORIENTED_EDGE('',*,*,#15137,.T.);
#20496=ORIENTED_EDGE('',*,*,#15138,.T.);
#20497=ORIENTED_EDGE('',*,*,#15139,.T.);
#20498=ORIENTED_EDGE('',*,*,#15140,.T.);
#20499=ORIENTED_EDGE('',*,*,#15141,.T.);
#20500=ORIENTED_EDGE('',*,*,#15142,.T.);
#20501=ORIENTED_EDGE('',*,*,#15138,.F.);
#20502=ORIENTED_EDGE('',*,*,#15143,.F.);
#20503=ORIENTED_EDGE('',*,*,#15144,.F.);
#20504=ORIENTED_EDGE('',*,*,#15145,.F.);
#20505=ORIENTED_EDGE('',*,*,#15137,.F.);
#20506=ORIENTED_EDGE('',*,*,#15146,.F.);
#20507=ORIENTED_EDGE('',*,*,#15147,.T.);
#20508=ORIENTED_EDGE('',*,*,#15148,.F.);
#20509=ORIENTED_EDGE('',*,*,#15149,.F.);
#20510=ORIENTED_EDGE('',*,*,#15143,.T.);
#20511=ORIENTED_EDGE('',*,*,#15142,.F.);
#20512=ORIENTED_EDGE('',*,*,#15150,.T.);
#20513=ORIENTED_EDGE('',*,*,#15151,.T.);
#20514=ORIENTED_EDGE('',*,*,#15152,.T.);
#20515=ORIENTED_EDGE('',*,*,#15146,.T.);
#20516=ORIENTED_EDGE('',*,*,#15153,.T.);
#20517=ORIENTED_EDGE('',*,*,#15154,.T.);
#20518=ORIENTED_EDGE('',*,*,#15155,.T.);
#20519=ORIENTED_EDGE('',*,*,#15156,.T.);
#20520=ORIENTED_EDGE('',*,*,#15157,.T.);
#20521=ORIENTED_EDGE('',*,*,#15158,.T.);
#20522=ORIENTED_EDGE('',*,*,#15156,.F.);
#20523=ORIENTED_EDGE('',*,*,#15159,.T.);
#20524=ORIENTED_EDGE('',*,*,#15160,.T.);
#20525=ORIENTED_EDGE('',*,*,#15161,.F.);
#20526=ORIENTED_EDGE('',*,*,#15162,.T.);
#20527=ORIENTED_EDGE('',*,*,#15155,.F.);
#20528=ORIENTED_EDGE('',*,*,#15163,.T.);
#20529=ORIENTED_EDGE('',*,*,#15164,.F.);
#20530=ORIENTED_EDGE('',*,*,#15165,.F.);
#20531=ORIENTED_EDGE('',*,*,#15166,.T.);
#20532=ORIENTED_EDGE('',*,*,#15159,.F.);
#20533=ORIENTED_EDGE('',*,*,#15154,.F.);
#20534=ORIENTED_EDGE('',*,*,#15167,.F.);
#20535=ORIENTED_EDGE('',*,*,#15168,.F.);
#20536=ORIENTED_EDGE('',*,*,#15163,.F.);
#20537=ORIENTED_EDGE('',*,*,#15164,.T.);
#20538=ORIENTED_EDGE('',*,*,#15168,.T.);
#20539=ORIENTED_EDGE('',*,*,#15169,.T.);
#20540=ORIENTED_EDGE('',*,*,#15170,.T.);
#20541=ORIENTED_EDGE('',*,*,#15171,.T.);
#20542=ORIENTED_EDGE('',*,*,#15172,.T.);
#20543=ORIENTED_EDGE('',*,*,#15172,.F.);
#20544=ORIENTED_EDGE('',*,*,#15173,.T.);
#20545=ORIENTED_EDGE('',*,*,#15174,.T.);
#20546=ORIENTED_EDGE('',*,*,#15175,.T.);
#20547=ORIENTED_EDGE('',*,*,#15165,.T.);
#20548=ORIENTED_EDGE('',*,*,#15176,.T.);
#20549=ORIENTED_EDGE('',*,*,#15177,.T.);
#20550=ORIENTED_EDGE('',*,*,#15178,.T.);
#20551=ORIENTED_EDGE('',*,*,#15179,.T.);
#20552=ORIENTED_EDGE('',*,*,#15180,.T.);
#20553=ORIENTED_EDGE('',*,*,#15181,.T.);
#20554=ORIENTED_EDGE('',*,*,#15180,.F.);
#20555=ORIENTED_EDGE('',*,*,#15182,.F.);
#20556=ORIENTED_EDGE('',*,*,#15183,.F.);
#20557=ORIENTED_EDGE('',*,*,#15184,.F.);
#20558=ORIENTED_EDGE('',*,*,#15179,.F.);
#20559=ORIENTED_EDGE('',*,*,#15185,.T.);
#20560=ORIENTED_EDGE('',*,*,#15186,.T.);
#20561=ORIENTED_EDGE('',*,*,#15187,.F.);
#20562=ORIENTED_EDGE('',*,*,#15182,.T.);
#20563=ORIENTED_EDGE('',*,*,#15023,.F.);
#20564=ORIENTED_EDGE('',*,*,#15032,.F.);
#20565=ORIENTED_EDGE('',*,*,#15188,.T.);
#20566=ORIENTED_EDGE('',*,*,#15185,.F.);
#20567=ORIENTED_EDGE('',*,*,#15178,.F.);
#20568=ORIENTED_EDGE('',*,*,#15189,.T.);
#20569=ORIENTED_EDGE('',*,*,#15190,.T.);
#20570=ORIENTED_EDGE('',*,*,#15191,.T.);
#20571=ORIENTED_EDGE('',*,*,#15192,.T.);
#20572=ORIENTED_EDGE('',*,*,#15193,.T.);
#20573=ORIENTED_EDGE('',*,*,#15194,.T.);
#20574=ORIENTED_EDGE('',*,*,#15195,.T.);
#20575=ORIENTED_EDGE('',*,*,#15193,.F.);
#20576=ORIENTED_EDGE('',*,*,#15196,.T.);
#20577=ORIENTED_EDGE('',*,*,#15197,.T.);
#20578=ORIENTED_EDGE('',*,*,#15198,.F.);
#20579=ORIENTED_EDGE('',*,*,#15199,.T.);
#20580=ORIENTED_EDGE('',*,*,#15192,.F.);
#20581=ORIENTED_EDGE('',*,*,#15200,.T.);
#20582=ORIENTED_EDGE('',*,*,#15201,.F.);
#20583=ORIENTED_EDGE('',*,*,#15202,.F.);
#20584=ORIENTED_EDGE('',*,*,#15203,.T.);
#20585=ORIENTED_EDGE('',*,*,#15196,.F.);
#20586=ORIENTED_EDGE('',*,*,#15191,.F.);
#20587=ORIENTED_EDGE('',*,*,#15204,.F.);
#20588=ORIENTED_EDGE('',*,*,#15205,.F.);
#20589=ORIENTED_EDGE('',*,*,#15200,.F.);
#20590=ORIENTED_EDGE('',*,*,#15201,.T.);
#20591=ORIENTED_EDGE('',*,*,#15205,.T.);
#20592=ORIENTED_EDGE('',*,*,#15206,.T.);
#20593=ORIENTED_EDGE('',*,*,#15207,.T.);
#20594=ORIENTED_EDGE('',*,*,#15208,.T.);
#20595=ORIENTED_EDGE('',*,*,#15209,.T.);
#20596=ORIENTED_EDGE('',*,*,#15209,.F.);
#20597=ORIENTED_EDGE('',*,*,#15210,.T.);
#20598=ORIENTED_EDGE('',*,*,#15211,.T.);
#20599=ORIENTED_EDGE('',*,*,#15212,.T.);
#20600=ORIENTED_EDGE('',*,*,#15202,.T.);
#20601=ORIENTED_EDGE('',*,*,#15213,.T.);
#20602=ORIENTED_EDGE('',*,*,#15214,.T.);
#20603=ORIENTED_EDGE('',*,*,#15215,.T.);
#20604=ORIENTED_EDGE('',*,*,#15216,.T.);
#20605=ORIENTED_EDGE('',*,*,#15217,.T.);
#20606=ORIENTED_EDGE('',*,*,#15218,.T.);
#20607=ORIENTED_EDGE('',*,*,#15217,.F.);
#20608=ORIENTED_EDGE('',*,*,#15219,.F.);
#20609=ORIENTED_EDGE('',*,*,#15220,.F.);
#20610=ORIENTED_EDGE('',*,*,#15221,.F.);
#20611=ORIENTED_EDGE('',*,*,#15216,.F.);
#20612=ORIENTED_EDGE('',*,*,#15222,.T.);
#20613=ORIENTED_EDGE('',*,*,#15223,.T.);
#20614=ORIENTED_EDGE('',*,*,#15224,.F.);
#20615=ORIENTED_EDGE('',*,*,#15219,.T.);
#20616=ORIENTED_EDGE('',*,*,#15215,.F.);
#20617=ORIENTED_EDGE('',*,*,#15225,.T.);
#20618=ORIENTED_EDGE('',*,*,#15226,.F.);
#20619=ORIENTED_EDGE('',*,*,#15227,.F.);
#20620=ORIENTED_EDGE('',*,*,#15228,.T.);
#20621=ORIENTED_EDGE('',*,*,#15222,.F.);
#20622=ORIENTED_EDGE('',*,*,#15226,.T.);
#20623=ORIENTED_EDGE('',*,*,#15229,.T.);
#20624=ORIENTED_EDGE('',*,*,#15230,.T.);
#20625=ORIENTED_EDGE('',*,*,#15231,.T.);
#20626=ORIENTED_EDGE('',*,*,#15232,.T.);
#20627=ORIENTED_EDGE('',*,*,#15233,.T.);
#20628=ORIENTED_EDGE('',*,*,#15232,.F.);
#20629=ORIENTED_EDGE('',*,*,#15234,.F.);
#20630=ORIENTED_EDGE('',*,*,#15235,.T.);
#20631=ORIENTED_EDGE('',*,*,#15236,.F.);
#20632=ORIENTED_EDGE('',*,*,#15231,.F.);
#20633=ORIENTED_EDGE('',*,*,#15237,.T.);
#20634=ORIENTED_EDGE('',*,*,#15238,.T.);
#20635=ORIENTED_EDGE('',*,*,#15239,.T.);
#20636=ORIENTED_EDGE('',*,*,#15234,.T.);
#20637=ORIENTED_EDGE('',*,*,#15213,.F.);
#20638=ORIENTED_EDGE('',*,*,#15240,.F.);
#20639=ORIENTED_EDGE('',*,*,#15241,.T.);
#20640=ORIENTED_EDGE('',*,*,#15237,.F.);
#20641=ORIENTED_EDGE('',*,*,#15230,.F.);
#20642=ORIENTED_EDGE('',*,*,#15242,.T.);
#20643=ORIENTED_EDGE('',*,*,#15243,.T.);
#20644=ORIENTED_EDGE('',*,*,#15244,.T.);
#20645=ORIENTED_EDGE('',*,*,#15245,.T.);
#20646=ORIENTED_EDGE('',*,*,#15246,.T.);
#20647=ORIENTED_EDGE('',*,*,#15247,.T.);
#20648=ORIENTED_EDGE('',*,*,#15248,.T.);
#20649=ORIENTED_EDGE('',*,*,#15246,.F.);
#20650=ORIENTED_EDGE('',*,*,#15249,.T.);
#20651=ORIENTED_EDGE('',*,*,#15250,.T.);
#20652=ORIENTED_EDGE('',*,*,#15251,.F.);
#20653=ORIENTED_EDGE('',*,*,#15252,.T.);
#20654=ORIENTED_EDGE('',*,*,#15245,.F.);
#20655=ORIENTED_EDGE('',*,*,#15253,.T.);
#20656=ORIENTED_EDGE('',*,*,#15254,.F.);
#20657=ORIENTED_EDGE('',*,*,#15255,.F.);
#20658=ORIENTED_EDGE('',*,*,#15256,.T.);
#20659=ORIENTED_EDGE('',*,*,#15249,.F.);
#20660=ORIENTED_EDGE('',*,*,#15244,.F.);
#20661=ORIENTED_EDGE('',*,*,#15257,.F.);
#20662=ORIENTED_EDGE('',*,*,#15258,.F.);
#20663=ORIENTED_EDGE('',*,*,#15253,.F.);
#20664=ORIENTED_EDGE('',*,*,#15254,.T.);
#20665=ORIENTED_EDGE('',*,*,#15258,.T.);
#20666=ORIENTED_EDGE('',*,*,#15259,.T.);
#20667=ORIENTED_EDGE('',*,*,#15260,.T.);
#20668=ORIENTED_EDGE('',*,*,#15261,.T.);
#20669=ORIENTED_EDGE('',*,*,#15262,.T.);
#20670=ORIENTED_EDGE('',*,*,#15262,.F.);
#20671=ORIENTED_EDGE('',*,*,#15263,.T.);
#20672=ORIENTED_EDGE('',*,*,#15264,.T.);
#20673=ORIENTED_EDGE('',*,*,#15265,.T.);
#20674=ORIENTED_EDGE('',*,*,#15255,.T.);
#20675=ORIENTED_EDGE('',*,*,#15266,.T.);
#20676=ORIENTED_EDGE('',*,*,#15267,.T.);
#20677=ORIENTED_EDGE('',*,*,#15268,.T.);
#20678=ORIENTED_EDGE('',*,*,#15269,.T.);
#20679=ORIENTED_EDGE('',*,*,#15270,.T.);
#20680=ORIENTED_EDGE('',*,*,#15271,.T.);
#20681=ORIENTED_EDGE('',*,*,#15269,.F.);
#20682=ORIENTED_EDGE('',*,*,#15272,.T.);
#20683=ORIENTED_EDGE('',*,*,#15273,.T.);
#20684=ORIENTED_EDGE('',*,*,#15274,.F.);
#20685=ORIENTED_EDGE('',*,*,#15275,.T.);
#20686=ORIENTED_EDGE('',*,*,#15268,.F.);
#20687=ORIENTED_EDGE('',*,*,#15276,.T.);
#20688=ORIENTED_EDGE('',*,*,#15277,.F.);
#20689=ORIENTED_EDGE('',*,*,#15278,.F.);
#20690=ORIENTED_EDGE('',*,*,#15279,.T.);
#20691=ORIENTED_EDGE('',*,*,#15272,.F.);
#20692=ORIENTED_EDGE('',*,*,#15267,.F.);
#20693=ORIENTED_EDGE('',*,*,#15280,.F.);
#20694=ORIENTED_EDGE('',*,*,#15281,.F.);
#20695=ORIENTED_EDGE('',*,*,#15276,.F.);
#20696=ORIENTED_EDGE('',*,*,#15277,.T.);
#20697=ORIENTED_EDGE('',*,*,#15281,.T.);
#20698=ORIENTED_EDGE('',*,*,#15282,.T.);
#20699=ORIENTED_EDGE('',*,*,#15283,.T.);
#20700=ORIENTED_EDGE('',*,*,#15284,.T.);
#20701=ORIENTED_EDGE('',*,*,#15285,.T.);
#20702=ORIENTED_EDGE('',*,*,#15285,.F.);
#20703=ORIENTED_EDGE('',*,*,#15286,.T.);
#20704=ORIENTED_EDGE('',*,*,#15287,.T.);
#20705=ORIENTED_EDGE('',*,*,#15288,.T.);
#20706=ORIENTED_EDGE('',*,*,#15278,.T.);
#20707=ORIENTED_EDGE('',*,*,#15289,.T.);
#20708=ORIENTED_EDGE('',*,*,#15290,.T.);
#20709=ORIENTED_EDGE('',*,*,#15291,.T.);
#20710=ORIENTED_EDGE('',*,*,#15292,.T.);
#20711=ORIENTED_EDGE('',*,*,#15293,.T.);
#20712=ORIENTED_EDGE('',*,*,#15294,.T.);
#20713=ORIENTED_EDGE('',*,*,#15294,.F.);
#20714=ORIENTED_EDGE('',*,*,#15295,.T.);
#20715=ORIENTED_EDGE('',*,*,#15296,.F.);
#20716=ORIENTED_EDGE('',*,*,#15297,.T.);
#20717=ORIENTED_EDGE('',*,*,#15298,.T.);
#20718=ORIENTED_EDGE('',*,*,#15293,.F.);
#20719=ORIENTED_EDGE('',*,*,#15299,.F.);
#20720=ORIENTED_EDGE('',*,*,#15300,.F.);
#20721=ORIENTED_EDGE('',*,*,#15295,.F.);
#20722=ORIENTED_EDGE('',*,*,#15292,.F.);
#20723=ORIENTED_EDGE('',*,*,#15301,.T.);
#20724=ORIENTED_EDGE('',*,*,#15302,.T.);
#20725=ORIENTED_EDGE('',*,*,#15303,.F.);
#20726=ORIENTED_EDGE('',*,*,#15299,.T.);
#20727=ORIENTED_EDGE('',*,*,#15304,.T.);
#20728=ORIENTED_EDGE('',*,*,#15305,.T.);
#20729=ORIENTED_EDGE('',*,*,#15306,.T.);
#20730=ORIENTED_EDGE('',*,*,#15307,.T.);
#20731=ORIENTED_EDGE('',*,*,#15308,.T.);
#20732=ORIENTED_EDGE('',*,*,#15309,.T.);
#20733=ORIENTED_EDGE('',*,*,#15307,.F.);
#20734=ORIENTED_EDGE('',*,*,#15310,.T.);
#20735=ORIENTED_EDGE('',*,*,#15311,.T.);
#20736=ORIENTED_EDGE('',*,*,#15312,.F.);
#20737=ORIENTED_EDGE('',*,*,#15313,.T.);
#20738=ORIENTED_EDGE('',*,*,#15306,.F.);
#20739=ORIENTED_EDGE('',*,*,#15314,.T.);
#20740=ORIENTED_EDGE('',*,*,#15315,.F.);
#20741=ORIENTED_EDGE('',*,*,#15316,.F.);
#20742=ORIENTED_EDGE('',*,*,#15317,.T.);
#20743=ORIENTED_EDGE('',*,*,#15310,.F.);
#20744=ORIENTED_EDGE('',*,*,#15305,.F.);
#20745=ORIENTED_EDGE('',*,*,#15318,.F.);
#20746=ORIENTED_EDGE('',*,*,#15319,.F.);
#20747=ORIENTED_EDGE('',*,*,#15314,.F.);
#20748=ORIENTED_EDGE('',*,*,#15315,.T.);
#20749=ORIENTED_EDGE('',*,*,#15319,.T.);
#20750=ORIENTED_EDGE('',*,*,#15320,.T.);
#20751=ORIENTED_EDGE('',*,*,#15321,.T.);
#20752=ORIENTED_EDGE('',*,*,#15322,.T.);
#20753=ORIENTED_EDGE('',*,*,#15323,.T.);
#20754=ORIENTED_EDGE('',*,*,#15323,.F.);
#20755=ORIENTED_EDGE('',*,*,#15324,.T.);
#20756=ORIENTED_EDGE('',*,*,#15325,.T.);
#20757=ORIENTED_EDGE('',*,*,#15326,.T.);
#20758=ORIENTED_EDGE('',*,*,#15316,.T.);
#20759=ORIENTED_EDGE('',*,*,#15327,.T.);
#20760=ORIENTED_EDGE('',*,*,#15328,.T.);
#20761=ORIENTED_EDGE('',*,*,#15329,.T.);
#20762=ORIENTED_EDGE('',*,*,#15330,.T.);
#20763=ORIENTED_EDGE('',*,*,#15331,.T.);
#20764=ORIENTED_EDGE('',*,*,#15332,.T.);
#20765=ORIENTED_EDGE('',*,*,#15330,.F.);
#20766=ORIENTED_EDGE('',*,*,#15333,.T.);
#20767=ORIENTED_EDGE('',*,*,#15334,.T.);
#20768=ORIENTED_EDGE('',*,*,#15335,.F.);
#20769=ORIENTED_EDGE('',*,*,#15336,.T.);
#20770=ORIENTED_EDGE('',*,*,#15329,.F.);
#20771=ORIENTED_EDGE('',*,*,#15337,.T.);
#20772=ORIENTED_EDGE('',*,*,#15338,.F.);
#20773=ORIENTED_EDGE('',*,*,#15339,.F.);
#20774=ORIENTED_EDGE('',*,*,#15340,.T.);
#20775=ORIENTED_EDGE('',*,*,#15333,.F.);
#20776=ORIENTED_EDGE('',*,*,#15328,.F.);
#20777=ORIENTED_EDGE('',*,*,#15341,.F.);
#20778=ORIENTED_EDGE('',*,*,#15342,.F.);
#20779=ORIENTED_EDGE('',*,*,#15337,.F.);
#20780=ORIENTED_EDGE('',*,*,#15338,.T.);
#20781=ORIENTED_EDGE('',*,*,#15342,.T.);
#20782=ORIENTED_EDGE('',*,*,#15343,.T.);
#20783=ORIENTED_EDGE('',*,*,#15344,.T.);
#20784=ORIENTED_EDGE('',*,*,#15345,.T.);
#20785=ORIENTED_EDGE('',*,*,#15346,.T.);
#20786=ORIENTED_EDGE('',*,*,#15346,.F.);
#20787=ORIENTED_EDGE('',*,*,#15347,.T.);
#20788=ORIENTED_EDGE('',*,*,#15348,.T.);
#20789=ORIENTED_EDGE('',*,*,#15349,.T.);
#20790=ORIENTED_EDGE('',*,*,#15339,.T.);
#20791=ORIENTED_EDGE('',*,*,#15066,.T.);
#20792=ORIENTED_EDGE('',*,*,#15350,.T.);
#20793=ORIENTED_EDGE('',*,*,#15351,.T.);
#20794=ORIENTED_EDGE('',*,*,#15352,.T.);
#20795=ORIENTED_EDGE('',*,*,#15353,.T.);
#20796=ORIENTED_EDGE('',*,*,#15354,.T.);
#20797=ORIENTED_EDGE('',*,*,#15354,.F.);
#20798=ORIENTED_EDGE('',*,*,#15355,.T.);
#20799=ORIENTED_EDGE('',*,*,#15356,.F.);
#20800=ORIENTED_EDGE('',*,*,#15357,.T.);
#20801=ORIENTED_EDGE('',*,*,#15067,.T.);
#20802=ORIENTED_EDGE('',*,*,#15353,.F.);
#20803=ORIENTED_EDGE('',*,*,#15358,.F.);
#20804=ORIENTED_EDGE('',*,*,#15359,.F.);
#20805=ORIENTED_EDGE('',*,*,#15355,.F.);
#20806=ORIENTED_EDGE('',*,*,#15352,.F.);
#20807=ORIENTED_EDGE('',*,*,#15360,.T.);
#20808=ORIENTED_EDGE('',*,*,#15361,.T.);
#20809=ORIENTED_EDGE('',*,*,#15362,.F.);
#20810=ORIENTED_EDGE('',*,*,#15358,.T.);
#20811=ORIENTED_EDGE('',*,*,#15363,.T.);
#20812=ORIENTED_EDGE('',*,*,#15364,.T.);
#20813=ORIENTED_EDGE('',*,*,#15365,.T.);
#20814=ORIENTED_EDGE('',*,*,#15366,.T.);
#20815=ORIENTED_EDGE('',*,*,#15366,.F.);
#20816=ORIENTED_EDGE('',*,*,#15367,.F.);
#20817=ORIENTED_EDGE('',*,*,#15368,.F.);
#20818=ORIENTED_EDGE('',*,*,#15369,.F.);
#20819=ORIENTED_EDGE('',*,*,#15370,.F.);
#20820=ORIENTED_EDGE('',*,*,#15365,.F.);
#20821=ORIENTED_EDGE('',*,*,#15371,.T.);
#20822=ORIENTED_EDGE('',*,*,#15372,.F.);
#20823=ORIENTED_EDGE('',*,*,#15373,.F.);
#20824=ORIENTED_EDGE('',*,*,#15374,.F.);
#20825=ORIENTED_EDGE('',*,*,#15367,.T.);
#20826=ORIENTED_EDGE('',*,*,#15375,.T.);
#20827=ORIENTED_EDGE('',*,*,#15376,.T.);
#20828=ORIENTED_EDGE('',*,*,#15377,.T.);
#20829=ORIENTED_EDGE('',*,*,#15378,.T.);
#20830=ORIENTED_EDGE('',*,*,#15379,.T.);
#20831=ORIENTED_EDGE('',*,*,#15380,.T.);
#20832=ORIENTED_EDGE('',*,*,#15376,.F.);
#20833=ORIENTED_EDGE('',*,*,#15381,.T.);
#20834=ORIENTED_EDGE('',*,*,#15382,.F.);
#20835=ORIENTED_EDGE('',*,*,#15373,.T.);
#20836=ORIENTED_EDGE('',*,*,#15375,.F.);
#20837=ORIENTED_EDGE('',*,*,#15383,.T.);
#20838=ORIENTED_EDGE('',*,*,#15384,.T.);
#20839=ORIENTED_EDGE('',*,*,#15385,.T.);
#20840=ORIENTED_EDGE('',*,*,#15386,.T.);
#20841=ORIENTED_EDGE('',*,*,#15387,.T.);
#20842=ORIENTED_EDGE('',*,*,#15380,.F.);
#20843=ORIENTED_EDGE('',*,*,#15388,.T.);
#20844=ORIENTED_EDGE('',*,*,#15389,.F.);
#20845=ORIENTED_EDGE('',*,*,#15390,.F.);
#20846=ORIENTED_EDGE('',*,*,#15391,.T.);
#20847=ORIENTED_EDGE('',*,*,#15383,.F.);
#20848=ORIENTED_EDGE('',*,*,#15374,.T.);
#20849=ORIENTED_EDGE('',*,*,#15382,.T.);
#20850=ORIENTED_EDGE('',*,*,#15392,.T.);
#20851=ORIENTED_EDGE('',*,*,#15368,.T.);
#20852=ORIENTED_EDGE('',*,*,#15393,.T.);
#20853=ORIENTED_EDGE('',*,*,#15394,.T.);
#20854=ORIENTED_EDGE('',*,*,#15395,.T.);
#20855=ORIENTED_EDGE('',*,*,#15396,.T.);
#20856=ORIENTED_EDGE('',*,*,#15397,.T.);
#20857=ORIENTED_EDGE('',*,*,#15398,.T.);
#20858=ORIENTED_EDGE('',*,*,#15393,.F.);
#20859=ORIENTED_EDGE('',*,*,#15399,.T.);
#20860=ORIENTED_EDGE('',*,*,#15400,.T.);
#20861=ORIENTED_EDGE('',*,*,#15390,.T.);
#20862=ORIENTED_EDGE('',*,*,#15401,.F.);
#20863=ORIENTED_EDGE('',*,*,#15402,.T.);
#20864=ORIENTED_EDGE('',*,*,#15398,.F.);
#20865=ORIENTED_EDGE('',*,*,#15403,.T.);
#20866=ORIENTED_EDGE('',*,*,#15404,.F.);
#20867=ORIENTED_EDGE('',*,*,#15405,.F.);
#20868=ORIENTED_EDGE('',*,*,#15406,.T.);
#20869=ORIENTED_EDGE('',*,*,#15399,.F.);
#20870=ORIENTED_EDGE('',*,*,#15397,.F.);
#20871=ORIENTED_EDGE('',*,*,#15407,.F.);
#20872=ORIENTED_EDGE('',*,*,#15408,.F.);
#20873=ORIENTED_EDGE('',*,*,#15403,.F.);
#20874=ORIENTED_EDGE('',*,*,#15409,.T.);
#20875=ORIENTED_EDGE('',*,*,#15410,.T.);
#20876=ORIENTED_EDGE('',*,*,#15411,.T.);
#20877=ORIENTED_EDGE('',*,*,#15412,.T.);
#20878=ORIENTED_EDGE('',*,*,#15413,.T.);
#20879=ORIENTED_EDGE('',*,*,#15414,.T.);
#20880=ORIENTED_EDGE('',*,*,#15412,.F.);
#20881=ORIENTED_EDGE('',*,*,#15415,.T.);
#20882=ORIENTED_EDGE('',*,*,#15416,.T.);
#20883=ORIENTED_EDGE('',*,*,#15417,.F.);
#20884=ORIENTED_EDGE('',*,*,#15418,.T.);
#20885=ORIENTED_EDGE('',*,*,#15411,.F.);
#20886=ORIENTED_EDGE('',*,*,#15419,.T.);
#20887=ORIENTED_EDGE('',*,*,#15420,.F.);
#20888=ORIENTED_EDGE('',*,*,#15421,.F.);
#20889=ORIENTED_EDGE('',*,*,#15422,.T.);
#20890=ORIENTED_EDGE('',*,*,#15415,.F.);
#20891=ORIENTED_EDGE('',*,*,#15410,.F.);
#20892=ORIENTED_EDGE('',*,*,#15423,.F.);
#20893=ORIENTED_EDGE('',*,*,#15424,.F.);
#20894=ORIENTED_EDGE('',*,*,#15419,.F.);
#20895=ORIENTED_EDGE('',*,*,#15420,.T.);
#20896=ORIENTED_EDGE('',*,*,#15424,.T.);
#20897=ORIENTED_EDGE('',*,*,#15425,.T.);
#20898=ORIENTED_EDGE('',*,*,#15426,.T.);
#20899=ORIENTED_EDGE('',*,*,#15427,.T.);
#20900=ORIENTED_EDGE('',*,*,#15428,.T.);
#20901=ORIENTED_EDGE('',*,*,#15428,.F.);
#20902=ORIENTED_EDGE('',*,*,#15429,.T.);
#20903=ORIENTED_EDGE('',*,*,#15430,.T.);
#20904=ORIENTED_EDGE('',*,*,#15431,.T.);
#20905=ORIENTED_EDGE('',*,*,#15421,.T.);
#20906=ORIENTED_EDGE('',*,*,#15432,.T.);
#20907=ORIENTED_EDGE('',*,*,#15433,.T.);
#20908=ORIENTED_EDGE('',*,*,#15434,.T.);
#20909=ORIENTED_EDGE('',*,*,#15435,.T.);
#20910=ORIENTED_EDGE('',*,*,#15436,.T.);
#20911=ORIENTED_EDGE('',*,*,#15437,.T.);
#20912=ORIENTED_EDGE('',*,*,#15435,.F.);
#20913=ORIENTED_EDGE('',*,*,#15438,.T.);
#20914=ORIENTED_EDGE('',*,*,#15439,.T.);
#20915=ORIENTED_EDGE('',*,*,#15440,.F.);
#20916=ORIENTED_EDGE('',*,*,#15441,.T.);
#20917=ORIENTED_EDGE('',*,*,#15434,.F.);
#20918=ORIENTED_EDGE('',*,*,#15442,.T.);
#20919=ORIENTED_EDGE('',*,*,#15443,.F.);
#20920=ORIENTED_EDGE('',*,*,#15444,.F.);
#20921=ORIENTED_EDGE('',*,*,#15445,.T.);
#20922=ORIENTED_EDGE('',*,*,#15438,.F.);
#20923=ORIENTED_EDGE('',*,*,#15433,.F.);
#20924=ORIENTED_EDGE('',*,*,#15446,.F.);
#20925=ORIENTED_EDGE('',*,*,#15447,.F.);
#20926=ORIENTED_EDGE('',*,*,#15442,.F.);
#20927=ORIENTED_EDGE('',*,*,#15443,.T.);
#20928=ORIENTED_EDGE('',*,*,#15447,.T.);
#20929=ORIENTED_EDGE('',*,*,#15448,.T.);
#20930=ORIENTED_EDGE('',*,*,#15449,.T.);
#20931=ORIENTED_EDGE('',*,*,#15450,.T.);
#20932=ORIENTED_EDGE('',*,*,#15451,.T.);
#20933=ORIENTED_EDGE('',*,*,#15451,.F.);
#20934=ORIENTED_EDGE('',*,*,#15452,.T.);
#20935=ORIENTED_EDGE('',*,*,#15453,.T.);
#20936=ORIENTED_EDGE('',*,*,#15454,.T.);
#20937=ORIENTED_EDGE('',*,*,#15444,.T.);
#20938=ORIENTED_EDGE('',*,*,#15455,.T.);
#20939=ORIENTED_EDGE('',*,*,#15456,.T.);
#20940=ORIENTED_EDGE('',*,*,#15457,.T.);
#20941=ORIENTED_EDGE('',*,*,#15458,.T.);
#20942=ORIENTED_EDGE('',*,*,#15459,.T.);
#20943=ORIENTED_EDGE('',*,*,#15460,.T.);
#20944=ORIENTED_EDGE('',*,*,#15458,.F.);
#20945=ORIENTED_EDGE('',*,*,#15461,.T.);
#20946=ORIENTED_EDGE('',*,*,#15462,.T.);
#20947=ORIENTED_EDGE('',*,*,#15463,.F.);
#20948=ORIENTED_EDGE('',*,*,#15464,.T.);
#20949=ORIENTED_EDGE('',*,*,#15457,.F.);
#20950=ORIENTED_EDGE('',*,*,#15465,.T.);
#20951=ORIENTED_EDGE('',*,*,#15466,.F.);
#20952=ORIENTED_EDGE('',*,*,#15467,.F.);
#20953=ORIENTED_EDGE('',*,*,#15468,.T.);
#20954=ORIENTED_EDGE('',*,*,#15461,.F.);
#20955=ORIENTED_EDGE('',*,*,#15456,.F.);
#20956=ORIENTED_EDGE('',*,*,#15469,.F.);
#20957=ORIENTED_EDGE('',*,*,#15470,.F.);
#20958=ORIENTED_EDGE('',*,*,#15465,.F.);
#20959=ORIENTED_EDGE('',*,*,#15466,.T.);
#20960=ORIENTED_EDGE('',*,*,#15470,.T.);
#20961=ORIENTED_EDGE('',*,*,#15471,.T.);
#20962=ORIENTED_EDGE('',*,*,#15472,.T.);
#20963=ORIENTED_EDGE('',*,*,#15473,.T.);
#20964=ORIENTED_EDGE('',*,*,#15474,.T.);
#20965=ORIENTED_EDGE('',*,*,#15474,.F.);
#20966=ORIENTED_EDGE('',*,*,#15475,.T.);
#20967=ORIENTED_EDGE('',*,*,#15476,.T.);
#20968=ORIENTED_EDGE('',*,*,#15477,.T.);
#20969=ORIENTED_EDGE('',*,*,#15467,.T.);
#20970=ORIENTED_EDGE('',*,*,#15478,.T.);
#20971=ORIENTED_EDGE('',*,*,#15479,.T.);
#20972=ORIENTED_EDGE('',*,*,#15480,.T.);
#20973=ORIENTED_EDGE('',*,*,#15481,.T.);
#20974=ORIENTED_EDGE('',*,*,#15482,.T.);
#20975=ORIENTED_EDGE('',*,*,#15483,.T.);
#20976=ORIENTED_EDGE('',*,*,#15481,.F.);
#20977=ORIENTED_EDGE('',*,*,#15484,.T.);
#20978=ORIENTED_EDGE('',*,*,#15485,.T.);
#20979=ORIENTED_EDGE('',*,*,#15486,.F.);
#20980=ORIENTED_EDGE('',*,*,#15487,.T.);
#20981=ORIENTED_EDGE('',*,*,#15480,.F.);
#20982=ORIENTED_EDGE('',*,*,#15488,.T.);
#20983=ORIENTED_EDGE('',*,*,#15489,.F.);
#20984=ORIENTED_EDGE('',*,*,#15490,.F.);
#20985=ORIENTED_EDGE('',*,*,#15491,.T.);
#20986=ORIENTED_EDGE('',*,*,#15484,.F.);
#20987=ORIENTED_EDGE('',*,*,#15479,.F.);
#20988=ORIENTED_EDGE('',*,*,#15492,.F.);
#20989=ORIENTED_EDGE('',*,*,#15493,.F.);
#20990=ORIENTED_EDGE('',*,*,#15488,.F.);
#20991=ORIENTED_EDGE('',*,*,#15489,.T.);
#20992=ORIENTED_EDGE('',*,*,#15493,.T.);
#20993=ORIENTED_EDGE('',*,*,#15494,.T.);
#20994=ORIENTED_EDGE('',*,*,#15495,.T.);
#20995=ORIENTED_EDGE('',*,*,#15496,.T.);
#20996=ORIENTED_EDGE('',*,*,#15497,.T.);
#20997=ORIENTED_EDGE('',*,*,#15497,.F.);
#20998=ORIENTED_EDGE('',*,*,#15498,.T.);
#20999=ORIENTED_EDGE('',*,*,#15499,.T.);
#21000=ORIENTED_EDGE('',*,*,#15500,.T.);
#21001=ORIENTED_EDGE('',*,*,#15490,.T.);
#21002=ORIENTED_EDGE('',*,*,#15501,.T.);
#21003=ORIENTED_EDGE('',*,*,#15502,.T.);
#21004=ORIENTED_EDGE('',*,*,#15503,.T.);
#21005=ORIENTED_EDGE('',*,*,#15504,.T.);
#21006=ORIENTED_EDGE('',*,*,#15505,.T.);
#21007=ORIENTED_EDGE('',*,*,#15506,.T.);
#21008=ORIENTED_EDGE('',*,*,#15505,.F.);
#21009=ORIENTED_EDGE('',*,*,#15507,.F.);
#21010=ORIENTED_EDGE('',*,*,#15508,.F.);
#21011=ORIENTED_EDGE('',*,*,#15509,.F.);
#21012=ORIENTED_EDGE('',*,*,#15504,.F.);
#21013=ORIENTED_EDGE('',*,*,#15510,.T.);
#21014=ORIENTED_EDGE('',*,*,#15511,.T.);
#21015=ORIENTED_EDGE('',*,*,#15512,.F.);
#21016=ORIENTED_EDGE('',*,*,#15507,.T.);
#21017=ORIENTED_EDGE('',*,*,#15069,.F.);
#21018=ORIENTED_EDGE('',*,*,#15078,.F.);
#21019=ORIENTED_EDGE('',*,*,#15513,.T.);
#21020=ORIENTED_EDGE('',*,*,#15510,.F.);
#21021=ORIENTED_EDGE('',*,*,#15503,.F.);
#21022=ORIENTED_EDGE('',*,*,#15514,.T.);
#21023=ORIENTED_EDGE('',*,*,#15515,.T.);
#21024=ORIENTED_EDGE('',*,*,#15348,.F.);
#21025=ORIENTED_EDGE('',*,*,#15516,.T.);
#21026=ORIENTED_EDGE('',*,*,#15362,.T.);
#21027=ORIENTED_EDGE('',*,*,#15516,.F.);
#21028=ORIENTED_EDGE('',*,*,#15517,.F.);
#21029=ORIENTED_EDGE('',*,*,#15518,.F.);
#21030=ORIENTED_EDGE('',*,*,#15359,.T.);
#21031=ORIENTED_EDGE('',*,*,#15345,.F.);
#21032=ORIENTED_EDGE('',*,*,#15519,.F.);
#21033=ORIENTED_EDGE('',*,*,#15517,.T.);
#21034=ORIENTED_EDGE('',*,*,#15347,.F.);
#21035=ORIENTED_EDGE('',*,*,#15520,.T.);
#21036=ORIENTED_EDGE('',*,*,#15325,.F.);
#21037=ORIENTED_EDGE('',*,*,#15521,.T.);
#21038=ORIENTED_EDGE('',*,*,#15335,.T.);
#21039=ORIENTED_EDGE('',*,*,#15331,.F.);
#21040=ORIENTED_EDGE('',*,*,#15336,.F.);
#21041=ORIENTED_EDGE('',*,*,#15522,.F.);
#21042=ORIENTED_EDGE('',*,*,#15523,.F.);
#21043=ORIENTED_EDGE('',*,*,#15521,.F.);
#21044=ORIENTED_EDGE('',*,*,#15524,.F.);
#21045=ORIENTED_EDGE('',*,*,#15525,.F.);
#21046=ORIENTED_EDGE('',*,*,#15522,.T.);
#21047=ORIENTED_EDGE('',*,*,#15322,.F.);
#21048=ORIENTED_EDGE('',*,*,#15526,.F.);
#21049=ORIENTED_EDGE('',*,*,#15524,.T.);
#21050=ORIENTED_EDGE('',*,*,#15324,.F.);
#21051=ORIENTED_EDGE('',*,*,#15527,.T.);
#21052=ORIENTED_EDGE('',*,*,#15076,.T.);
#21053=ORIENTED_EDGE('',*,*,#15528,.T.);
#21054=ORIENTED_EDGE('',*,*,#15312,.T.);
#21055=ORIENTED_EDGE('',*,*,#15308,.F.);
#21056=ORIENTED_EDGE('',*,*,#15313,.F.);
#21057=ORIENTED_EDGE('',*,*,#15529,.F.);
#21058=ORIENTED_EDGE('',*,*,#15530,.F.);
#21059=ORIENTED_EDGE('',*,*,#15528,.F.);
#21060=ORIENTED_EDGE('',*,*,#15080,.F.);
#21061=ORIENTED_EDGE('',*,*,#15531,.F.);
#21062=ORIENTED_EDGE('',*,*,#15529,.T.);
#21063=ORIENTED_EDGE('',*,*,#15361,.F.);
#21064=ORIENTED_EDGE('',*,*,#15532,.F.);
#21065=ORIENTED_EDGE('',*,*,#15533,.F.);
#21066=ORIENTED_EDGE('',*,*,#15534,.F.);
#21067=ORIENTED_EDGE('',*,*,#15535,.F.);
#21068=ORIENTED_EDGE('',*,*,#15536,.F.);
#21069=ORIENTED_EDGE('',*,*,#15537,.F.);
#21070=ORIENTED_EDGE('',*,*,#15538,.F.);
#21071=ORIENTED_EDGE('',*,*,#15539,.F.);
#21072=ORIENTED_EDGE('',*,*,#15540,.F.);
#21073=ORIENTED_EDGE('',*,*,#15541,.F.);
#21074=ORIENTED_EDGE('',*,*,#15542,.F.);
#21075=ORIENTED_EDGE('',*,*,#15543,.F.);
#21076=ORIENTED_EDGE('',*,*,#15544,.F.);
#21077=ORIENTED_EDGE('',*,*,#15545,.F.);
#21078=ORIENTED_EDGE('',*,*,#15546,.F.);
#21079=ORIENTED_EDGE('',*,*,#15547,.F.);
#21080=ORIENTED_EDGE('',*,*,#15548,.F.);
#21081=ORIENTED_EDGE('',*,*,#15549,.F.);
#21082=ORIENTED_EDGE('',*,*,#15550,.F.);
#21083=ORIENTED_EDGE('',*,*,#15551,.F.);
#21084=ORIENTED_EDGE('',*,*,#15552,.F.);
#21085=ORIENTED_EDGE('',*,*,#15553,.F.);
#21086=ORIENTED_EDGE('',*,*,#15554,.F.);
#21087=ORIENTED_EDGE('',*,*,#15555,.F.);
#21088=ORIENTED_EDGE('',*,*,#15556,.F.);
#21089=ORIENTED_EDGE('',*,*,#15557,.F.);
#21090=ORIENTED_EDGE('',*,*,#15558,.F.);
#21091=ORIENTED_EDGE('',*,*,#15559,.F.);
#21092=ORIENTED_EDGE('',*,*,#15094,.F.);
#21093=ORIENTED_EDGE('',*,*,#15099,.F.);
#21094=ORIENTED_EDGE('',*,*,#15560,.F.);
#21095=ORIENTED_EDGE('',*,*,#15107,.F.);
#21096=ORIENTED_EDGE('',*,*,#15113,.F.);
#21097=ORIENTED_EDGE('',*,*,#15122,.F.);
#21098=ORIENTED_EDGE('',*,*,#15561,.F.);
#21099=ORIENTED_EDGE('',*,*,#15133,.F.);
#21100=ORIENTED_EDGE('',*,*,#15135,.F.);
#21101=ORIENTED_EDGE('',*,*,#15046,.F.);
#21102=ORIENTED_EDGE('',*,*,#15562,.F.);
#21103=ORIENTED_EDGE('',*,*,#15563,.F.);
#21104=ORIENTED_EDGE('',*,*,#15564,.F.);
#21105=ORIENTED_EDGE('',*,*,#15565,.F.);
#21106=ORIENTED_EDGE('',*,*,#15566,.F.);
#21107=ORIENTED_EDGE('',*,*,#15567,.F.);
#21108=ORIENTED_EDGE('',*,*,#15568,.F.);
#21109=ORIENTED_EDGE('',*,*,#15569,.F.);
#21110=ORIENTED_EDGE('',*,*,#15570,.F.);
#21111=ORIENTED_EDGE('',*,*,#15571,.F.);
#21112=ORIENTED_EDGE('',*,*,#15572,.F.);
#21113=ORIENTED_EDGE('',*,*,#15573,.F.);
#21114=ORIENTED_EDGE('',*,*,#15574,.F.);
#21115=ORIENTED_EDGE('',*,*,#15575,.F.);
#21116=ORIENTED_EDGE('',*,*,#15576,.F.);
#21117=ORIENTED_EDGE('',*,*,#15577,.F.);
#21118=ORIENTED_EDGE('',*,*,#15578,.F.);
#21119=ORIENTED_EDGE('',*,*,#15579,.F.);
#21120=ORIENTED_EDGE('',*,*,#15580,.F.);
#21121=ORIENTED_EDGE('',*,*,#15581,.F.);
#21122=ORIENTED_EDGE('',*,*,#15582,.F.);
#21123=ORIENTED_EDGE('',*,*,#15583,.F.);
#21124=ORIENTED_EDGE('',*,*,#15584,.F.);
#21125=ORIENTED_EDGE('',*,*,#15585,.F.);
#21126=ORIENTED_EDGE('',*,*,#15586,.F.);
#21127=ORIENTED_EDGE('',*,*,#15587,.F.);
#21128=ORIENTED_EDGE('',*,*,#15147,.F.);
#21129=ORIENTED_EDGE('',*,*,#15152,.F.);
#21130=ORIENTED_EDGE('',*,*,#15588,.F.);
#21131=ORIENTED_EDGE('',*,*,#15160,.F.);
#21132=ORIENTED_EDGE('',*,*,#15166,.F.);
#21133=ORIENTED_EDGE('',*,*,#15175,.F.);
#21134=ORIENTED_EDGE('',*,*,#15589,.F.);
#21135=ORIENTED_EDGE('',*,*,#15186,.F.);
#21136=ORIENTED_EDGE('',*,*,#15188,.F.);
#21137=ORIENTED_EDGE('',*,*,#15031,.F.);
#21138=ORIENTED_EDGE('',*,*,#15590,.F.);
#21139=ORIENTED_EDGE('',*,*,#15197,.F.);
#21140=ORIENTED_EDGE('',*,*,#15203,.F.);
#21141=ORIENTED_EDGE('',*,*,#15212,.F.);
#21142=ORIENTED_EDGE('',*,*,#15591,.F.);
#21143=ORIENTED_EDGE('',*,*,#15223,.F.);
#21144=ORIENTED_EDGE('',*,*,#15228,.F.);
#21145=ORIENTED_EDGE('',*,*,#15592,.F.);
#21146=ORIENTED_EDGE('',*,*,#15593,.F.);
#21147=ORIENTED_EDGE('',*,*,#15250,.F.);
#21148=ORIENTED_EDGE('',*,*,#15256,.F.);
#21149=ORIENTED_EDGE('',*,*,#15265,.F.);
#21150=ORIENTED_EDGE('',*,*,#15594,.F.);
#21151=ORIENTED_EDGE('',*,*,#15273,.F.);
#21152=ORIENTED_EDGE('',*,*,#15279,.F.);
#21153=ORIENTED_EDGE('',*,*,#15288,.F.);
#21154=ORIENTED_EDGE('',*,*,#15595,.F.);
#21155=ORIENTED_EDGE('',*,*,#15302,.F.);
#21156=ORIENTED_EDGE('',*,*,#15596,.F.);
#21157=ORIENTED_EDGE('',*,*,#15384,.F.);
#21158=ORIENTED_EDGE('',*,*,#15391,.F.);
#21159=ORIENTED_EDGE('',*,*,#15400,.F.);
#21160=ORIENTED_EDGE('',*,*,#15406,.F.);
#21161=ORIENTED_EDGE('',*,*,#15597,.F.);
#21162=ORIENTED_EDGE('',*,*,#15598,.F.);
#21163=ORIENTED_EDGE('',*,*,#15599,.F.);
#21164=ORIENTED_EDGE('',*,*,#15600,.F.);
#21165=ORIENTED_EDGE('',*,*,#15601,.F.);
#21166=ORIENTED_EDGE('',*,*,#15602,.F.);
#21167=ORIENTED_EDGE('',*,*,#15416,.F.);
#21168=ORIENTED_EDGE('',*,*,#15422,.F.);
#21169=ORIENTED_EDGE('',*,*,#15431,.F.);
#21170=ORIENTED_EDGE('',*,*,#15603,.F.);
#21171=ORIENTED_EDGE('',*,*,#15439,.F.);
#21172=ORIENTED_EDGE('',*,*,#15445,.F.);
#21173=ORIENTED_EDGE('',*,*,#15454,.F.);
#21174=ORIENTED_EDGE('',*,*,#15604,.F.);
#21175=ORIENTED_EDGE('',*,*,#15462,.F.);
#21176=ORIENTED_EDGE('',*,*,#15468,.F.);
#21177=ORIENTED_EDGE('',*,*,#15477,.F.);
#21178=ORIENTED_EDGE('',*,*,#15605,.F.);
#21179=ORIENTED_EDGE('',*,*,#15485,.F.);
#21180=ORIENTED_EDGE('',*,*,#15491,.F.);
#21181=ORIENTED_EDGE('',*,*,#15500,.F.);
#21182=ORIENTED_EDGE('',*,*,#15606,.F.);
#21183=ORIENTED_EDGE('',*,*,#15511,.F.);
#21184=ORIENTED_EDGE('',*,*,#15513,.F.);
#21185=ORIENTED_EDGE('',*,*,#15077,.F.);
#21186=ORIENTED_EDGE('',*,*,#15527,.F.);
#21187=ORIENTED_EDGE('',*,*,#15311,.F.);
#21188=ORIENTED_EDGE('',*,*,#15317,.F.);
#21189=ORIENTED_EDGE('',*,*,#15326,.F.);
#21190=ORIENTED_EDGE('',*,*,#15520,.F.);
#21191=ORIENTED_EDGE('',*,*,#15334,.F.);
#21192=ORIENTED_EDGE('',*,*,#15340,.F.);
#21193=ORIENTED_EDGE('',*,*,#15349,.F.);
#21194=ORIENTED_EDGE('',*,*,#15515,.F.);
#21195=ORIENTED_EDGE('',*,*,#15606,.T.);
#21196=ORIENTED_EDGE('',*,*,#15499,.F.);
#21197=ORIENTED_EDGE('',*,*,#15607,.T.);
#21198=ORIENTED_EDGE('',*,*,#15512,.T.);
#21199=ORIENTED_EDGE('',*,*,#15607,.F.);
#21200=ORIENTED_EDGE('',*,*,#15608,.F.);
#21201=ORIENTED_EDGE('',*,*,#15609,.F.);
#21202=ORIENTED_EDGE('',*,*,#15508,.T.);
#21203=ORIENTED_EDGE('',*,*,#15496,.F.);
#21204=ORIENTED_EDGE('',*,*,#15610,.F.);
#21205=ORIENTED_EDGE('',*,*,#15608,.T.);
#21206=ORIENTED_EDGE('',*,*,#15498,.F.);
#21207=ORIENTED_EDGE('',*,*,#15605,.T.);
#21208=ORIENTED_EDGE('',*,*,#15476,.F.);
#21209=ORIENTED_EDGE('',*,*,#15611,.T.);
#21210=ORIENTED_EDGE('',*,*,#15486,.T.);
#21211=ORIENTED_EDGE('',*,*,#15482,.F.);
#21212=ORIENTED_EDGE('',*,*,#15487,.F.);
#21213=ORIENTED_EDGE('',*,*,#15612,.F.);
#21214=ORIENTED_EDGE('',*,*,#15613,.F.);
#21215=ORIENTED_EDGE('',*,*,#15611,.F.);
#21216=ORIENTED_EDGE('',*,*,#15614,.F.);
#21217=ORIENTED_EDGE('',*,*,#15615,.F.);
#21218=ORIENTED_EDGE('',*,*,#15612,.T.);
#21219=ORIENTED_EDGE('',*,*,#15473,.F.);
#21220=ORIENTED_EDGE('',*,*,#15616,.F.);
#21221=ORIENTED_EDGE('',*,*,#15614,.T.);
#21222=ORIENTED_EDGE('',*,*,#15475,.F.);
#21223=ORIENTED_EDGE('',*,*,#15604,.T.);
#21224=ORIENTED_EDGE('',*,*,#15453,.F.);
#21225=ORIENTED_EDGE('',*,*,#15617,.T.);
#21226=ORIENTED_EDGE('',*,*,#15463,.T.);
#21227=ORIENTED_EDGE('',*,*,#15459,.F.);
#21228=ORIENTED_EDGE('',*,*,#15464,.F.);
#21229=ORIENTED_EDGE('',*,*,#15618,.F.);
#21230=ORIENTED_EDGE('',*,*,#15619,.F.);
#21231=ORIENTED_EDGE('',*,*,#15617,.F.);
#21232=ORIENTED_EDGE('',*,*,#15620,.F.);
#21233=ORIENTED_EDGE('',*,*,#15621,.F.);
#21234=ORIENTED_EDGE('',*,*,#15618,.T.);
#21235=ORIENTED_EDGE('',*,*,#15450,.F.);
#21236=ORIENTED_EDGE('',*,*,#15622,.F.);
#21237=ORIENTED_EDGE('',*,*,#15620,.T.);
#21238=ORIENTED_EDGE('',*,*,#15452,.F.);
#21239=ORIENTED_EDGE('',*,*,#15603,.T.);
#21240=ORIENTED_EDGE('',*,*,#15430,.F.);
#21241=ORIENTED_EDGE('',*,*,#15623,.T.);
#21242=ORIENTED_EDGE('',*,*,#15440,.T.);
#21243=ORIENTED_EDGE('',*,*,#15436,.F.);
#21244=ORIENTED_EDGE('',*,*,#15441,.F.);
#21245=ORIENTED_EDGE('',*,*,#15624,.F.);
#21246=ORIENTED_EDGE('',*,*,#15625,.F.);
#21247=ORIENTED_EDGE('',*,*,#15623,.F.);
#21248=ORIENTED_EDGE('',*,*,#15626,.F.);
#21249=ORIENTED_EDGE('',*,*,#15627,.F.);
#21250=ORIENTED_EDGE('',*,*,#15624,.T.);
#21251=ORIENTED_EDGE('',*,*,#15427,.F.);
#21252=ORIENTED_EDGE('',*,*,#15628,.F.);
#21253=ORIENTED_EDGE('',*,*,#15626,.T.);
#21254=ORIENTED_EDGE('',*,*,#15429,.F.);
#21255=ORIENTED_EDGE('',*,*,#15602,.T.);
#21256=ORIENTED_EDGE('',*,*,#15629,.T.);
#21257=ORIENTED_EDGE('',*,*,#15630,.T.);
#21258=ORIENTED_EDGE('',*,*,#15417,.T.);
#21259=ORIENTED_EDGE('',*,*,#15413,.F.);
#21260=ORIENTED_EDGE('',*,*,#15418,.F.);
#21261=ORIENTED_EDGE('',*,*,#15631,.F.);
#21262=ORIENTED_EDGE('',*,*,#15632,.F.);
#21263=ORIENTED_EDGE('',*,*,#15630,.F.);
#21264=ORIENTED_EDGE('',*,*,#15633,.F.);
#21265=ORIENTED_EDGE('',*,*,#15634,.F.);
#21266=ORIENTED_EDGE('',*,*,#15631,.T.);
#21267=ORIENTED_EDGE('',*,*,#15635,.T.);
#21268=ORIENTED_EDGE('',*,*,#15636,.T.);
#21269=ORIENTED_EDGE('',*,*,#15637,.T.);
#21270=ORIENTED_EDGE('',*,*,#15638,.T.);
#21271=ORIENTED_EDGE('',*,*,#15637,.F.);
#21272=ORIENTED_EDGE('',*,*,#15639,.T.);
#21273=ORIENTED_EDGE('',*,*,#15640,.F.);
#21274=ORIENTED_EDGE('',*,*,#15641,.F.);
#21275=ORIENTED_EDGE('',*,*,#15642,.T.);
#21276=ORIENTED_EDGE('',*,*,#15636,.F.);
#21277=ORIENTED_EDGE('',*,*,#15643,.T.);
#21278=ORIENTED_EDGE('',*,*,#15644,.F.);
#21279=ORIENTED_EDGE('',*,*,#15639,.F.);
#21280=ORIENTED_EDGE('',*,*,#15645,.T.);
#21281=ORIENTED_EDGE('',*,*,#15644,.T.);
#21282=ORIENTED_EDGE('',*,*,#15401,.T.);
#21283=ORIENTED_EDGE('',*,*,#15389,.T.);
#21284=ORIENTED_EDGE('',*,*,#15646,.T.);
#21285=ORIENTED_EDGE('',*,*,#15647,.T.);
#21286=ORIENTED_EDGE('',*,*,#15395,.F.);
#21287=ORIENTED_EDGE('',*,*,#15640,.T.);
#21288=ORIENTED_EDGE('',*,*,#15645,.F.);
#21289=ORIENTED_EDGE('',*,*,#15648,.T.);
#21290=ORIENTED_EDGE('',*,*,#15649,.T.);
#21291=ORIENTED_EDGE('',*,*,#15650,.T.);
#21292=ORIENTED_EDGE('',*,*,#15378,.F.);
#21293=ORIENTED_EDGE('',*,*,#15651,.F.);
#21294=ORIENTED_EDGE('',*,*,#15652,.T.);
#21295=ORIENTED_EDGE('',*,*,#15648,.F.);
#21296=ORIENTED_EDGE('',*,*,#15647,.F.);
#21297=ORIENTED_EDGE('',*,*,#15653,.T.);
#21298=ORIENTED_EDGE('',*,*,#15404,.T.);
#21299=ORIENTED_EDGE('',*,*,#15408,.T.);
#21300=ORIENTED_EDGE('',*,*,#15654,.T.);
#21301=ORIENTED_EDGE('',*,*,#15655,.T.);
#21302=ORIENTED_EDGE('',*,*,#15656,.T.);
#21303=ORIENTED_EDGE('',*,*,#15657,.T.);
#21304=ORIENTED_EDGE('',*,*,#15657,.F.);
#21305=ORIENTED_EDGE('',*,*,#15658,.T.);
#21306=ORIENTED_EDGE('',*,*,#15659,.T.);
#21307=ORIENTED_EDGE('',*,*,#15597,.T.);
#21308=ORIENTED_EDGE('',*,*,#15405,.T.);
#21309=ORIENTED_EDGE('',*,*,#15660,.T.);
#21310=ORIENTED_EDGE('',*,*,#15661,.T.);
#21311=ORIENTED_EDGE('',*,*,#15662,.T.);
#21312=ORIENTED_EDGE('',*,*,#15663,.T.);
#21313=ORIENTED_EDGE('',*,*,#15664,.T.);
#21314=ORIENTED_EDGE('',*,*,#15665,.T.);
#21315=ORIENTED_EDGE('',*,*,#15663,.F.);
#21316=ORIENTED_EDGE('',*,*,#15666,.T.);
#21317=ORIENTED_EDGE('',*,*,#15599,.T.);
#21318=ORIENTED_EDGE('',*,*,#15667,.F.);
#21319=ORIENTED_EDGE('',*,*,#15668,.T.);
#21320=ORIENTED_EDGE('',*,*,#15662,.F.);
#21321=ORIENTED_EDGE('',*,*,#15669,.T.);
#21322=ORIENTED_EDGE('',*,*,#15670,.F.);
#21323=ORIENTED_EDGE('',*,*,#15671,.F.);
#21324=ORIENTED_EDGE('',*,*,#15600,.T.);
#21325=ORIENTED_EDGE('',*,*,#15666,.F.);
#21326=ORIENTED_EDGE('',*,*,#15661,.F.);
#21327=ORIENTED_EDGE('',*,*,#15672,.F.);
#21328=ORIENTED_EDGE('',*,*,#15673,.F.);
#21329=ORIENTED_EDGE('',*,*,#15669,.F.);
#21330=ORIENTED_EDGE('',*,*,#15670,.T.);
#21331=ORIENTED_EDGE('',*,*,#15673,.T.);
#21332=ORIENTED_EDGE('',*,*,#15674,.T.);
#21333=ORIENTED_EDGE('',*,*,#15675,.T.);
#21334=ORIENTED_EDGE('',*,*,#15676,.T.);
#21335=ORIENTED_EDGE('',*,*,#15677,.T.);
#21336=ORIENTED_EDGE('',*,*,#15677,.F.);
#21337=ORIENTED_EDGE('',*,*,#15678,.T.);
#21338=ORIENTED_EDGE('',*,*,#15629,.F.);
#21339=ORIENTED_EDGE('',*,*,#15601,.T.);
#21340=ORIENTED_EDGE('',*,*,#15671,.T.);
#21341=ORIENTED_EDGE('',*,*,#15676,.F.);
#21342=ORIENTED_EDGE('',*,*,#15679,.F.);
#21343=ORIENTED_EDGE('',*,*,#15633,.T.);
#21344=ORIENTED_EDGE('',*,*,#15678,.F.);
#21345=ORIENTED_EDGE('',*,*,#15598,.T.);
#21346=ORIENTED_EDGE('',*,*,#15659,.F.);
#21347=ORIENTED_EDGE('',*,*,#15680,.T.);
#21348=ORIENTED_EDGE('',*,*,#15667,.T.);
#21349=ORIENTED_EDGE('',*,*,#15664,.F.);
#21350=ORIENTED_EDGE('',*,*,#15668,.F.);
#21351=ORIENTED_EDGE('',*,*,#15681,.F.);
#21352=ORIENTED_EDGE('',*,*,#15682,.F.);
#21353=ORIENTED_EDGE('',*,*,#15680,.F.);
#21354=ORIENTED_EDGE('',*,*,#15683,.F.);
#21355=ORIENTED_EDGE('',*,*,#15684,.F.);
#21356=ORIENTED_EDGE('',*,*,#15681,.T.);
#21357=ORIENTED_EDGE('',*,*,#15656,.F.);
#21358=ORIENTED_EDGE('',*,*,#15685,.F.);
#21359=ORIENTED_EDGE('',*,*,#15683,.T.);
#21360=ORIENTED_EDGE('',*,*,#15658,.F.);
#21361=ORIENTED_EDGE('',*,*,#15595,.T.);
#21362=ORIENTED_EDGE('',*,*,#15287,.F.);
#21363=ORIENTED_EDGE('',*,*,#15686,.T.);
#21364=ORIENTED_EDGE('',*,*,#15303,.T.);
#21365=ORIENTED_EDGE('',*,*,#15686,.F.);
#21366=ORIENTED_EDGE('',*,*,#15687,.F.);
#21367=ORIENTED_EDGE('',*,*,#15688,.F.);
#21368=ORIENTED_EDGE('',*,*,#15300,.T.);
#21369=ORIENTED_EDGE('',*,*,#15284,.F.);
#21370=ORIENTED_EDGE('',*,*,#15689,.F.);
#21371=ORIENTED_EDGE('',*,*,#15687,.T.);
#21372=ORIENTED_EDGE('',*,*,#15286,.F.);
#21373=ORIENTED_EDGE('',*,*,#15594,.T.);
#21374=ORIENTED_EDGE('',*,*,#15264,.F.);
#21375=ORIENTED_EDGE('',*,*,#15690,.T.);
#21376=ORIENTED_EDGE('',*,*,#15274,.T.);
#21377=ORIENTED_EDGE('',*,*,#15270,.F.);
#21378=ORIENTED_EDGE('',*,*,#15275,.F.);
#21379=ORIENTED_EDGE('',*,*,#15691,.F.);
#21380=ORIENTED_EDGE('',*,*,#15692,.F.);
#21381=ORIENTED_EDGE('',*,*,#15690,.F.);
#21382=ORIENTED_EDGE('',*,*,#15693,.F.);
#21383=ORIENTED_EDGE('',*,*,#15694,.F.);
#21384=ORIENTED_EDGE('',*,*,#15691,.T.);
#21385=ORIENTED_EDGE('',*,*,#15261,.F.);
#21386=ORIENTED_EDGE('',*,*,#15695,.F.);
#21387=ORIENTED_EDGE('',*,*,#15693,.T.);
#21388=ORIENTED_EDGE('',*,*,#15263,.F.);
#21389=ORIENTED_EDGE('',*,*,#15233,.F.);
#21390=ORIENTED_EDGE('',*,*,#15236,.T.);
#21391=ORIENTED_EDGE('',*,*,#15696,.T.);
#21392=ORIENTED_EDGE('',*,*,#15592,.T.);
#21393=ORIENTED_EDGE('',*,*,#15227,.T.);
#21394=ORIENTED_EDGE('',*,*,#15593,.T.);
#21395=ORIENTED_EDGE('',*,*,#15696,.F.);
#21396=ORIENTED_EDGE('',*,*,#15697,.T.);
#21397=ORIENTED_EDGE('',*,*,#15251,.T.);
#21398=ORIENTED_EDGE('',*,*,#15247,.F.);
#21399=ORIENTED_EDGE('',*,*,#15252,.F.);
#21400=ORIENTED_EDGE('',*,*,#15698,.F.);
#21401=ORIENTED_EDGE('',*,*,#15699,.F.);
#21402=ORIENTED_EDGE('',*,*,#15697,.F.);
#21403=ORIENTED_EDGE('',*,*,#15235,.F.);
#21404=ORIENTED_EDGE('',*,*,#15700,.F.);
#21405=ORIENTED_EDGE('',*,*,#15698,.T.);
#21406=ORIENTED_EDGE('',*,*,#15591,.T.);
#21407=ORIENTED_EDGE('',*,*,#15211,.F.);
#21408=ORIENTED_EDGE('',*,*,#15701,.T.);
#21409=ORIENTED_EDGE('',*,*,#15224,.T.);
#21410=ORIENTED_EDGE('',*,*,#15701,.F.);
#21411=ORIENTED_EDGE('',*,*,#15702,.F.);
#21412=ORIENTED_EDGE('',*,*,#15703,.F.);
#21413=ORIENTED_EDGE('',*,*,#15220,.T.);
#21414=ORIENTED_EDGE('',*,*,#15208,.F.);
#21415=ORIENTED_EDGE('',*,*,#15704,.F.);
#21416=ORIENTED_EDGE('',*,*,#15702,.T.);
#21417=ORIENTED_EDGE('',*,*,#15210,.F.);
#21418=ORIENTED_EDGE('',*,*,#15590,.T.);
#21419=ORIENTED_EDGE('',*,*,#15030,.T.);
#21420=ORIENTED_EDGE('',*,*,#15705,.T.);
#21421=ORIENTED_EDGE('',*,*,#15198,.T.);
#21422=ORIENTED_EDGE('',*,*,#15194,.F.);
#21423=ORIENTED_EDGE('',*,*,#15199,.F.);
#21424=ORIENTED_EDGE('',*,*,#15706,.F.);
#21425=ORIENTED_EDGE('',*,*,#15707,.F.);
#21426=ORIENTED_EDGE('',*,*,#15705,.F.);
#21427=ORIENTED_EDGE('',*,*,#15034,.F.);
#21428=ORIENTED_EDGE('',*,*,#15708,.F.);
#21429=ORIENTED_EDGE('',*,*,#15706,.T.);
#21430=ORIENTED_EDGE('',*,*,#15589,.T.);
#21431=ORIENTED_EDGE('',*,*,#15174,.F.);
#21432=ORIENTED_EDGE('',*,*,#15709,.T.);
#21433=ORIENTED_EDGE('',*,*,#15187,.T.);
#21434=ORIENTED_EDGE('',*,*,#15709,.F.);
#21435=ORIENTED_EDGE('',*,*,#15710,.F.);
#21436=ORIENTED_EDGE('',*,*,#15711,.F.);
#21437=ORIENTED_EDGE('',*,*,#15183,.T.);
#21438=ORIENTED_EDGE('',*,*,#15171,.F.);
#21439=ORIENTED_EDGE('',*,*,#15712,.F.);
#21440=ORIENTED_EDGE('',*,*,#15710,.T.);
#21441=ORIENTED_EDGE('',*,*,#15173,.F.);
#21442=ORIENTED_EDGE('',*,*,#15588,.T.);
#21443=ORIENTED_EDGE('',*,*,#15151,.F.);
#21444=ORIENTED_EDGE('',*,*,#15713,.T.);
#21445=ORIENTED_EDGE('',*,*,#15161,.T.);
#21446=ORIENTED_EDGE('',*,*,#15157,.F.);
#21447=ORIENTED_EDGE('',*,*,#15162,.F.);
#21448=ORIENTED_EDGE('',*,*,#15714,.F.);
#21449=ORIENTED_EDGE('',*,*,#15715,.F.);
#21450=ORIENTED_EDGE('',*,*,#15713,.F.);
#21451=ORIENTED_EDGE('',*,*,#15716,.F.);
#21452=ORIENTED_EDGE('',*,*,#15717,.F.);
#21453=ORIENTED_EDGE('',*,*,#15714,.T.);
#21454=ORIENTED_EDGE('',*,*,#15141,.F.);
#21455=ORIENTED_EDGE('',*,*,#15718,.F.);
#21456=ORIENTED_EDGE('',*,*,#15716,.T.);
#21457=ORIENTED_EDGE('',*,*,#15150,.F.);
#21458=ORIENTED_EDGE('',*,*,#15719,.T.);
#21459=ORIENTED_EDGE('',*,*,#15720,.T.);
#21460=ORIENTED_EDGE('',*,*,#15721,.T.);
#21461=ORIENTED_EDGE('',*,*,#15722,.T.);
#21462=ORIENTED_EDGE('',*,*,#15723,.T.);
#21463=ORIENTED_EDGE('',*,*,#15724,.T.);
#21464=ORIENTED_EDGE('',*,*,#15722,.F.);
#21465=ORIENTED_EDGE('',*,*,#15725,.T.);
#21466=ORIENTED_EDGE('',*,*,#15563,.T.);
#21467=ORIENTED_EDGE('',*,*,#15726,.F.);
#21468=ORIENTED_EDGE('',*,*,#15727,.T.);
#21469=ORIENTED_EDGE('',*,*,#15721,.F.);
#21470=ORIENTED_EDGE('',*,*,#15728,.T.);
#21471=ORIENTED_EDGE('',*,*,#15729,.F.);
#21472=ORIENTED_EDGE('',*,*,#15730,.F.);
#21473=ORIENTED_EDGE('',*,*,#15564,.T.);
#21474=ORIENTED_EDGE('',*,*,#15725,.F.);
#21475=ORIENTED_EDGE('',*,*,#15720,.F.);
#21476=ORIENTED_EDGE('',*,*,#15731,.F.);
#21477=ORIENTED_EDGE('',*,*,#15732,.F.);
#21478=ORIENTED_EDGE('',*,*,#15728,.F.);
#21479=ORIENTED_EDGE('',*,*,#15729,.T.);
#21480=ORIENTED_EDGE('',*,*,#15732,.T.);
#21481=ORIENTED_EDGE('',*,*,#15733,.T.);
#21482=ORIENTED_EDGE('',*,*,#15734,.T.);
#21483=ORIENTED_EDGE('',*,*,#15735,.T.);
#21484=ORIENTED_EDGE('',*,*,#15736,.T.);
#21485=ORIENTED_EDGE('',*,*,#15736,.F.);
#21486=ORIENTED_EDGE('',*,*,#15737,.T.);
#21487=ORIENTED_EDGE('',*,*,#15738,.T.);
#21488=ORIENTED_EDGE('',*,*,#15565,.T.);
#21489=ORIENTED_EDGE('',*,*,#15730,.T.);
#21490=ORIENTED_EDGE('',*,*,#15739,.T.);
#21491=ORIENTED_EDGE('',*,*,#15740,.T.);
#21492=ORIENTED_EDGE('',*,*,#15741,.T.);
#21493=ORIENTED_EDGE('',*,*,#15742,.T.);
#21494=ORIENTED_EDGE('',*,*,#15743,.T.);
#21495=ORIENTED_EDGE('',*,*,#15744,.T.);
#21496=ORIENTED_EDGE('',*,*,#15742,.F.);
#21497=ORIENTED_EDGE('',*,*,#15745,.T.);
#21498=ORIENTED_EDGE('',*,*,#15567,.T.);
#21499=ORIENTED_EDGE('',*,*,#15746,.F.);
#21500=ORIENTED_EDGE('',*,*,#15747,.T.);
#21501=ORIENTED_EDGE('',*,*,#15741,.F.);
#21502=ORIENTED_EDGE('',*,*,#15748,.T.);
#21503=ORIENTED_EDGE('',*,*,#15749,.F.);
#21504=ORIENTED_EDGE('',*,*,#15750,.F.);
#21505=ORIENTED_EDGE('',*,*,#15568,.T.);
#21506=ORIENTED_EDGE('',*,*,#15745,.F.);
#21507=ORIENTED_EDGE('',*,*,#15740,.F.);
#21508=ORIENTED_EDGE('',*,*,#15751,.F.);
#21509=ORIENTED_EDGE('',*,*,#15752,.F.);
#21510=ORIENTED_EDGE('',*,*,#15748,.F.);
#21511=ORIENTED_EDGE('',*,*,#15749,.T.);
#21512=ORIENTED_EDGE('',*,*,#15752,.T.);
#21513=ORIENTED_EDGE('',*,*,#15753,.T.);
#21514=ORIENTED_EDGE('',*,*,#15754,.T.);
#21515=ORIENTED_EDGE('',*,*,#15755,.T.);
#21516=ORIENTED_EDGE('',*,*,#15756,.T.);
#21517=ORIENTED_EDGE('',*,*,#15756,.F.);
#21518=ORIENTED_EDGE('',*,*,#15757,.T.);
#21519=ORIENTED_EDGE('',*,*,#15758,.T.);
#21520=ORIENTED_EDGE('',*,*,#15569,.T.);
#21521=ORIENTED_EDGE('',*,*,#15750,.T.);
#21522=ORIENTED_EDGE('',*,*,#15759,.T.);
#21523=ORIENTED_EDGE('',*,*,#15760,.T.);
#21524=ORIENTED_EDGE('',*,*,#15761,.T.);
#21525=ORIENTED_EDGE('',*,*,#15762,.T.);
#21526=ORIENTED_EDGE('',*,*,#15763,.T.);
#21527=ORIENTED_EDGE('',*,*,#15764,.T.);
#21528=ORIENTED_EDGE('',*,*,#15762,.F.);
#21529=ORIENTED_EDGE('',*,*,#15765,.T.);
#21530=ORIENTED_EDGE('',*,*,#15571,.T.);
#21531=ORIENTED_EDGE('',*,*,#15766,.F.);
#21532=ORIENTED_EDGE('',*,*,#15767,.T.);
#21533=ORIENTED_EDGE('',*,*,#15761,.F.);
#21534=ORIENTED_EDGE('',*,*,#15768,.T.);
#21535=ORIENTED_EDGE('',*,*,#15769,.F.);
#21536=ORIENTED_EDGE('',*,*,#15770,.F.);
#21537=ORIENTED_EDGE('',*,*,#15572,.T.);
#21538=ORIENTED_EDGE('',*,*,#15765,.F.);
#21539=ORIENTED_EDGE('',*,*,#15760,.F.);
#21540=ORIENTED_EDGE('',*,*,#15771,.F.);
#21541=ORIENTED_EDGE('',*,*,#15772,.F.);
#21542=ORIENTED_EDGE('',*,*,#15768,.F.);
#21543=ORIENTED_EDGE('',*,*,#15769,.T.);
#21544=ORIENTED_EDGE('',*,*,#15772,.T.);
#21545=ORIENTED_EDGE('',*,*,#15773,.T.);
#21546=ORIENTED_EDGE('',*,*,#15774,.T.);
#21547=ORIENTED_EDGE('',*,*,#15775,.T.);
#21548=ORIENTED_EDGE('',*,*,#15776,.T.);
#21549=ORIENTED_EDGE('',*,*,#15776,.F.);
#21550=ORIENTED_EDGE('',*,*,#15777,.T.);
#21551=ORIENTED_EDGE('',*,*,#15778,.T.);
#21552=ORIENTED_EDGE('',*,*,#15573,.T.);
#21553=ORIENTED_EDGE('',*,*,#15770,.T.);
#21554=ORIENTED_EDGE('',*,*,#15779,.T.);
#21555=ORIENTED_EDGE('',*,*,#15780,.T.);
#21556=ORIENTED_EDGE('',*,*,#15781,.T.);
#21557=ORIENTED_EDGE('',*,*,#15782,.T.);
#21558=ORIENTED_EDGE('',*,*,#15783,.T.);
#21559=ORIENTED_EDGE('',*,*,#15784,.T.);
#21560=ORIENTED_EDGE('',*,*,#15783,.F.);
#21561=ORIENTED_EDGE('',*,*,#15785,.F.);
#21562=ORIENTED_EDGE('',*,*,#15786,.F.);
#21563=ORIENTED_EDGE('',*,*,#15787,.F.);
#21564=ORIENTED_EDGE('',*,*,#15782,.F.);
#21565=ORIENTED_EDGE('',*,*,#15788,.T.);
#21566=ORIENTED_EDGE('',*,*,#15575,.T.);
#21567=ORIENTED_EDGE('',*,*,#15789,.F.);
#21568=ORIENTED_EDGE('',*,*,#15785,.T.);
#21569=ORIENTED_EDGE('',*,*,#15781,.F.);
#21570=ORIENTED_EDGE('',*,*,#15790,.T.);
#21571=ORIENTED_EDGE('',*,*,#15791,.F.);
#21572=ORIENTED_EDGE('',*,*,#15792,.F.);
#21573=ORIENTED_EDGE('',*,*,#15576,.T.);
#21574=ORIENTED_EDGE('',*,*,#15788,.F.);
#21575=ORIENTED_EDGE('',*,*,#15791,.T.);
#21576=ORIENTED_EDGE('',*,*,#15793,.T.);
#21577=ORIENTED_EDGE('',*,*,#15794,.T.);
#21578=ORIENTED_EDGE('',*,*,#15795,.T.);
#21579=ORIENTED_EDGE('',*,*,#15796,.T.);
#21580=ORIENTED_EDGE('',*,*,#15797,.T.);
#21581=ORIENTED_EDGE('',*,*,#15796,.F.);
#21582=ORIENTED_EDGE('',*,*,#15798,.F.);
#21583=ORIENTED_EDGE('',*,*,#15799,.T.);
#21584=ORIENTED_EDGE('',*,*,#15800,.F.);
#21585=ORIENTED_EDGE('',*,*,#15795,.F.);
#21586=ORIENTED_EDGE('',*,*,#15801,.T.);
#21587=ORIENTED_EDGE('',*,*,#15802,.T.);
#21588=ORIENTED_EDGE('',*,*,#15803,.T.);
#21589=ORIENTED_EDGE('',*,*,#15798,.T.);
#21590=ORIENTED_EDGE('',*,*,#15779,.F.);
#21591=ORIENTED_EDGE('',*,*,#15804,.F.);
#21592=ORIENTED_EDGE('',*,*,#15805,.T.);
#21593=ORIENTED_EDGE('',*,*,#15801,.F.);
#21594=ORIENTED_EDGE('',*,*,#15794,.F.);
#21595=ORIENTED_EDGE('',*,*,#15806,.T.);
#21596=ORIENTED_EDGE('',*,*,#15807,.T.);
#21597=ORIENTED_EDGE('',*,*,#15808,.T.);
#21598=ORIENTED_EDGE('',*,*,#15809,.T.);
#21599=ORIENTED_EDGE('',*,*,#15810,.T.);
#21600=ORIENTED_EDGE('',*,*,#15811,.T.);
#21601=ORIENTED_EDGE('',*,*,#15812,.T.);
#21602=ORIENTED_EDGE('',*,*,#15810,.F.);
#21603=ORIENTED_EDGE('',*,*,#15813,.T.);
#21604=ORIENTED_EDGE('',*,*,#15579,.T.);
#21605=ORIENTED_EDGE('',*,*,#15814,.F.);
#21606=ORIENTED_EDGE('',*,*,#15815,.T.);
#21607=ORIENTED_EDGE('',*,*,#15809,.F.);
#21608=ORIENTED_EDGE('',*,*,#15816,.T.);
#21609=ORIENTED_EDGE('',*,*,#15817,.F.);
#21610=ORIENTED_EDGE('',*,*,#15818,.F.);
#21611=ORIENTED_EDGE('',*,*,#15580,.T.);
#21612=ORIENTED_EDGE('',*,*,#15813,.F.);
#21613=ORIENTED_EDGE('',*,*,#15808,.F.);
#21614=ORIENTED_EDGE('',*,*,#15819,.F.);
#21615=ORIENTED_EDGE('',*,*,#15820,.F.);
#21616=ORIENTED_EDGE('',*,*,#15816,.F.);
#21617=ORIENTED_EDGE('',*,*,#15817,.T.);
#21618=ORIENTED_EDGE('',*,*,#15820,.T.);
#21619=ORIENTED_EDGE('',*,*,#15821,.T.);
#21620=ORIENTED_EDGE('',*,*,#15822,.T.);
#21621=ORIENTED_EDGE('',*,*,#15823,.T.);
#21622=ORIENTED_EDGE('',*,*,#15824,.T.);
#21623=ORIENTED_EDGE('',*,*,#15824,.F.);
#21624=ORIENTED_EDGE('',*,*,#15825,.T.);
#21625=ORIENTED_EDGE('',*,*,#15826,.T.);
#21626=ORIENTED_EDGE('',*,*,#15581,.T.);
#21627=ORIENTED_EDGE('',*,*,#15818,.T.);
#21628=ORIENTED_EDGE('',*,*,#15827,.T.);
#21629=ORIENTED_EDGE('',*,*,#15828,.T.);
#21630=ORIENTED_EDGE('',*,*,#15829,.T.);
#21631=ORIENTED_EDGE('',*,*,#15830,.T.);
#21632=ORIENTED_EDGE('',*,*,#15831,.T.);
#21633=ORIENTED_EDGE('',*,*,#15832,.T.);
#21634=ORIENTED_EDGE('',*,*,#15830,.F.);
#21635=ORIENTED_EDGE('',*,*,#15833,.T.);
#21636=ORIENTED_EDGE('',*,*,#15583,.T.);
#21637=ORIENTED_EDGE('',*,*,#15834,.F.);
#21638=ORIENTED_EDGE('',*,*,#15835,.T.);
#21639=ORIENTED_EDGE('',*,*,#15829,.F.);
#21640=ORIENTED_EDGE('',*,*,#15836,.T.);
#21641=ORIENTED_EDGE('',*,*,#15837,.F.);
#21642=ORIENTED_EDGE('',*,*,#15838,.F.);
#21643=ORIENTED_EDGE('',*,*,#15584,.T.);
#21644=ORIENTED_EDGE('',*,*,#15833,.F.);
#21645=ORIENTED_EDGE('',*,*,#15828,.F.);
#21646=ORIENTED_EDGE('',*,*,#15839,.F.);
#21647=ORIENTED_EDGE('',*,*,#15840,.F.);
#21648=ORIENTED_EDGE('',*,*,#15836,.F.);
#21649=ORIENTED_EDGE('',*,*,#15837,.T.);
#21650=ORIENTED_EDGE('',*,*,#15840,.T.);
#21651=ORIENTED_EDGE('',*,*,#15841,.T.);
#21652=ORIENTED_EDGE('',*,*,#15842,.T.);
#21653=ORIENTED_EDGE('',*,*,#15843,.T.);
#21654=ORIENTED_EDGE('',*,*,#15844,.T.);
#21655=ORIENTED_EDGE('',*,*,#15844,.F.);
#21656=ORIENTED_EDGE('',*,*,#15845,.T.);
#21657=ORIENTED_EDGE('',*,*,#15846,.T.);
#21658=ORIENTED_EDGE('',*,*,#15585,.T.);
#21659=ORIENTED_EDGE('',*,*,#15838,.T.);
#21660=ORIENTED_EDGE('',*,*,#15847,.T.);
#21661=ORIENTED_EDGE('',*,*,#15144,.T.);
#21662=ORIENTED_EDGE('',*,*,#15149,.T.);
#21663=ORIENTED_EDGE('',*,*,#15848,.T.);
#21664=ORIENTED_EDGE('',*,*,#15849,.T.);
#21665=ORIENTED_EDGE('',*,*,#15850,.T.);
#21666=ORIENTED_EDGE('',*,*,#15850,.F.);
#21667=ORIENTED_EDGE('',*,*,#15851,.T.);
#21668=ORIENTED_EDGE('',*,*,#15852,.F.);
#21669=ORIENTED_EDGE('',*,*,#15853,.T.);
#21670=ORIENTED_EDGE('',*,*,#15854,.T.);
#21671=ORIENTED_EDGE('',*,*,#15849,.F.);
#21672=ORIENTED_EDGE('',*,*,#15855,.F.);
#21673=ORIENTED_EDGE('',*,*,#15856,.F.);
#21674=ORIENTED_EDGE('',*,*,#15851,.F.);
#21675=ORIENTED_EDGE('',*,*,#15848,.F.);
#21676=ORIENTED_EDGE('',*,*,#15148,.T.);
#21677=ORIENTED_EDGE('',*,*,#15587,.T.);
#21678=ORIENTED_EDGE('',*,*,#15857,.F.);
#21679=ORIENTED_EDGE('',*,*,#15855,.T.);
#21680=ORIENTED_EDGE('',*,*,#15586,.T.);
#21681=ORIENTED_EDGE('',*,*,#15846,.F.);
#21682=ORIENTED_EDGE('',*,*,#15858,.T.);
#21683=ORIENTED_EDGE('',*,*,#15857,.T.);
#21684=ORIENTED_EDGE('',*,*,#15858,.F.);
#21685=ORIENTED_EDGE('',*,*,#15859,.F.);
#21686=ORIENTED_EDGE('',*,*,#15860,.F.);
#21687=ORIENTED_EDGE('',*,*,#15856,.T.);
#21688=ORIENTED_EDGE('',*,*,#15843,.F.);
#21689=ORIENTED_EDGE('',*,*,#15861,.F.);
#21690=ORIENTED_EDGE('',*,*,#15859,.T.);
#21691=ORIENTED_EDGE('',*,*,#15845,.F.);
#21692=ORIENTED_EDGE('',*,*,#15582,.T.);
#21693=ORIENTED_EDGE('',*,*,#15826,.F.);
#21694=ORIENTED_EDGE('',*,*,#15862,.T.);
#21695=ORIENTED_EDGE('',*,*,#15834,.T.);
#21696=ORIENTED_EDGE('',*,*,#15831,.F.);
#21697=ORIENTED_EDGE('',*,*,#15835,.F.);
#21698=ORIENTED_EDGE('',*,*,#15863,.F.);
#21699=ORIENTED_EDGE('',*,*,#15864,.F.);
#21700=ORIENTED_EDGE('',*,*,#15862,.F.);
#21701=ORIENTED_EDGE('',*,*,#15865,.F.);
#21702=ORIENTED_EDGE('',*,*,#15866,.F.);
#21703=ORIENTED_EDGE('',*,*,#15863,.T.);
#21704=ORIENTED_EDGE('',*,*,#15823,.F.);
#21705=ORIENTED_EDGE('',*,*,#15867,.F.);
#21706=ORIENTED_EDGE('',*,*,#15865,.T.);
#21707=ORIENTED_EDGE('',*,*,#15825,.F.);
#21708=ORIENTED_EDGE('',*,*,#15797,.F.);
#21709=ORIENTED_EDGE('',*,*,#15800,.T.);
#21710=ORIENTED_EDGE('',*,*,#15868,.T.);
#21711=ORIENTED_EDGE('',*,*,#15577,.T.);
#21712=ORIENTED_EDGE('',*,*,#15792,.T.);
#21713=ORIENTED_EDGE('',*,*,#15578,.T.);
#21714=ORIENTED_EDGE('',*,*,#15868,.F.);
#21715=ORIENTED_EDGE('',*,*,#15869,.T.);
#21716=ORIENTED_EDGE('',*,*,#15814,.T.);
#21717=ORIENTED_EDGE('',*,*,#15811,.F.);
#21718=ORIENTED_EDGE('',*,*,#15815,.F.);
#21719=ORIENTED_EDGE('',*,*,#15870,.F.);
#21720=ORIENTED_EDGE('',*,*,#15871,.F.);
#21721=ORIENTED_EDGE('',*,*,#15869,.F.);
#21722=ORIENTED_EDGE('',*,*,#15799,.F.);
#21723=ORIENTED_EDGE('',*,*,#15872,.F.);
#21724=ORIENTED_EDGE('',*,*,#15870,.T.);
#21725=ORIENTED_EDGE('',*,*,#15574,.T.);
#21726=ORIENTED_EDGE('',*,*,#15778,.F.);
#21727=ORIENTED_EDGE('',*,*,#15873,.T.);
#21728=ORIENTED_EDGE('',*,*,#15789,.T.);
#21729=ORIENTED_EDGE('',*,*,#15873,.F.);
#21730=ORIENTED_EDGE('',*,*,#15874,.F.);
#21731=ORIENTED_EDGE('',*,*,#15875,.F.);
#21732=ORIENTED_EDGE('',*,*,#15786,.T.);
#21733=ORIENTED_EDGE('',*,*,#15775,.F.);
#21734=ORIENTED_EDGE('',*,*,#15876,.F.);
#21735=ORIENTED_EDGE('',*,*,#15874,.T.);
#21736=ORIENTED_EDGE('',*,*,#15777,.F.);
#21737=ORIENTED_EDGE('',*,*,#15570,.T.);
#21738=ORIENTED_EDGE('',*,*,#15758,.F.);
#21739=ORIENTED_EDGE('',*,*,#15877,.T.);
#21740=ORIENTED_EDGE('',*,*,#15766,.T.);
#21741=ORIENTED_EDGE('',*,*,#15763,.F.);
#21742=ORIENTED_EDGE('',*,*,#15767,.F.);
#21743=ORIENTED_EDGE('',*,*,#15878,.F.);
#21744=ORIENTED_EDGE('',*,*,#15879,.F.);
#21745=ORIENTED_EDGE('',*,*,#15877,.F.);
#21746=ORIENTED_EDGE('',*,*,#15880,.F.);
#21747=ORIENTED_EDGE('',*,*,#15881,.F.);
#21748=ORIENTED_EDGE('',*,*,#15878,.T.);
#21749=ORIENTED_EDGE('',*,*,#15755,.F.);
#21750=ORIENTED_EDGE('',*,*,#15882,.F.);
#21751=ORIENTED_EDGE('',*,*,#15880,.T.);
#21752=ORIENTED_EDGE('',*,*,#15757,.F.);
#21753=ORIENTED_EDGE('',*,*,#15566,.T.);
#21754=ORIENTED_EDGE('',*,*,#15738,.F.);
#21755=ORIENTED_EDGE('',*,*,#15883,.T.);
#21756=ORIENTED_EDGE('',*,*,#15746,.T.);
#21757=ORIENTED_EDGE('',*,*,#15743,.F.);
#21758=ORIENTED_EDGE('',*,*,#15747,.F.);
#21759=ORIENTED_EDGE('',*,*,#15884,.F.);
#21760=ORIENTED_EDGE('',*,*,#15885,.F.);
#21761=ORIENTED_EDGE('',*,*,#15883,.F.);
#21762=ORIENTED_EDGE('',*,*,#15886,.F.);
#21763=ORIENTED_EDGE('',*,*,#15887,.F.);
#21764=ORIENTED_EDGE('',*,*,#15884,.T.);
#21765=ORIENTED_EDGE('',*,*,#15735,.F.);
#21766=ORIENTED_EDGE('',*,*,#15888,.F.);
#21767=ORIENTED_EDGE('',*,*,#15886,.T.);
#21768=ORIENTED_EDGE('',*,*,#15737,.F.);
#21769=ORIENTED_EDGE('',*,*,#15562,.T.);
#21770=ORIENTED_EDGE('',*,*,#15045,.T.);
#21771=ORIENTED_EDGE('',*,*,#15889,.T.);
#21772=ORIENTED_EDGE('',*,*,#15726,.T.);
#21773=ORIENTED_EDGE('',*,*,#15723,.F.);
#21774=ORIENTED_EDGE('',*,*,#15727,.F.);
#21775=ORIENTED_EDGE('',*,*,#15890,.F.);
#21776=ORIENTED_EDGE('',*,*,#15891,.F.);
#21777=ORIENTED_EDGE('',*,*,#15889,.F.);
#21778=ORIENTED_EDGE('',*,*,#15049,.F.);
#21779=ORIENTED_EDGE('',*,*,#15892,.F.);
#21780=ORIENTED_EDGE('',*,*,#15890,.T.);
#21781=ORIENTED_EDGE('',*,*,#15561,.T.);
#21782=ORIENTED_EDGE('',*,*,#15121,.F.);
#21783=ORIENTED_EDGE('',*,*,#15893,.T.);
#21784=ORIENTED_EDGE('',*,*,#15134,.T.);
#21785=ORIENTED_EDGE('',*,*,#15893,.F.);
#21786=ORIENTED_EDGE('',*,*,#15894,.F.);
#21787=ORIENTED_EDGE('',*,*,#15895,.F.);
#21788=ORIENTED_EDGE('',*,*,#15130,.T.);
#21789=ORIENTED_EDGE('',*,*,#15118,.F.);
#21790=ORIENTED_EDGE('',*,*,#15896,.F.);
#21791=ORIENTED_EDGE('',*,*,#15894,.T.);
#21792=ORIENTED_EDGE('',*,*,#15120,.F.);
#21793=ORIENTED_EDGE('',*,*,#15560,.T.);
#21794=ORIENTED_EDGE('',*,*,#15098,.F.);
#21795=ORIENTED_EDGE('',*,*,#15897,.T.);
#21796=ORIENTED_EDGE('',*,*,#15108,.T.);
#21797=ORIENTED_EDGE('',*,*,#15104,.F.);
#21798=ORIENTED_EDGE('',*,*,#15109,.F.);
#21799=ORIENTED_EDGE('',*,*,#15898,.F.);
#21800=ORIENTED_EDGE('',*,*,#15899,.F.);
#21801=ORIENTED_EDGE('',*,*,#15897,.F.);
#21802=ORIENTED_EDGE('',*,*,#15900,.F.);
#21803=ORIENTED_EDGE('',*,*,#15901,.F.);
#21804=ORIENTED_EDGE('',*,*,#15898,.T.);
#21805=ORIENTED_EDGE('',*,*,#15088,.F.);
#21806=ORIENTED_EDGE('',*,*,#15902,.F.);
#21807=ORIENTED_EDGE('',*,*,#15900,.T.);
#21808=ORIENTED_EDGE('',*,*,#15097,.F.);
#21809=ORIENTED_EDGE('',*,*,#15903,.T.);
#21810=ORIENTED_EDGE('',*,*,#15904,.T.);
#21811=ORIENTED_EDGE('',*,*,#15905,.T.);
#21812=ORIENTED_EDGE('',*,*,#15906,.T.);
#21813=ORIENTED_EDGE('',*,*,#15907,.T.);
#21814=ORIENTED_EDGE('',*,*,#15908,.T.);
#21815=ORIENTED_EDGE('',*,*,#15906,.F.);
#21816=ORIENTED_EDGE('',*,*,#15909,.T.);
#21817=ORIENTED_EDGE('',*,*,#15535,.T.);
#21818=ORIENTED_EDGE('',*,*,#15910,.F.);
#21819=ORIENTED_EDGE('',*,*,#15911,.T.);
#21820=ORIENTED_EDGE('',*,*,#15905,.F.);
#21821=ORIENTED_EDGE('',*,*,#15912,.T.);
#21822=ORIENTED_EDGE('',*,*,#15913,.F.);
#21823=ORIENTED_EDGE('',*,*,#15914,.F.);
#21824=ORIENTED_EDGE('',*,*,#15536,.T.);
#21825=ORIENTED_EDGE('',*,*,#15909,.F.);
#21826=ORIENTED_EDGE('',*,*,#15904,.F.);
#21827=ORIENTED_EDGE('',*,*,#15915,.F.);
#21828=ORIENTED_EDGE('',*,*,#15916,.F.);
#21829=ORIENTED_EDGE('',*,*,#15912,.F.);
#21830=ORIENTED_EDGE('',*,*,#15913,.T.);
#21831=ORIENTED_EDGE('',*,*,#15916,.T.);
#21832=ORIENTED_EDGE('',*,*,#15917,.T.);
#21833=ORIENTED_EDGE('',*,*,#15918,.T.);
#21834=ORIENTED_EDGE('',*,*,#15919,.T.);
#21835=ORIENTED_EDGE('',*,*,#15920,.T.);
#21836=ORIENTED_EDGE('',*,*,#15920,.F.);
#21837=ORIENTED_EDGE('',*,*,#15921,.T.);
#21838=ORIENTED_EDGE('',*,*,#15922,.T.);
#21839=ORIENTED_EDGE('',*,*,#15537,.T.);
#21840=ORIENTED_EDGE('',*,*,#15914,.T.);
#21841=ORIENTED_EDGE('',*,*,#15923,.T.);
#21842=ORIENTED_EDGE('',*,*,#15924,.T.);
#21843=ORIENTED_EDGE('',*,*,#15925,.T.);
#21844=ORIENTED_EDGE('',*,*,#15926,.T.);
#21845=ORIENTED_EDGE('',*,*,#15927,.T.);
#21846=ORIENTED_EDGE('',*,*,#15928,.T.);
#21847=ORIENTED_EDGE('',*,*,#15926,.F.);
#21848=ORIENTED_EDGE('',*,*,#15929,.T.);
#21849=ORIENTED_EDGE('',*,*,#15539,.T.);
#21850=ORIENTED_EDGE('',*,*,#15930,.F.);
#21851=ORIENTED_EDGE('',*,*,#15931,.T.);
#21852=ORIENTED_EDGE('',*,*,#15925,.F.);
#21853=ORIENTED_EDGE('',*,*,#15932,.T.);
#21854=ORIENTED_EDGE('',*,*,#15933,.F.);
#21855=ORIENTED_EDGE('',*,*,#15934,.F.);
#21856=ORIENTED_EDGE('',*,*,#15540,.T.);
#21857=ORIENTED_EDGE('',*,*,#15929,.F.);
#21858=ORIENTED_EDGE('',*,*,#15924,.F.);
#21859=ORIENTED_EDGE('',*,*,#15935,.F.);
#21860=ORIENTED_EDGE('',*,*,#15936,.F.);
#21861=ORIENTED_EDGE('',*,*,#15932,.F.);
#21862=ORIENTED_EDGE('',*,*,#15933,.T.);
#21863=ORIENTED_EDGE('',*,*,#15936,.T.);
#21864=ORIENTED_EDGE('',*,*,#15937,.T.);
#21865=ORIENTED_EDGE('',*,*,#15938,.T.);
#21866=ORIENTED_EDGE('',*,*,#15939,.T.);
#21867=ORIENTED_EDGE('',*,*,#15940,.T.);
#21868=ORIENTED_EDGE('',*,*,#15940,.F.);
#21869=ORIENTED_EDGE('',*,*,#15941,.T.);
#21870=ORIENTED_EDGE('',*,*,#15942,.T.);
#21871=ORIENTED_EDGE('',*,*,#15541,.T.);
#21872=ORIENTED_EDGE('',*,*,#15934,.T.);
#21873=ORIENTED_EDGE('',*,*,#15943,.T.);
#21874=ORIENTED_EDGE('',*,*,#15944,.T.);
#21875=ORIENTED_EDGE('',*,*,#15945,.T.);
#21876=ORIENTED_EDGE('',*,*,#15946,.T.);
#21877=ORIENTED_EDGE('',*,*,#15947,.T.);
#21878=ORIENTED_EDGE('',*,*,#15948,.T.);
#21879=ORIENTED_EDGE('',*,*,#15946,.F.);
#21880=ORIENTED_EDGE('',*,*,#15949,.T.);
#21881=ORIENTED_EDGE('',*,*,#15543,.T.);
#21882=ORIENTED_EDGE('',*,*,#15950,.F.);
#21883=ORIENTED_EDGE('',*,*,#15951,.T.);
#21884=ORIENTED_EDGE('',*,*,#15945,.F.);
#21885=ORIENTED_EDGE('',*,*,#15952,.T.);
#21886=ORIENTED_EDGE('',*,*,#15953,.F.);
#21887=ORIENTED_EDGE('',*,*,#15954,.F.);
#21888=ORIENTED_EDGE('',*,*,#15544,.T.);
#21889=ORIENTED_EDGE('',*,*,#15949,.F.);
#21890=ORIENTED_EDGE('',*,*,#15944,.F.);
#21891=ORIENTED_EDGE('',*,*,#15955,.F.);
#21892=ORIENTED_EDGE('',*,*,#15956,.F.);
#21893=ORIENTED_EDGE('',*,*,#15952,.F.);
#21894=ORIENTED_EDGE('',*,*,#15953,.T.);
#21895=ORIENTED_EDGE('',*,*,#15956,.T.);
#21896=ORIENTED_EDGE('',*,*,#15957,.T.);
#21897=ORIENTED_EDGE('',*,*,#15958,.T.);
#21898=ORIENTED_EDGE('',*,*,#15959,.T.);
#21899=ORIENTED_EDGE('',*,*,#15960,.T.);
#21900=ORIENTED_EDGE('',*,*,#15960,.F.);
#21901=ORIENTED_EDGE('',*,*,#15961,.T.);
#21902=ORIENTED_EDGE('',*,*,#15962,.T.);
#21903=ORIENTED_EDGE('',*,*,#15545,.T.);
#21904=ORIENTED_EDGE('',*,*,#15954,.T.);
#21905=ORIENTED_EDGE('',*,*,#15963,.T.);
#21906=ORIENTED_EDGE('',*,*,#15964,.T.);
#21907=ORIENTED_EDGE('',*,*,#15965,.T.);
#21908=ORIENTED_EDGE('',*,*,#15966,.T.);
#21909=ORIENTED_EDGE('',*,*,#15967,.T.);
#21910=ORIENTED_EDGE('',*,*,#15968,.T.);
#21911=ORIENTED_EDGE('',*,*,#15966,.F.);
#21912=ORIENTED_EDGE('',*,*,#15969,.T.);
#21913=ORIENTED_EDGE('',*,*,#15547,.T.);
#21914=ORIENTED_EDGE('',*,*,#15970,.F.);
#21915=ORIENTED_EDGE('',*,*,#15971,.T.);
#21916=ORIENTED_EDGE('',*,*,#15965,.F.);
#21917=ORIENTED_EDGE('',*,*,#15972,.T.);
#21918=ORIENTED_EDGE('',*,*,#15973,.F.);
#21919=ORIENTED_EDGE('',*,*,#15974,.F.);
#21920=ORIENTED_EDGE('',*,*,#15548,.T.);
#21921=ORIENTED_EDGE('',*,*,#15969,.F.);
#21922=ORIENTED_EDGE('',*,*,#15964,.F.);
#21923=ORIENTED_EDGE('',*,*,#15975,.F.);
#21924=ORIENTED_EDGE('',*,*,#15976,.F.);
#21925=ORIENTED_EDGE('',*,*,#15972,.F.);
#21926=ORIENTED_EDGE('',*,*,#15973,.T.);
#21927=ORIENTED_EDGE('',*,*,#15976,.T.);
#21928=ORIENTED_EDGE('',*,*,#15977,.T.);
#21929=ORIENTED_EDGE('',*,*,#15978,.T.);
#21930=ORIENTED_EDGE('',*,*,#15979,.T.);
#21931=ORIENTED_EDGE('',*,*,#15980,.T.);
#21932=ORIENTED_EDGE('',*,*,#15980,.F.);
#21933=ORIENTED_EDGE('',*,*,#15981,.T.);
#21934=ORIENTED_EDGE('',*,*,#15982,.T.);
#21935=ORIENTED_EDGE('',*,*,#15549,.T.);
#21936=ORIENTED_EDGE('',*,*,#15974,.T.);
#21937=ORIENTED_EDGE('',*,*,#15983,.T.);
#21938=ORIENTED_EDGE('',*,*,#15984,.T.);
#21939=ORIENTED_EDGE('',*,*,#15985,.T.);
#21940=ORIENTED_EDGE('',*,*,#15986,.T.);
#21941=ORIENTED_EDGE('',*,*,#15987,.T.);
#21942=ORIENTED_EDGE('',*,*,#15988,.T.);
#21943=ORIENTED_EDGE('',*,*,#15986,.F.);
#21944=ORIENTED_EDGE('',*,*,#15989,.T.);
#21945=ORIENTED_EDGE('',*,*,#15551,.T.);
#21946=ORIENTED_EDGE('',*,*,#15990,.F.);
#21947=ORIENTED_EDGE('',*,*,#15991,.T.);
#21948=ORIENTED_EDGE('',*,*,#15985,.F.);
#21949=ORIENTED_EDGE('',*,*,#15992,.T.);
#21950=ORIENTED_EDGE('',*,*,#15993,.F.);
#21951=ORIENTED_EDGE('',*,*,#15994,.F.);
#21952=ORIENTED_EDGE('',*,*,#15552,.T.);
#21953=ORIENTED_EDGE('',*,*,#15989,.F.);
#21954=ORIENTED_EDGE('',*,*,#15984,.F.);
#21955=ORIENTED_EDGE('',*,*,#15995,.F.);
#21956=ORIENTED_EDGE('',*,*,#15996,.F.);
#21957=ORIENTED_EDGE('',*,*,#15992,.F.);
#21958=ORIENTED_EDGE('',*,*,#15993,.T.);
#21959=ORIENTED_EDGE('',*,*,#15996,.T.);
#21960=ORIENTED_EDGE('',*,*,#15997,.T.);
#21961=ORIENTED_EDGE('',*,*,#15998,.T.);
#21962=ORIENTED_EDGE('',*,*,#15999,.T.);
#21963=ORIENTED_EDGE('',*,*,#16000,.T.);
#21964=ORIENTED_EDGE('',*,*,#16000,.F.);
#21965=ORIENTED_EDGE('',*,*,#16001,.T.);
#21966=ORIENTED_EDGE('',*,*,#16002,.T.);
#21967=ORIENTED_EDGE('',*,*,#15553,.T.);
#21968=ORIENTED_EDGE('',*,*,#15994,.T.);
#21969=ORIENTED_EDGE('',*,*,#16003,.T.);
#21970=ORIENTED_EDGE('',*,*,#16004,.T.);
#21971=ORIENTED_EDGE('',*,*,#16005,.T.);
#21972=ORIENTED_EDGE('',*,*,#16006,.T.);
#21973=ORIENTED_EDGE('',*,*,#16007,.T.);
#21974=ORIENTED_EDGE('',*,*,#16008,.T.);
#21975=ORIENTED_EDGE('',*,*,#16006,.F.);
#21976=ORIENTED_EDGE('',*,*,#16009,.T.);
#21977=ORIENTED_EDGE('',*,*,#15555,.T.);
#21978=ORIENTED_EDGE('',*,*,#16010,.F.);
#21979=ORIENTED_EDGE('',*,*,#16011,.T.);
#21980=ORIENTED_EDGE('',*,*,#16005,.F.);
#21981=ORIENTED_EDGE('',*,*,#16012,.T.);
#21982=ORIENTED_EDGE('',*,*,#16013,.F.);
#21983=ORIENTED_EDGE('',*,*,#16014,.F.);
#21984=ORIENTED_EDGE('',*,*,#15556,.T.);
#21985=ORIENTED_EDGE('',*,*,#16009,.F.);
#21986=ORIENTED_EDGE('',*,*,#16004,.F.);
#21987=ORIENTED_EDGE('',*,*,#16015,.F.);
#21988=ORIENTED_EDGE('',*,*,#16016,.F.);
#21989=ORIENTED_EDGE('',*,*,#16012,.F.);
#21990=ORIENTED_EDGE('',*,*,#16013,.T.);
#21991=ORIENTED_EDGE('',*,*,#16016,.T.);
#21992=ORIENTED_EDGE('',*,*,#16017,.T.);
#21993=ORIENTED_EDGE('',*,*,#16018,.T.);
#21994=ORIENTED_EDGE('',*,*,#16019,.T.);
#21995=ORIENTED_EDGE('',*,*,#16020,.T.);
#21996=ORIENTED_EDGE('',*,*,#16020,.F.);
#21997=ORIENTED_EDGE('',*,*,#16021,.T.);
#21998=ORIENTED_EDGE('',*,*,#16022,.T.);
#21999=ORIENTED_EDGE('',*,*,#15557,.T.);
#22000=ORIENTED_EDGE('',*,*,#16014,.T.);
#22001=ORIENTED_EDGE('',*,*,#16023,.T.);
#22002=ORIENTED_EDGE('',*,*,#15091,.T.);
#22003=ORIENTED_EDGE('',*,*,#15096,.T.);
#22004=ORIENTED_EDGE('',*,*,#16024,.T.);
#22005=ORIENTED_EDGE('',*,*,#16025,.T.);
#22006=ORIENTED_EDGE('',*,*,#16026,.T.);
#22007=ORIENTED_EDGE('',*,*,#16026,.F.);
#22008=ORIENTED_EDGE('',*,*,#16027,.T.);
#22009=ORIENTED_EDGE('',*,*,#16028,.F.);
#22010=ORIENTED_EDGE('',*,*,#16029,.T.);
#22011=ORIENTED_EDGE('',*,*,#16030,.T.);
#22012=ORIENTED_EDGE('',*,*,#16025,.F.);
#22013=ORIENTED_EDGE('',*,*,#16031,.F.);
#22014=ORIENTED_EDGE('',*,*,#16032,.F.);
#22015=ORIENTED_EDGE('',*,*,#16027,.F.);
#22016=ORIENTED_EDGE('',*,*,#16024,.F.);
#22017=ORIENTED_EDGE('',*,*,#15095,.T.);
#22018=ORIENTED_EDGE('',*,*,#15559,.T.);
#22019=ORIENTED_EDGE('',*,*,#16033,.F.);
#22020=ORIENTED_EDGE('',*,*,#16031,.T.);
#22021=ORIENTED_EDGE('',*,*,#15558,.T.);
#22022=ORIENTED_EDGE('',*,*,#16022,.F.);
#22023=ORIENTED_EDGE('',*,*,#16034,.T.);
#22024=ORIENTED_EDGE('',*,*,#16033,.T.);
#22025=ORIENTED_EDGE('',*,*,#16034,.F.);
#22026=ORIENTED_EDGE('',*,*,#16035,.F.);
#22027=ORIENTED_EDGE('',*,*,#16036,.F.);
#22028=ORIENTED_EDGE('',*,*,#16032,.T.);
#22029=ORIENTED_EDGE('',*,*,#16019,.F.);
#22030=ORIENTED_EDGE('',*,*,#16037,.F.);
#22031=ORIENTED_EDGE('',*,*,#16035,.T.);
#22032=ORIENTED_EDGE('',*,*,#16021,.F.);
#22033=ORIENTED_EDGE('',*,*,#15554,.T.);
#22034=ORIENTED_EDGE('',*,*,#16002,.F.);
#22035=ORIENTED_EDGE('',*,*,#16038,.T.);
#22036=ORIENTED_EDGE('',*,*,#16010,.T.);
#22037=ORIENTED_EDGE('',*,*,#16007,.F.);
#22038=ORIENTED_EDGE('',*,*,#16011,.F.);
#22039=ORIENTED_EDGE('',*,*,#16039,.F.);
#22040=ORIENTED_EDGE('',*,*,#16040,.F.);
#22041=ORIENTED_EDGE('',*,*,#16038,.F.);
#22042=ORIENTED_EDGE('',*,*,#16041,.F.);
#22043=ORIENTED_EDGE('',*,*,#16042,.F.);
#22044=ORIENTED_EDGE('',*,*,#16039,.T.);
#22045=ORIENTED_EDGE('',*,*,#15999,.F.);
#22046=ORIENTED_EDGE('',*,*,#16043,.F.);
#22047=ORIENTED_EDGE('',*,*,#16041,.T.);
#22048=ORIENTED_EDGE('',*,*,#16001,.F.);
#22049=ORIENTED_EDGE('',*,*,#15550,.T.);
#22050=ORIENTED_EDGE('',*,*,#15982,.F.);
#22051=ORIENTED_EDGE('',*,*,#16044,.T.);
#22052=ORIENTED_EDGE('',*,*,#15990,.T.);
#22053=ORIENTED_EDGE('',*,*,#15987,.F.);
#22054=ORIENTED_EDGE('',*,*,#15991,.F.);
#22055=ORIENTED_EDGE('',*,*,#16045,.F.);
#22056=ORIENTED_EDGE('',*,*,#16046,.F.);
#22057=ORIENTED_EDGE('',*,*,#16044,.F.);
#22058=ORIENTED_EDGE('',*,*,#16047,.F.);
#22059=ORIENTED_EDGE('',*,*,#16048,.F.);
#22060=ORIENTED_EDGE('',*,*,#16045,.T.);
#22061=ORIENTED_EDGE('',*,*,#15979,.F.);
#22062=ORIENTED_EDGE('',*,*,#16049,.F.);
#22063=ORIENTED_EDGE('',*,*,#16047,.T.);
#22064=ORIENTED_EDGE('',*,*,#15981,.F.);
#22065=ORIENTED_EDGE('',*,*,#15546,.T.);
#22066=ORIENTED_EDGE('',*,*,#15962,.F.);
#22067=ORIENTED_EDGE('',*,*,#16050,.T.);
#22068=ORIENTED_EDGE('',*,*,#15970,.T.);
#22069=ORIENTED_EDGE('',*,*,#15967,.F.);
#22070=ORIENTED_EDGE('',*,*,#15971,.F.);
#22071=ORIENTED_EDGE('',*,*,#16051,.F.);
#22072=ORIENTED_EDGE('',*,*,#16052,.F.);
#22073=ORIENTED_EDGE('',*,*,#16050,.F.);
#22074=ORIENTED_EDGE('',*,*,#16053,.F.);
#22075=ORIENTED_EDGE('',*,*,#16054,.F.);
#22076=ORIENTED_EDGE('',*,*,#16051,.T.);
#22077=ORIENTED_EDGE('',*,*,#15959,.F.);
#22078=ORIENTED_EDGE('',*,*,#16055,.F.);
#22079=ORIENTED_EDGE('',*,*,#16053,.T.);
#22080=ORIENTED_EDGE('',*,*,#15961,.F.);
#22081=ORIENTED_EDGE('',*,*,#15542,.T.);
#22082=ORIENTED_EDGE('',*,*,#15942,.F.);
#22083=ORIENTED_EDGE('',*,*,#16056,.T.);
#22084=ORIENTED_EDGE('',*,*,#15950,.T.);
#22085=ORIENTED_EDGE('',*,*,#15947,.F.);
#22086=ORIENTED_EDGE('',*,*,#15951,.F.);
#22087=ORIENTED_EDGE('',*,*,#16057,.F.);
#22088=ORIENTED_EDGE('',*,*,#16058,.F.);
#22089=ORIENTED_EDGE('',*,*,#16056,.F.);
#22090=ORIENTED_EDGE('',*,*,#16059,.F.);
#22091=ORIENTED_EDGE('',*,*,#16060,.F.);
#22092=ORIENTED_EDGE('',*,*,#16057,.T.);
#22093=ORIENTED_EDGE('',*,*,#15939,.F.);
#22094=ORIENTED_EDGE('',*,*,#16061,.F.);
#22095=ORIENTED_EDGE('',*,*,#16059,.T.);
#22096=ORIENTED_EDGE('',*,*,#15941,.F.);
#22097=ORIENTED_EDGE('',*,*,#15538,.T.);
#22098=ORIENTED_EDGE('',*,*,#15922,.F.);
#22099=ORIENTED_EDGE('',*,*,#16062,.T.);
#22100=ORIENTED_EDGE('',*,*,#15930,.T.);
#22101=ORIENTED_EDGE('',*,*,#15927,.F.);
#22102=ORIENTED_EDGE('',*,*,#15931,.F.);
#22103=ORIENTED_EDGE('',*,*,#16063,.F.);
#22104=ORIENTED_EDGE('',*,*,#16064,.F.);
#22105=ORIENTED_EDGE('',*,*,#16062,.F.);
#22106=ORIENTED_EDGE('',*,*,#16065,.F.);
#22107=ORIENTED_EDGE('',*,*,#16066,.F.);
#22108=ORIENTED_EDGE('',*,*,#16063,.T.);
#22109=ORIENTED_EDGE('',*,*,#15919,.F.);
#22110=ORIENTED_EDGE('',*,*,#16067,.F.);
#22111=ORIENTED_EDGE('',*,*,#16065,.T.);
#22112=ORIENTED_EDGE('',*,*,#15921,.F.);
#22113=ORIENTED_EDGE('',*,*,#15534,.T.);
#22114=ORIENTED_EDGE('',*,*,#16068,.T.);
#22115=ORIENTED_EDGE('',*,*,#16069,.T.);
#22116=ORIENTED_EDGE('',*,*,#15910,.T.);
#22117=ORIENTED_EDGE('',*,*,#15907,.F.);
#22118=ORIENTED_EDGE('',*,*,#15911,.F.);
#22119=ORIENTED_EDGE('',*,*,#16070,.F.);
#22120=ORIENTED_EDGE('',*,*,#16071,.F.);
#22121=ORIENTED_EDGE('',*,*,#16069,.F.);
#22122=ORIENTED_EDGE('',*,*,#15060,.F.);
#22123=ORIENTED_EDGE('',*,*,#16072,.F.);
#22124=ORIENTED_EDGE('',*,*,#16070,.T.);
#22125=ORIENTED_EDGE('',*,*,#15058,.F.);
#22126=ORIENTED_EDGE('',*,*,#15061,.T.);
#22127=ORIENTED_EDGE('',*,*,#16068,.F.);
#22128=ORIENTED_EDGE('',*,*,#15533,.T.);
#22129=ORIENTED_EDGE('',*,*,#16073,.T.);
#22130=ORIENTED_EDGE('',*,*,#15426,.F.);
#22131=ORIENTED_EDGE('',*,*,#16074,.T.);
#22132=ORIENTED_EDGE('',*,*,#16075,.T.);
#22133=ORIENTED_EDGE('',*,*,#16076,.T.);
#22134=ORIENTED_EDGE('',*,*,#15628,.T.);
#22135=ORIENTED_EDGE('',*,*,#16077,.T.);
#22136=ORIENTED_EDGE('',*,*,#16078,.T.);
#22137=ORIENTED_EDGE('',*,*,#15627,.T.);
#22138=ORIENTED_EDGE('',*,*,#16076,.F.);
#22139=ORIENTED_EDGE('',*,*,#15437,.F.);
#22140=ORIENTED_EDGE('',*,*,#15625,.T.);
#22141=ORIENTED_EDGE('',*,*,#16078,.F.);
#22142=ORIENTED_EDGE('',*,*,#16079,.T.);
#22143=ORIENTED_EDGE('',*,*,#16080,.T.);
#22144=ORIENTED_EDGE('',*,*,#16079,.F.);
#22145=ORIENTED_EDGE('',*,*,#16077,.F.);
#22146=ORIENTED_EDGE('',*,*,#16075,.F.);
#22147=ORIENTED_EDGE('',*,*,#16081,.F.);
#22148=ORIENTED_EDGE('',*,*,#16082,.F.);
#22149=ORIENTED_EDGE('',*,*,#16083,.F.);
#22150=ORIENTED_EDGE('',*,*,#16084,.F.);
#22151=ORIENTED_EDGE('',*,*,#16085,.F.);
#22152=ORIENTED_EDGE('',*,*,#16086,.F.);
#22153=ORIENTED_EDGE('',*,*,#16087,.F.);
#22154=ORIENTED_EDGE('',*,*,#16088,.F.);
#22155=ORIENTED_EDGE('',*,*,#16089,.F.);
#22156=ORIENTED_EDGE('',*,*,#15649,.F.);
#22157=ORIENTED_EDGE('',*,*,#15652,.F.);
#22158=ORIENTED_EDGE('',*,*,#16090,.F.);
#22159=ORIENTED_EDGE('',*,*,#16091,.F.);
#22160=ORIENTED_EDGE('',*,*,#15297,.F.);
#22161=ORIENTED_EDGE('',*,*,#16092,.F.);
#22162=ORIENTED_EDGE('',*,*,#16093,.F.);
#22163=ORIENTED_EDGE('',*,*,#16094,.F.);
#22164=ORIENTED_EDGE('',*,*,#16095,.F.);
#22165=ORIENTED_EDGE('',*,*,#16096,.F.);
#22166=ORIENTED_EDGE('',*,*,#16097,.F.);
#22167=ORIENTED_EDGE('',*,*,#16098,.F.);
#22168=ORIENTED_EDGE('',*,*,#16099,.F.);
#22169=ORIENTED_EDGE('',*,*,#16100,.F.);
#22170=ORIENTED_EDGE('',*,*,#15238,.F.);
#22171=ORIENTED_EDGE('',*,*,#15241,.F.);
#22172=ORIENTED_EDGE('',*,*,#16101,.F.);
#22173=ORIENTED_EDGE('',*,*,#16102,.F.);
#22174=ORIENTED_EDGE('',*,*,#16103,.F.);
#22175=ORIENTED_EDGE('',*,*,#16104,.F.);
#22176=ORIENTED_EDGE('',*,*,#16105,.F.);
#22177=ORIENTED_EDGE('',*,*,#16106,.F.);
#22178=ORIENTED_EDGE('',*,*,#15036,.F.);
#22179=ORIENTED_EDGE('',*,*,#16107,.F.);
#22180=ORIENTED_EDGE('',*,*,#16108,.F.);
#22181=ORIENTED_EDGE('',*,*,#16109,.F.);
#22182=ORIENTED_EDGE('',*,*,#16110,.F.);
#22183=ORIENTED_EDGE('',*,*,#16111,.F.);
#22184=ORIENTED_EDGE('',*,*,#16112,.F.);
#22185=ORIENTED_EDGE('',*,*,#16113,.F.);
#22186=ORIENTED_EDGE('',*,*,#16114,.F.);
#22187=ORIENTED_EDGE('',*,*,#16115,.F.);
#22188=ORIENTED_EDGE('',*,*,#15853,.F.);
#22189=ORIENTED_EDGE('',*,*,#16116,.F.);
#22190=ORIENTED_EDGE('',*,*,#16117,.F.);
#22191=ORIENTED_EDGE('',*,*,#16118,.F.);
#22192=ORIENTED_EDGE('',*,*,#16119,.F.);
#22193=ORIENTED_EDGE('',*,*,#16120,.F.);
#22194=ORIENTED_EDGE('',*,*,#16121,.F.);
#22195=ORIENTED_EDGE('',*,*,#16122,.F.);
#22196=ORIENTED_EDGE('',*,*,#16123,.F.);
#22197=ORIENTED_EDGE('',*,*,#16124,.F.);
#22198=ORIENTED_EDGE('',*,*,#15802,.F.);
#22199=ORIENTED_EDGE('',*,*,#15805,.F.);
#22200=ORIENTED_EDGE('',*,*,#16125,.F.);
#22201=ORIENTED_EDGE('',*,*,#16126,.F.);
#22202=ORIENTED_EDGE('',*,*,#16127,.F.);
#22203=ORIENTED_EDGE('',*,*,#16128,.F.);
#22204=ORIENTED_EDGE('',*,*,#16129,.F.);
#22205=ORIENTED_EDGE('',*,*,#16130,.F.);
#22206=ORIENTED_EDGE('',*,*,#16131,.F.);
#22207=ORIENTED_EDGE('',*,*,#16132,.F.);
#22208=ORIENTED_EDGE('',*,*,#16133,.F.);
#22209=ORIENTED_EDGE('',*,*,#16134,.F.);
#22210=ORIENTED_EDGE('',*,*,#16135,.F.);
#22211=ORIENTED_EDGE('',*,*,#16136,.F.);
#22212=ORIENTED_EDGE('',*,*,#16137,.F.);
#22213=ORIENTED_EDGE('',*,*,#16138,.F.);
#22214=ORIENTED_EDGE('',*,*,#15051,.F.);
#22215=ORIENTED_EDGE('',*,*,#16139,.F.);
#22216=ORIENTED_EDGE('',*,*,#16140,.F.);
#22217=ORIENTED_EDGE('',*,*,#16141,.F.);
#22218=ORIENTED_EDGE('',*,*,#16142,.F.);
#22219=ORIENTED_EDGE('',*,*,#16143,.F.);
#22220=ORIENTED_EDGE('',*,*,#16144,.F.);
#22221=ORIENTED_EDGE('',*,*,#16145,.F.);
#22222=ORIENTED_EDGE('',*,*,#16146,.F.);
#22223=ORIENTED_EDGE('',*,*,#16147,.F.);
#22224=ORIENTED_EDGE('',*,*,#16029,.F.);
#22225=ORIENTED_EDGE('',*,*,#16148,.F.);
#22226=ORIENTED_EDGE('',*,*,#16149,.F.);
#22227=ORIENTED_EDGE('',*,*,#16150,.F.);
#22228=ORIENTED_EDGE('',*,*,#16151,.F.);
#22229=ORIENTED_EDGE('',*,*,#16152,.F.);
#22230=ORIENTED_EDGE('',*,*,#16153,.F.);
#22231=ORIENTED_EDGE('',*,*,#16154,.F.);
#22232=ORIENTED_EDGE('',*,*,#16155,.F.);
#22233=ORIENTED_EDGE('',*,*,#16156,.F.);
#22234=ORIENTED_EDGE('',*,*,#16157,.F.);
#22235=ORIENTED_EDGE('',*,*,#16158,.F.);
#22236=ORIENTED_EDGE('',*,*,#16159,.F.);
#22237=ORIENTED_EDGE('',*,*,#16160,.F.);
#22238=ORIENTED_EDGE('',*,*,#16161,.F.);
#22239=ORIENTED_EDGE('',*,*,#16162,.F.);
#22240=ORIENTED_EDGE('',*,*,#16163,.F.);
#22241=ORIENTED_EDGE('',*,*,#16164,.F.);
#22242=ORIENTED_EDGE('',*,*,#16165,.F.);
#22243=ORIENTED_EDGE('',*,*,#16166,.F.);
#22244=ORIENTED_EDGE('',*,*,#16167,.F.);
#22245=ORIENTED_EDGE('',*,*,#16168,.F.);
#22246=ORIENTED_EDGE('',*,*,#16169,.F.);
#22247=ORIENTED_EDGE('',*,*,#16170,.F.);
#22248=ORIENTED_EDGE('',*,*,#16171,.F.);
#22249=ORIENTED_EDGE('',*,*,#16172,.F.);
#22250=ORIENTED_EDGE('',*,*,#15063,.F.);
#22251=ORIENTED_EDGE('',*,*,#15068,.F.);
#22252=ORIENTED_EDGE('',*,*,#15357,.F.);
#22253=ORIENTED_EDGE('',*,*,#16173,.F.);
#22254=ORIENTED_EDGE('',*,*,#16174,.F.);
#22255=ORIENTED_EDGE('',*,*,#16175,.F.);
#22256=ORIENTED_EDGE('',*,*,#16176,.F.);
#22257=ORIENTED_EDGE('',*,*,#16177,.F.);
#22258=ORIENTED_EDGE('',*,*,#16178,.F.);
#22259=ORIENTED_EDGE('',*,*,#16179,.F.);
#22260=ORIENTED_EDGE('',*,*,#16180,.F.);
#22261=ORIENTED_EDGE('',*,*,#16181,.F.);
#22262=ORIENTED_EDGE('',*,*,#15082,.F.);
#22263=ORIENTED_EDGE('',*,*,#16182,.F.);
#22264=ORIENTED_EDGE('',*,*,#16183,.F.);
#22265=ORIENTED_EDGE('',*,*,#16184,.F.);
#22266=ORIENTED_EDGE('',*,*,#16185,.F.);
#22267=ORIENTED_EDGE('',*,*,#16186,.F.);
#22268=ORIENTED_EDGE('',*,*,#16187,.F.);
#22269=ORIENTED_EDGE('',*,*,#16188,.F.);
#22270=ORIENTED_EDGE('',*,*,#16189,.F.);
#22271=ORIENTED_EDGE('',*,*,#16190,.F.);
#22272=ORIENTED_EDGE('',*,*,#16191,.F.);
#22273=ORIENTED_EDGE('',*,*,#16192,.F.);
#22274=ORIENTED_EDGE('',*,*,#16193,.F.);
#22275=ORIENTED_EDGE('',*,*,#16194,.F.);
#22276=ORIENTED_EDGE('',*,*,#16195,.F.);
#22277=ORIENTED_EDGE('',*,*,#15409,.F.);
#22278=ORIENTED_EDGE('',*,*,#16196,.F.);
#22279=ORIENTED_EDGE('',*,*,#16081,.T.);
#22280=ORIENTED_EDGE('',*,*,#16074,.F.);
#22281=ORIENTED_EDGE('',*,*,#15425,.F.);
#22282=ORIENTED_EDGE('',*,*,#15423,.T.);
#22283=ORIENTED_EDGE('',*,*,#15449,.F.);
#22284=ORIENTED_EDGE('',*,*,#16197,.T.);
#22285=ORIENTED_EDGE('',*,*,#16193,.T.);
#22286=ORIENTED_EDGE('',*,*,#16198,.T.);
#22287=ORIENTED_EDGE('',*,*,#15622,.T.);
#22288=ORIENTED_EDGE('',*,*,#16192,.T.);
#22289=ORIENTED_EDGE('',*,*,#16199,.T.);
#22290=ORIENTED_EDGE('',*,*,#15621,.T.);
#22291=ORIENTED_EDGE('',*,*,#16198,.F.);
#22292=ORIENTED_EDGE('',*,*,#15460,.F.);
#22293=ORIENTED_EDGE('',*,*,#15619,.T.);
#22294=ORIENTED_EDGE('',*,*,#16199,.F.);
#22295=ORIENTED_EDGE('',*,*,#16191,.T.);
#22296=ORIENTED_EDGE('',*,*,#16200,.T.);
#22297=ORIENTED_EDGE('',*,*,#15432,.F.);
#22298=ORIENTED_EDGE('',*,*,#16080,.F.);
#22299=ORIENTED_EDGE('',*,*,#16194,.T.);
#22300=ORIENTED_EDGE('',*,*,#16197,.F.);
#22301=ORIENTED_EDGE('',*,*,#15448,.F.);
#22302=ORIENTED_EDGE('',*,*,#15446,.T.);
#22303=ORIENTED_EDGE('',*,*,#15472,.F.);
#22304=ORIENTED_EDGE('',*,*,#16201,.T.);
#22305=ORIENTED_EDGE('',*,*,#16189,.T.);
#22306=ORIENTED_EDGE('',*,*,#16202,.T.);
#22307=ORIENTED_EDGE('',*,*,#15616,.T.);
#22308=ORIENTED_EDGE('',*,*,#16188,.T.);
#22309=ORIENTED_EDGE('',*,*,#16203,.T.);
#22310=ORIENTED_EDGE('',*,*,#15615,.T.);
#22311=ORIENTED_EDGE('',*,*,#16202,.F.);
#22312=ORIENTED_EDGE('',*,*,#15483,.F.);
#22313=ORIENTED_EDGE('',*,*,#15613,.T.);
#22314=ORIENTED_EDGE('',*,*,#16203,.F.);
#22315=ORIENTED_EDGE('',*,*,#16187,.T.);
#22316=ORIENTED_EDGE('',*,*,#16204,.T.);
#22317=ORIENTED_EDGE('',*,*,#15455,.F.);
#22318=ORIENTED_EDGE('',*,*,#16200,.F.);
#22319=ORIENTED_EDGE('',*,*,#16190,.T.);
#22320=ORIENTED_EDGE('',*,*,#16201,.F.);
#22321=ORIENTED_EDGE('',*,*,#15471,.F.);
#22322=ORIENTED_EDGE('',*,*,#15469,.T.);
#22323=ORIENTED_EDGE('',*,*,#15495,.F.);
#22324=ORIENTED_EDGE('',*,*,#16205,.T.);
#22325=ORIENTED_EDGE('',*,*,#16185,.T.);
#22326=ORIENTED_EDGE('',*,*,#16206,.T.);
#22327=ORIENTED_EDGE('',*,*,#15610,.T.);
#22328=ORIENTED_EDGE('',*,*,#16184,.T.);
#22329=ORIENTED_EDGE('',*,*,#16207,.T.);
#22330=ORIENTED_EDGE('',*,*,#15609,.T.);
#22331=ORIENTED_EDGE('',*,*,#16206,.F.);
#22332=ORIENTED_EDGE('',*,*,#15506,.F.);
#22333=ORIENTED_EDGE('',*,*,#15509,.T.);
#22334=ORIENTED_EDGE('',*,*,#16207,.F.);
#22335=ORIENTED_EDGE('',*,*,#16183,.T.);
#22336=ORIENTED_EDGE('',*,*,#16208,.T.);
#22337=ORIENTED_EDGE('',*,*,#15478,.F.);
#22338=ORIENTED_EDGE('',*,*,#16204,.F.);
#22339=ORIENTED_EDGE('',*,*,#16186,.T.);
#22340=ORIENTED_EDGE('',*,*,#16205,.F.);
#22341=ORIENTED_EDGE('',*,*,#15494,.F.);
#22342=ORIENTED_EDGE('',*,*,#15492,.T.);
#22343=ORIENTED_EDGE('',*,*,#16181,.T.);
#22344=ORIENTED_EDGE('',*,*,#16209,.T.);
#22345=ORIENTED_EDGE('',*,*,#15531,.T.);
#22346=ORIENTED_EDGE('',*,*,#15083,.F.);
#22347=ORIENTED_EDGE('',*,*,#15309,.F.);
#22348=ORIENTED_EDGE('',*,*,#15530,.T.);
#22349=ORIENTED_EDGE('',*,*,#16209,.F.);
#22350=ORIENTED_EDGE('',*,*,#16180,.T.);
#22351=ORIENTED_EDGE('',*,*,#16210,.T.);
#22352=ORIENTED_EDGE('',*,*,#15071,.F.);
#22353=ORIENTED_EDGE('',*,*,#16211,.T.);
#22354=ORIENTED_EDGE('',*,*,#15501,.F.);
#22355=ORIENTED_EDGE('',*,*,#16208,.F.);
#22356=ORIENTED_EDGE('',*,*,#16182,.T.);
#22357=ORIENTED_EDGE('',*,*,#15081,.F.);
#22358=ORIENTED_EDGE('',*,*,#15321,.F.);
#22359=ORIENTED_EDGE('',*,*,#16212,.T.);
#22360=ORIENTED_EDGE('',*,*,#16178,.T.);
#22361=ORIENTED_EDGE('',*,*,#16213,.T.);
#22362=ORIENTED_EDGE('',*,*,#15526,.T.);
#22363=ORIENTED_EDGE('',*,*,#16177,.T.);
#22364=ORIENTED_EDGE('',*,*,#16214,.T.);
#22365=ORIENTED_EDGE('',*,*,#15525,.T.);
#22366=ORIENTED_EDGE('',*,*,#16213,.F.);
#22367=ORIENTED_EDGE('',*,*,#15332,.F.);
#22368=ORIENTED_EDGE('',*,*,#15523,.T.);
#22369=ORIENTED_EDGE('',*,*,#16214,.F.);
#22370=ORIENTED_EDGE('',*,*,#16176,.T.);
#22371=ORIENTED_EDGE('',*,*,#16215,.T.);
#22372=ORIENTED_EDGE('',*,*,#15304,.F.);
#22373=ORIENTED_EDGE('',*,*,#16210,.F.);
#22374=ORIENTED_EDGE('',*,*,#16179,.T.);
#22375=ORIENTED_EDGE('',*,*,#16212,.F.);
#22376=ORIENTED_EDGE('',*,*,#15320,.F.);
#22377=ORIENTED_EDGE('',*,*,#15318,.T.);
#22378=ORIENTED_EDGE('',*,*,#15344,.F.);
#22379=ORIENTED_EDGE('',*,*,#16216,.T.);
#22380=ORIENTED_EDGE('',*,*,#16174,.T.);
#22381=ORIENTED_EDGE('',*,*,#16217,.T.);
#22382=ORIENTED_EDGE('',*,*,#15519,.T.);
#22383=ORIENTED_EDGE('',*,*,#15518,.T.);
#22384=ORIENTED_EDGE('',*,*,#16217,.F.);
#22385=ORIENTED_EDGE('',*,*,#16173,.T.);
#22386=ORIENTED_EDGE('',*,*,#15356,.T.);
#22387=ORIENTED_EDGE('',*,*,#16172,.T.);
#22388=ORIENTED_EDGE('',*,*,#16218,.T.);
#22389=ORIENTED_EDGE('',*,*,#16072,.T.);
#22390=ORIENTED_EDGE('',*,*,#15064,.F.);
#22391=ORIENTED_EDGE('',*,*,#15908,.F.);
#22392=ORIENTED_EDGE('',*,*,#16071,.T.);
#22393=ORIENTED_EDGE('',*,*,#16218,.F.);
#22394=ORIENTED_EDGE('',*,*,#16171,.T.);
#22395=ORIENTED_EDGE('',*,*,#16219,.T.);
#22396=ORIENTED_EDGE('',*,*,#15918,.F.);
#22397=ORIENTED_EDGE('',*,*,#16220,.T.);
#22398=ORIENTED_EDGE('',*,*,#16169,.T.);
#22399=ORIENTED_EDGE('',*,*,#16221,.T.);
#22400=ORIENTED_EDGE('',*,*,#16067,.T.);
#22401=ORIENTED_EDGE('',*,*,#16168,.T.);
#22402=ORIENTED_EDGE('',*,*,#16222,.T.);
#22403=ORIENTED_EDGE('',*,*,#16066,.T.);
#22404=ORIENTED_EDGE('',*,*,#16221,.F.);
#22405=ORIENTED_EDGE('',*,*,#15928,.F.);
#22406=ORIENTED_EDGE('',*,*,#16064,.T.);
#22407=ORIENTED_EDGE('',*,*,#16222,.F.);
#22408=ORIENTED_EDGE('',*,*,#16167,.T.);
#22409=ORIENTED_EDGE('',*,*,#16223,.T.);
#22410=ORIENTED_EDGE('',*,*,#15903,.F.);
#22411=ORIENTED_EDGE('',*,*,#16219,.F.);
#22412=ORIENTED_EDGE('',*,*,#16170,.T.);
#22413=ORIENTED_EDGE('',*,*,#16220,.F.);
#22414=ORIENTED_EDGE('',*,*,#15917,.F.);
#22415=ORIENTED_EDGE('',*,*,#15915,.T.);
#22416=ORIENTED_EDGE('',*,*,#15938,.F.);
#22417=ORIENTED_EDGE('',*,*,#16224,.T.);
#22418=ORIENTED_EDGE('',*,*,#16165,.T.);
#22419=ORIENTED_EDGE('',*,*,#16225,.T.);
#22420=ORIENTED_EDGE('',*,*,#16061,.T.);
#22421=ORIENTED_EDGE('',*,*,#16164,.T.);
#22422=ORIENTED_EDGE('',*,*,#16226,.T.);
#22423=ORIENTED_EDGE('',*,*,#16060,.T.);
#22424=ORIENTED_EDGE('',*,*,#16225,.F.);
#22425=ORIENTED_EDGE('',*,*,#15948,.F.);
#22426=ORIENTED_EDGE('',*,*,#16058,.T.);
#22427=ORIENTED_EDGE('',*,*,#16226,.F.);
#22428=ORIENTED_EDGE('',*,*,#16163,.T.);
#22429=ORIENTED_EDGE('',*,*,#16227,.T.);
#22430=ORIENTED_EDGE('',*,*,#15923,.F.);
#22431=ORIENTED_EDGE('',*,*,#16223,.F.);
#22432=ORIENTED_EDGE('',*,*,#16166,.T.);
#22433=ORIENTED_EDGE('',*,*,#16224,.F.);
#22434=ORIENTED_EDGE('',*,*,#15937,.F.);
#22435=ORIENTED_EDGE('',*,*,#15935,.T.);
#22436=ORIENTED_EDGE('',*,*,#15958,.F.);
#22437=ORIENTED_EDGE('',*,*,#16228,.T.);
#22438=ORIENTED_EDGE('',*,*,#16161,.T.);
#22439=ORIENTED_EDGE('',*,*,#16229,.T.);
#22440=ORIENTED_EDGE('',*,*,#16055,.T.);
#22441=ORIENTED_EDGE('',*,*,#16160,.T.);
#22442=ORIENTED_EDGE('',*,*,#16230,.T.);
#22443=ORIENTED_EDGE('',*,*,#16054,.T.);
#22444=ORIENTED_EDGE('',*,*,#16229,.F.);
#22445=ORIENTED_EDGE('',*,*,#15968,.F.);
#22446=ORIENTED_EDGE('',*,*,#16052,.T.);
#22447=ORIENTED_EDGE('',*,*,#16230,.F.);
#22448=ORIENTED_EDGE('',*,*,#16159,.T.);
#22449=ORIENTED_EDGE('',*,*,#16231,.T.);
#22450=ORIENTED_EDGE('',*,*,#15943,.F.);
#22451=ORIENTED_EDGE('',*,*,#16227,.F.);
#22452=ORIENTED_EDGE('',*,*,#16162,.T.);
#22453=ORIENTED_EDGE('',*,*,#16228,.F.);
#22454=ORIENTED_EDGE('',*,*,#15957,.F.);
#22455=ORIENTED_EDGE('',*,*,#15955,.T.);
#22456=ORIENTED_EDGE('',*,*,#15978,.F.);
#22457=ORIENTED_EDGE('',*,*,#16232,.T.);
#22458=ORIENTED_EDGE('',*,*,#16157,.T.);
#22459=ORIENTED_EDGE('',*,*,#16233,.T.);
#22460=ORIENTED_EDGE('',*,*,#16049,.T.);
#22461=ORIENTED_EDGE('',*,*,#16156,.T.);
#22462=ORIENTED_EDGE('',*,*,#16234,.T.);
#22463=ORIENTED_EDGE('',*,*,#16048,.T.);
#22464=ORIENTED_EDGE('',*,*,#16233,.F.);
#22465=ORIENTED_EDGE('',*,*,#15988,.F.);
#22466=ORIENTED_EDGE('',*,*,#16046,.T.);
#22467=ORIENTED_EDGE('',*,*,#16234,.F.);
#22468=ORIENTED_EDGE('',*,*,#16155,.T.);
#22469=ORIENTED_EDGE('',*,*,#16235,.T.);
#22470=ORIENTED_EDGE('',*,*,#15963,.F.);
#22471=ORIENTED_EDGE('',*,*,#16231,.F.);
#22472=ORIENTED_EDGE('',*,*,#16158,.T.);
#22473=ORIENTED_EDGE('',*,*,#16232,.F.);
#22474=ORIENTED_EDGE('',*,*,#15977,.F.);
#22475=ORIENTED_EDGE('',*,*,#15975,.T.);
#22476=ORIENTED_EDGE('',*,*,#15998,.F.);
#22477=ORIENTED_EDGE('',*,*,#16236,.T.);
#22478=ORIENTED_EDGE('',*,*,#16153,.T.);
#22479=ORIENTED_EDGE('',*,*,#16237,.T.);
#22480=ORIENTED_EDGE('',*,*,#16043,.T.);
#22481=ORIENTED_EDGE('',*,*,#16152,.T.);
#22482=ORIENTED_EDGE('',*,*,#16238,.T.);
#22483=ORIENTED_EDGE('',*,*,#16042,.T.);
#22484=ORIENTED_EDGE('',*,*,#16237,.F.);
#22485=ORIENTED_EDGE('',*,*,#16008,.F.);
#22486=ORIENTED_EDGE('',*,*,#16040,.T.);
#22487=ORIENTED_EDGE('',*,*,#16238,.F.);
#22488=ORIENTED_EDGE('',*,*,#16151,.T.);
#22489=ORIENTED_EDGE('',*,*,#16239,.T.);
#22490=ORIENTED_EDGE('',*,*,#15983,.F.);
#22491=ORIENTED_EDGE('',*,*,#16235,.F.);
#22492=ORIENTED_EDGE('',*,*,#16154,.T.);
#22493=ORIENTED_EDGE('',*,*,#16236,.F.);
#22494=ORIENTED_EDGE('',*,*,#15997,.F.);
#22495=ORIENTED_EDGE('',*,*,#15995,.T.);
#22496=ORIENTED_EDGE('',*,*,#16018,.F.);
#22497=ORIENTED_EDGE('',*,*,#16240,.T.);
#22498=ORIENTED_EDGE('',*,*,#16149,.T.);
#22499=ORIENTED_EDGE('',*,*,#16241,.T.);
#22500=ORIENTED_EDGE('',*,*,#16037,.T.);
#22501=ORIENTED_EDGE('',*,*,#16148,.T.);
#22502=ORIENTED_EDGE('',*,*,#16028,.T.);
#22503=ORIENTED_EDGE('',*,*,#16036,.T.);
#22504=ORIENTED_EDGE('',*,*,#16241,.F.);
#22505=ORIENTED_EDGE('',*,*,#16003,.F.);
#22506=ORIENTED_EDGE('',*,*,#16239,.F.);
#22507=ORIENTED_EDGE('',*,*,#16150,.T.);
#22508=ORIENTED_EDGE('',*,*,#16240,.F.);
#22509=ORIENTED_EDGE('',*,*,#16017,.F.);
#22510=ORIENTED_EDGE('',*,*,#16015,.T.);
#22511=ORIENTED_EDGE('',*,*,#15087,.F.);
#22512=ORIENTED_EDGE('',*,*,#16242,.T.);
#22513=ORIENTED_EDGE('',*,*,#16146,.T.);
#22514=ORIENTED_EDGE('',*,*,#16243,.T.);
#22515=ORIENTED_EDGE('',*,*,#15902,.T.);
#22516=ORIENTED_EDGE('',*,*,#16145,.T.);
#22517=ORIENTED_EDGE('',*,*,#16244,.T.);
#22518=ORIENTED_EDGE('',*,*,#15901,.T.);
#22519=ORIENTED_EDGE('',*,*,#16243,.F.);
#22520=ORIENTED_EDGE('',*,*,#15105,.F.);
#22521=ORIENTED_EDGE('',*,*,#15899,.T.);
#22522=ORIENTED_EDGE('',*,*,#16244,.F.);
#22523=ORIENTED_EDGE('',*,*,#16144,.T.);
#22524=ORIENTED_EDGE('',*,*,#16245,.T.);
#22525=ORIENTED_EDGE('',*,*,#15086,.F.);
#22526=ORIENTED_EDGE('',*,*,#15092,.T.);
#22527=ORIENTED_EDGE('',*,*,#16023,.F.);
#22528=ORIENTED_EDGE('',*,*,#16030,.F.);
#22529=ORIENTED_EDGE('',*,*,#16147,.T.);
#22530=ORIENTED_EDGE('',*,*,#16242,.F.);
#22531=ORIENTED_EDGE('',*,*,#15117,.F.);
#22532=ORIENTED_EDGE('',*,*,#16246,.T.);
#22533=ORIENTED_EDGE('',*,*,#16142,.T.);
#22534=ORIENTED_EDGE('',*,*,#16247,.T.);
#22535=ORIENTED_EDGE('',*,*,#15896,.T.);
#22536=ORIENTED_EDGE('',*,*,#16141,.T.);
#22537=ORIENTED_EDGE('',*,*,#16248,.T.);
#22538=ORIENTED_EDGE('',*,*,#15895,.T.);
#22539=ORIENTED_EDGE('',*,*,#16247,.F.);
#22540=ORIENTED_EDGE('',*,*,#15128,.F.);
#22541=ORIENTED_EDGE('',*,*,#15131,.T.);
#22542=ORIENTED_EDGE('',*,*,#16248,.F.);
#22543=ORIENTED_EDGE('',*,*,#16140,.T.);
#22544=ORIENTED_EDGE('',*,*,#16249,.T.);
#22545=ORIENTED_EDGE('',*,*,#15100,.F.);
#22546=ORIENTED_EDGE('',*,*,#16245,.F.);
#22547=ORIENTED_EDGE('',*,*,#16143,.T.);
#22548=ORIENTED_EDGE('',*,*,#16246,.F.);
#22549=ORIENTED_EDGE('',*,*,#15116,.F.);
#22550=ORIENTED_EDGE('',*,*,#15114,.T.);
#22551=ORIENTED_EDGE('',*,*,#16138,.T.);
#22552=ORIENTED_EDGE('',*,*,#16250,.T.);
#22553=ORIENTED_EDGE('',*,*,#15892,.T.);
#22554=ORIENTED_EDGE('',*,*,#15052,.F.);
#22555=ORIENTED_EDGE('',*,*,#15724,.F.);
#22556=ORIENTED_EDGE('',*,*,#15891,.T.);
#22557=ORIENTED_EDGE('',*,*,#16250,.F.);
#22558=ORIENTED_EDGE('',*,*,#16137,.T.);
#22559=ORIENTED_EDGE('',*,*,#16251,.T.);
#22560=ORIENTED_EDGE('',*,*,#15040,.F.);
#22561=ORIENTED_EDGE('',*,*,#16252,.T.);
#22562=ORIENTED_EDGE('',*,*,#15123,.F.);
#22563=ORIENTED_EDGE('',*,*,#16249,.F.);
#22564=ORIENTED_EDGE('',*,*,#16139,.T.);
#22565=ORIENTED_EDGE('',*,*,#15050,.F.);
#22566=ORIENTED_EDGE('',*,*,#15734,.F.);
#22567=ORIENTED_EDGE('',*,*,#16253,.T.);
#22568=ORIENTED_EDGE('',*,*,#16135,.T.);
#22569=ORIENTED_EDGE('',*,*,#16254,.T.);
#22570=ORIENTED_EDGE('',*,*,#15888,.T.);
#22571=ORIENTED_EDGE('',*,*,#16134,.T.);
#22572=ORIENTED_EDGE('',*,*,#16255,.T.);
#22573=ORIENTED_EDGE('',*,*,#15887,.T.);
#22574=ORIENTED_EDGE('',*,*,#16254,.F.);
#22575=ORIENTED_EDGE('',*,*,#15744,.F.);
#22576=ORIENTED_EDGE('',*,*,#15885,.T.);
#22577=ORIENTED_EDGE('',*,*,#16255,.F.);
#22578=ORIENTED_EDGE('',*,*,#16133,.T.);
#22579=ORIENTED_EDGE('',*,*,#16256,.T.);
#22580=ORIENTED_EDGE('',*,*,#15719,.F.);
#22581=ORIENTED_EDGE('',*,*,#16251,.F.);
#22582=ORIENTED_EDGE('',*,*,#16136,.T.);
#22583=ORIENTED_EDGE('',*,*,#16253,.F.);
#22584=ORIENTED_EDGE('',*,*,#15733,.F.);
#22585=ORIENTED_EDGE('',*,*,#15731,.T.);
#22586=ORIENTED_EDGE('',*,*,#15754,.F.);
#22587=ORIENTED_EDGE('',*,*,#16257,.T.);
#22588=ORIENTED_EDGE('',*,*,#16131,.T.);
#22589=ORIENTED_EDGE('',*,*,#16258,.T.);
#22590=ORIENTED_EDGE('',*,*,#15882,.T.);
#22591=ORIENTED_EDGE('',*,*,#16130,.T.);
#22592=ORIENTED_EDGE('',*,*,#16259,.T.);
#22593=ORIENTED_EDGE('',*,*,#15881,.T.);
#22594=ORIENTED_EDGE('',*,*,#16258,.F.);
#22595=ORIENTED_EDGE('',*,*,#15764,.F.);
#22596=ORIENTED_EDGE('',*,*,#15879,.T.);
#22597=ORIENTED_EDGE('',*,*,#16259,.F.);
#22598=ORIENTED_EDGE('',*,*,#16129,.T.);
#22599=ORIENTED_EDGE('',*,*,#16260,.T.);
#22600=ORIENTED_EDGE('',*,*,#15739,.F.);
#22601=ORIENTED_EDGE('',*,*,#16256,.F.);
#22602=ORIENTED_EDGE('',*,*,#16132,.T.);
#22603=ORIENTED_EDGE('',*,*,#16257,.F.);
#22604=ORIENTED_EDGE('',*,*,#15753,.F.);
#22605=ORIENTED_EDGE('',*,*,#15751,.T.);
#22606=ORIENTED_EDGE('',*,*,#15774,.F.);
#22607=ORIENTED_EDGE('',*,*,#16261,.T.);
#22608=ORIENTED_EDGE('',*,*,#16127,.T.);
#22609=ORIENTED_EDGE('',*,*,#16262,.T.);
#22610=ORIENTED_EDGE('',*,*,#15876,.T.);
#22611=ORIENTED_EDGE('',*,*,#16126,.T.);
#22612=ORIENTED_EDGE('',*,*,#16263,.T.);
#22613=ORIENTED_EDGE('',*,*,#15875,.T.);
#22614=ORIENTED_EDGE('',*,*,#16262,.F.);
#22615=ORIENTED_EDGE('',*,*,#15784,.F.);
#22616=ORIENTED_EDGE('',*,*,#15787,.T.);
#22617=ORIENTED_EDGE('',*,*,#16263,.F.);
#22618=ORIENTED_EDGE('',*,*,#16125,.T.);
#22619=ORIENTED_EDGE('',*,*,#15804,.T.);
#22620=ORIENTED_EDGE('',*,*,#16124,.T.);
#22621=ORIENTED_EDGE('',*,*,#16264,.T.);
#22622=ORIENTED_EDGE('',*,*,#15872,.T.);
#22623=ORIENTED_EDGE('',*,*,#15803,.F.);
#22624=ORIENTED_EDGE('',*,*,#15812,.F.);
#22625=ORIENTED_EDGE('',*,*,#15871,.T.);
#22626=ORIENTED_EDGE('',*,*,#16264,.F.);
#22627=ORIENTED_EDGE('',*,*,#16123,.T.);
#22628=ORIENTED_EDGE('',*,*,#16265,.T.);
#22629=ORIENTED_EDGE('',*,*,#15822,.F.);
#22630=ORIENTED_EDGE('',*,*,#16266,.T.);
#22631=ORIENTED_EDGE('',*,*,#16121,.T.);
#22632=ORIENTED_EDGE('',*,*,#16267,.T.);
#22633=ORIENTED_EDGE('',*,*,#15867,.T.);
#22634=ORIENTED_EDGE('',*,*,#16120,.T.);
#22635=ORIENTED_EDGE('',*,*,#16268,.T.);
#22636=ORIENTED_EDGE('',*,*,#15866,.T.);
#22637=ORIENTED_EDGE('',*,*,#16267,.F.);
#22638=ORIENTED_EDGE('',*,*,#15832,.F.);
#22639=ORIENTED_EDGE('',*,*,#15864,.T.);
#22640=ORIENTED_EDGE('',*,*,#16268,.F.);
#22641=ORIENTED_EDGE('',*,*,#16119,.T.);
#22642=ORIENTED_EDGE('',*,*,#16269,.T.);
#22643=ORIENTED_EDGE('',*,*,#15807,.F.);
#22644=ORIENTED_EDGE('',*,*,#16265,.F.);
#22645=ORIENTED_EDGE('',*,*,#16122,.T.);
#22646=ORIENTED_EDGE('',*,*,#16266,.F.);
#22647=ORIENTED_EDGE('',*,*,#15821,.F.);
#22648=ORIENTED_EDGE('',*,*,#15819,.T.);
#22649=ORIENTED_EDGE('',*,*,#15842,.F.);
#22650=ORIENTED_EDGE('',*,*,#16270,.T.);
#22651=ORIENTED_EDGE('',*,*,#16117,.T.);
#22652=ORIENTED_EDGE('',*,*,#16271,.T.);
#22653=ORIENTED_EDGE('',*,*,#15861,.T.);
#22654=ORIENTED_EDGE('',*,*,#16116,.T.);
#22655=ORIENTED_EDGE('',*,*,#15852,.T.);
#22656=ORIENTED_EDGE('',*,*,#15860,.T.);
#22657=ORIENTED_EDGE('',*,*,#16271,.F.);
#22658=ORIENTED_EDGE('',*,*,#15827,.F.);
#22659=ORIENTED_EDGE('',*,*,#16269,.F.);
#22660=ORIENTED_EDGE('',*,*,#16118,.T.);
#22661=ORIENTED_EDGE('',*,*,#16270,.F.);
#22662=ORIENTED_EDGE('',*,*,#15841,.F.);
#22663=ORIENTED_EDGE('',*,*,#15839,.T.);
#22664=ORIENTED_EDGE('',*,*,#15140,.F.);
#22665=ORIENTED_EDGE('',*,*,#16272,.T.);
#22666=ORIENTED_EDGE('',*,*,#16114,.T.);
#22667=ORIENTED_EDGE('',*,*,#16273,.T.);
#22668=ORIENTED_EDGE('',*,*,#15718,.T.);
#22669=ORIENTED_EDGE('',*,*,#16113,.T.);
#22670=ORIENTED_EDGE('',*,*,#16274,.T.);
#22671=ORIENTED_EDGE('',*,*,#15717,.T.);
#22672=ORIENTED_EDGE('',*,*,#16273,.F.);
#22673=ORIENTED_EDGE('',*,*,#15158,.F.);
#22674=ORIENTED_EDGE('',*,*,#15715,.T.);
#22675=ORIENTED_EDGE('',*,*,#16274,.F.);
#22676=ORIENTED_EDGE('',*,*,#16112,.T.);
#22677=ORIENTED_EDGE('',*,*,#16275,.T.);
#22678=ORIENTED_EDGE('',*,*,#15139,.F.);
#22679=ORIENTED_EDGE('',*,*,#15145,.T.);
#22680=ORIENTED_EDGE('',*,*,#15847,.F.);
#22681=ORIENTED_EDGE('',*,*,#15854,.F.);
#22682=ORIENTED_EDGE('',*,*,#16115,.T.);
#22683=ORIENTED_EDGE('',*,*,#16272,.F.);
#22684=ORIENTED_EDGE('',*,*,#15170,.F.);
#22685=ORIENTED_EDGE('',*,*,#16276,.T.);
#22686=ORIENTED_EDGE('',*,*,#16110,.T.);
#22687=ORIENTED_EDGE('',*,*,#16277,.T.);
#22688=ORIENTED_EDGE('',*,*,#15712,.T.);
#22689=ORIENTED_EDGE('',*,*,#16109,.T.);
#22690=ORIENTED_EDGE('',*,*,#16278,.T.);
#22691=ORIENTED_EDGE('',*,*,#15711,.T.);
#22692=ORIENTED_EDGE('',*,*,#16277,.F.);
#22693=ORIENTED_EDGE('',*,*,#15181,.F.);
#22694=ORIENTED_EDGE('',*,*,#15184,.T.);
#22695=ORIENTED_EDGE('',*,*,#16278,.F.);
#22696=ORIENTED_EDGE('',*,*,#16108,.T.);
#22697=ORIENTED_EDGE('',*,*,#16279,.T.);
#22698=ORIENTED_EDGE('',*,*,#15153,.F.);
#22699=ORIENTED_EDGE('',*,*,#16275,.F.);
#22700=ORIENTED_EDGE('',*,*,#16111,.T.);
#22701=ORIENTED_EDGE('',*,*,#16276,.F.);
#22702=ORIENTED_EDGE('',*,*,#15169,.F.);
#22703=ORIENTED_EDGE('',*,*,#15167,.T.);
#22704=ORIENTED_EDGE('',*,*,#16106,.T.);
#22705=ORIENTED_EDGE('',*,*,#16280,.T.);
#22706=ORIENTED_EDGE('',*,*,#15708,.T.);
#22707=ORIENTED_EDGE('',*,*,#15037,.F.);
#22708=ORIENTED_EDGE('',*,*,#15195,.F.);
#22709=ORIENTED_EDGE('',*,*,#15707,.T.);
#22710=ORIENTED_EDGE('',*,*,#16280,.F.);
#22711=ORIENTED_EDGE('',*,*,#16105,.T.);
#22712=ORIENTED_EDGE('',*,*,#16281,.T.);
#22713=ORIENTED_EDGE('',*,*,#15025,.F.);
#22714=ORIENTED_EDGE('',*,*,#16282,.T.);
#22715=ORIENTED_EDGE('',*,*,#15176,.F.);
#22716=ORIENTED_EDGE('',*,*,#16279,.F.);
#22717=ORIENTED_EDGE('',*,*,#16107,.T.);
#22718=ORIENTED_EDGE('',*,*,#15035,.F.);
#22719=ORIENTED_EDGE('',*,*,#15207,.F.);
#22720=ORIENTED_EDGE('',*,*,#16283,.T.);
#22721=ORIENTED_EDGE('',*,*,#16103,.T.);
#22722=ORIENTED_EDGE('',*,*,#16284,.T.);
#22723=ORIENTED_EDGE('',*,*,#15704,.T.);
#22724=ORIENTED_EDGE('',*,*,#15703,.T.);
#22725=ORIENTED_EDGE('',*,*,#16284,.F.);
#22726=ORIENTED_EDGE('',*,*,#16102,.T.);
#22727=ORIENTED_EDGE('',*,*,#16285,.T.);
#22728=ORIENTED_EDGE('',*,*,#15218,.F.);
#22729=ORIENTED_EDGE('',*,*,#15221,.T.);
#22730=ORIENTED_EDGE('',*,*,#16285,.F.);
#22731=ORIENTED_EDGE('',*,*,#16101,.T.);
#22732=ORIENTED_EDGE('',*,*,#15240,.T.);
#22733=ORIENTED_EDGE('',*,*,#16100,.T.);
#22734=ORIENTED_EDGE('',*,*,#16286,.T.);
#22735=ORIENTED_EDGE('',*,*,#15700,.T.);
#22736=ORIENTED_EDGE('',*,*,#15239,.F.);
#22737=ORIENTED_EDGE('',*,*,#15248,.F.);
#22738=ORIENTED_EDGE('',*,*,#15699,.T.);
#22739=ORIENTED_EDGE('',*,*,#16286,.F.);
#22740=ORIENTED_EDGE('',*,*,#16099,.T.);
#22741=ORIENTED_EDGE('',*,*,#16287,.T.);
#22742=ORIENTED_EDGE('',*,*,#15260,.F.);
#22743=ORIENTED_EDGE('',*,*,#16288,.T.);
#22744=ORIENTED_EDGE('',*,*,#16097,.T.);
#22745=ORIENTED_EDGE('',*,*,#16289,.T.);
#22746=ORIENTED_EDGE('',*,*,#15695,.T.);
#22747=ORIENTED_EDGE('',*,*,#16096,.T.);
#22748=ORIENTED_EDGE('',*,*,#16290,.T.);
#22749=ORIENTED_EDGE('',*,*,#15694,.T.);
#22750=ORIENTED_EDGE('',*,*,#16289,.F.);
#22751=ORIENTED_EDGE('',*,*,#15271,.F.);
#22752=ORIENTED_EDGE('',*,*,#15692,.T.);
#22753=ORIENTED_EDGE('',*,*,#16290,.F.);
#22754=ORIENTED_EDGE('',*,*,#16095,.T.);
#22755=ORIENTED_EDGE('',*,*,#16291,.T.);
#22756=ORIENTED_EDGE('',*,*,#15243,.F.);
#22757=ORIENTED_EDGE('',*,*,#16287,.F.);
#22758=ORIENTED_EDGE('',*,*,#16098,.T.);
#22759=ORIENTED_EDGE('',*,*,#16288,.F.);
#22760=ORIENTED_EDGE('',*,*,#15259,.F.);
#22761=ORIENTED_EDGE('',*,*,#15257,.T.);
#22762=ORIENTED_EDGE('',*,*,#15283,.F.);
#22763=ORIENTED_EDGE('',*,*,#16292,.T.);
#22764=ORIENTED_EDGE('',*,*,#16093,.T.);
#22765=ORIENTED_EDGE('',*,*,#16293,.T.);
#22766=ORIENTED_EDGE('',*,*,#15689,.T.);
#22767=ORIENTED_EDGE('',*,*,#16092,.T.);
#22768=ORIENTED_EDGE('',*,*,#15296,.T.);
#22769=ORIENTED_EDGE('',*,*,#15688,.T.);
#22770=ORIENTED_EDGE('',*,*,#16293,.F.);
#22771=ORIENTED_EDGE('',*,*,#15266,.F.);
#22772=ORIENTED_EDGE('',*,*,#16291,.F.);
#22773=ORIENTED_EDGE('',*,*,#16094,.T.);
#22774=ORIENTED_EDGE('',*,*,#16292,.F.);
#22775=ORIENTED_EDGE('',*,*,#15282,.F.);
#22776=ORIENTED_EDGE('',*,*,#15280,.T.);
#22777=ORIENTED_EDGE('',*,*,#15377,.F.);
#22778=ORIENTED_EDGE('',*,*,#15372,.T.);
#22779=ORIENTED_EDGE('',*,*,#16294,.T.);
#22780=ORIENTED_EDGE('',*,*,#16295,.T.);
#22781=ORIENTED_EDGE('',*,*,#16090,.T.);
#22782=ORIENTED_EDGE('',*,*,#15651,.T.);
#22783=ORIENTED_EDGE('',*,*,#15655,.F.);
#22784=ORIENTED_EDGE('',*,*,#16296,.T.);
#22785=ORIENTED_EDGE('',*,*,#16088,.T.);
#22786=ORIENTED_EDGE('',*,*,#16297,.T.);
#22787=ORIENTED_EDGE('',*,*,#15685,.T.);
#22788=ORIENTED_EDGE('',*,*,#16087,.T.);
#22789=ORIENTED_EDGE('',*,*,#16298,.T.);
#22790=ORIENTED_EDGE('',*,*,#15684,.T.);
#22791=ORIENTED_EDGE('',*,*,#16297,.F.);
#22792=ORIENTED_EDGE('',*,*,#15665,.F.);
#22793=ORIENTED_EDGE('',*,*,#15682,.T.);
#22794=ORIENTED_EDGE('',*,*,#16298,.F.);
#22795=ORIENTED_EDGE('',*,*,#16086,.T.);
#22796=ORIENTED_EDGE('',*,*,#16299,.T.);
#22797=ORIENTED_EDGE('',*,*,#15396,.F.);
#22798=ORIENTED_EDGE('',*,*,#15650,.F.);
#22799=ORIENTED_EDGE('',*,*,#16089,.T.);
#22800=ORIENTED_EDGE('',*,*,#16296,.F.);
#22801=ORIENTED_EDGE('',*,*,#15654,.F.);
#22802=ORIENTED_EDGE('',*,*,#15407,.T.);
#22803=ORIENTED_EDGE('',*,*,#15675,.F.);
#22804=ORIENTED_EDGE('',*,*,#16300,.T.);
#22805=ORIENTED_EDGE('',*,*,#16084,.T.);
#22806=ORIENTED_EDGE('',*,*,#16301,.T.);
#22807=ORIENTED_EDGE('',*,*,#15679,.T.);
#22808=ORIENTED_EDGE('',*,*,#16083,.T.);
#22809=ORIENTED_EDGE('',*,*,#16302,.T.);
#22810=ORIENTED_EDGE('',*,*,#15634,.T.);
#22811=ORIENTED_EDGE('',*,*,#16301,.F.);
#22812=ORIENTED_EDGE('',*,*,#15414,.F.);
#22813=ORIENTED_EDGE('',*,*,#15632,.T.);
#22814=ORIENTED_EDGE('',*,*,#16302,.F.);
#22815=ORIENTED_EDGE('',*,*,#16082,.T.);
#22816=ORIENTED_EDGE('',*,*,#16196,.T.);
#22817=ORIENTED_EDGE('',*,*,#15660,.F.);
#22818=ORIENTED_EDGE('',*,*,#16299,.F.);
#22819=ORIENTED_EDGE('',*,*,#16085,.T.);
#22820=ORIENTED_EDGE('',*,*,#16300,.F.);
#22821=ORIENTED_EDGE('',*,*,#15674,.F.);
#22822=ORIENTED_EDGE('',*,*,#15672,.T.);
#22823=ORIENTED_EDGE('',*,*,#16303,.T.);
#22824=ORIENTED_EDGE('',*,*,#16304,.T.);
#22825=ORIENTED_EDGE('',*,*,#16305,.T.);
#22826=ORIENTED_EDGE('',*,*,#16303,.F.);
#22827=ORIENTED_EDGE('',*,*,#16306,.T.);
#22828=ORIENTED_EDGE('',*,*,#16307,.F.);
#22829=ORIENTED_EDGE('',*,*,#16308,.T.);
#22830=ORIENTED_EDGE('',*,*,#16304,.F.);
#22831=ORIENTED_EDGE('',*,*,#16305,.F.);
#22832=ORIENTED_EDGE('',*,*,#16308,.F.);
#22833=ORIENTED_EDGE('',*,*,#16309,.F.);
#22834=ORIENTED_EDGE('',*,*,#16310,.T.);
#22835=ORIENTED_EDGE('',*,*,#16311,.T.);
#22836=ORIENTED_EDGE('',*,*,#16310,.F.);
#22837=ORIENTED_EDGE('',*,*,#16306,.F.);
#22838=ORIENTED_EDGE('',*,*,#16195,.T.);
#22839=ORIENTED_EDGE('',*,*,#16312,.T.);
#22840=ORIENTED_EDGE('',*,*,#16307,.T.);
#22841=ORIENTED_EDGE('',*,*,#16312,.F.);
#22842=ORIENTED_EDGE('',*,*,#15370,.T.);
#22843=ORIENTED_EDGE('',*,*,#16313,.T.);
#22844=ORIENTED_EDGE('',*,*,#16309,.T.);
#22845=ORIENTED_EDGE('',*,*,#16313,.F.);
#22846=ORIENTED_EDGE('',*,*,#16311,.F.);
#22847=ORIENTED_EDGE('',*,*,#16314,.T.);
#22848=ORIENTED_EDGE('',*,*,#16314,.F.);
#22849=ORIENTED_EDGE('',*,*,#15291,.F.);
#22850=ORIENTED_EDGE('',*,*,#16315,.T.);
#22851=ORIENTED_EDGE('',*,*,#16316,.T.);
#22852=ORIENTED_EDGE('',*,*,#15385,.F.);
#22853=ORIENTED_EDGE('',*,*,#15596,.T.);
#22854=ORIENTED_EDGE('',*,*,#15301,.F.);
#22855=ORIENTED_EDGE('',*,*,#15053,.F.);
#22856=ORIENTED_EDGE('',*,*,#16073,.F.);
#22857=ORIENTED_EDGE('',*,*,#15532,.T.);
#22858=ORIENTED_EDGE('',*,*,#15360,.F.);
#22859=ORIENTED_EDGE('',*,*,#15351,.F.);
#22860=ORIENTED_EDGE('',*,*,#16317,.T.);
#22861=ORIENTED_EDGE('',*,*,#15290,.F.);
#22862=ORIENTED_EDGE('',*,*,#16318,.F.);
#22863=ORIENTED_EDGE('',*,*,#16319,.F.);
#22864=ORIENTED_EDGE('',*,*,#16315,.F.);
#22865=ORIENTED_EDGE('',*,*,#15070,.F.);
#22866=ORIENTED_EDGE('',*,*,#15514,.F.);
#22867=ORIENTED_EDGE('',*,*,#15502,.F.);
#22868=ORIENTED_EDGE('',*,*,#16211,.F.);
#22869=ORIENTED_EDGE('',*,*,#15024,.F.);
#22870=ORIENTED_EDGE('',*,*,#15189,.F.);
#22871=ORIENTED_EDGE('',*,*,#15177,.F.);
#22872=ORIENTED_EDGE('',*,*,#16282,.F.);
#22873=ORIENTED_EDGE('',*,*,#15214,.F.);
#22874=ORIENTED_EDGE('',*,*,#15242,.F.);
#22875=ORIENTED_EDGE('',*,*,#15229,.F.);
#22876=ORIENTED_EDGE('',*,*,#15225,.F.);
#22877=ORIENTED_EDGE('',*,*,#15780,.F.);
#22878=ORIENTED_EDGE('',*,*,#15806,.F.);
#22879=ORIENTED_EDGE('',*,*,#15793,.F.);
#22880=ORIENTED_EDGE('',*,*,#15790,.F.);
#22881=ORIENTED_EDGE('',*,*,#15039,.F.);
#22882=ORIENTED_EDGE('',*,*,#15136,.F.);
#22883=ORIENTED_EDGE('',*,*,#15124,.F.);
#22884=ORIENTED_EDGE('',*,*,#16252,.F.);
#22885=ORIENTED_EDGE('',*,*,#15054,.F.);
#22886=ORIENTED_EDGE('',*,*,#16317,.F.);
#22887=ORIENTED_EDGE('',*,*,#15350,.F.);
#22888=ORIENTED_EDGE('',*,*,#15065,.F.);
#22889=ORIENTED_EDGE('',*,*,#15289,.F.);
#22890=ORIENTED_EDGE('',*,*,#15298,.F.);
#22891=ORIENTED_EDGE('',*,*,#16091,.T.);
#22892=ORIENTED_EDGE('',*,*,#16295,.F.);
#22893=ORIENTED_EDGE('',*,*,#16320,.T.);
#22894=ORIENTED_EDGE('',*,*,#16318,.T.);
#22895=ORIENTED_EDGE('',*,*,#15327,.F.);
#22896=ORIENTED_EDGE('',*,*,#16215,.F.);
#22897=ORIENTED_EDGE('',*,*,#16175,.T.);
#22898=ORIENTED_EDGE('',*,*,#16216,.F.);
#22899=ORIENTED_EDGE('',*,*,#15343,.F.);
#22900=ORIENTED_EDGE('',*,*,#15341,.T.);
#22901=ORIENTED_EDGE('',*,*,#15759,.F.);
#22902=ORIENTED_EDGE('',*,*,#16260,.F.);
#22903=ORIENTED_EDGE('',*,*,#16128,.T.);
#22904=ORIENTED_EDGE('',*,*,#16261,.F.);
#22905=ORIENTED_EDGE('',*,*,#15773,.F.);
#22906=ORIENTED_EDGE('',*,*,#15771,.T.);
#22907=ORIENTED_EDGE('',*,*,#15190,.F.);
#22908=ORIENTED_EDGE('',*,*,#16281,.F.);
#22909=ORIENTED_EDGE('',*,*,#16104,.T.);
#22910=ORIENTED_EDGE('',*,*,#16283,.F.);
#22911=ORIENTED_EDGE('',*,*,#15206,.F.);
#22912=ORIENTED_EDGE('',*,*,#15204,.T.);
#22913=ORIENTED_EDGE('',*,*,#15635,.F.);
#22914=ORIENTED_EDGE('',*,*,#16321,.T.);
#22915=ORIENTED_EDGE('',*,*,#16322,.T.);
#22916=ORIENTED_EDGE('',*,*,#15402,.F.);
#22917=ORIENTED_EDGE('',*,*,#15643,.F.);
#22918=ORIENTED_EDGE('',*,*,#15364,.F.);
#22919=ORIENTED_EDGE('',*,*,#16323,.T.);
#22920=ORIENTED_EDGE('',*,*,#15386,.F.);
#22921=ORIENTED_EDGE('',*,*,#16316,.F.);
#22922=ORIENTED_EDGE('',*,*,#16319,.T.);
#22923=ORIENTED_EDGE('',*,*,#16320,.F.);
#22924=ORIENTED_EDGE('',*,*,#16294,.F.);
#22925=ORIENTED_EDGE('',*,*,#15371,.F.);
#22926=ORIENTED_EDGE('',*,*,#15394,.F.);
#22927=ORIENTED_EDGE('',*,*,#16322,.F.);
#22928=ORIENTED_EDGE('',*,*,#16324,.T.);
#22929=ORIENTED_EDGE('',*,*,#15641,.T.);
#22930=ORIENTED_EDGE('',*,*,#15363,.F.);
#22931=ORIENTED_EDGE('',*,*,#15369,.T.);
#22932=ORIENTED_EDGE('',*,*,#15392,.F.);
#22933=ORIENTED_EDGE('',*,*,#15381,.F.);
#22934=ORIENTED_EDGE('',*,*,#15387,.F.);
#22935=ORIENTED_EDGE('',*,*,#16323,.F.);
#22936=ORIENTED_EDGE('',*,*,#15638,.F.);
#22937=ORIENTED_EDGE('',*,*,#15642,.F.);
#22938=ORIENTED_EDGE('',*,*,#16324,.F.);
#22939=ORIENTED_EDGE('',*,*,#16321,.F.);
#22940=ORIENTED_EDGE('',*,*,#15379,.F.);
#22941=ORIENTED_EDGE('',*,*,#15653,.F.);
#22942=ORIENTED_EDGE('',*,*,#15646,.F.);
#22943=ORIENTED_EDGE('',*,*,#15388,.F.);
#25344=CONICAL_SURFACE('',#28283,0.855,0.785398163397457);
#25345=CONICAL_SURFACE('',#28284,1.83,0.785398163397454);
#25346=CONICAL_SURFACE('',#28285,1.755,1.02974425867665);
#25936=ADVANCED_FACE('',(#3123),#1916,.T.);
#25937=ADVANCED_FACE('',(#3124),#1917,.T.);
#25938=ADVANCED_FACE('',(#3125),#1918,.F.);
#25939=ADVANCED_FACE('',(#3126),#1919,.T.);
#25940=ADVANCED_FACE('',(#3127),#1920,.T.);
#25941=ADVANCED_FACE('',(#3128),#1921,.T.);
#25942=ADVANCED_FACE('',(#3129),#1922,.F.);
#25943=ADVANCED_FACE('',(#3130),#1923,.T.);
#25944=ADVANCED_FACE('',(#3131),#1924,.T.);
#25945=ADVANCED_FACE('',(#3132),#1925,.F.);
#25946=ADVANCED_FACE('',(#3133),#1926,.T.);
#25947=ADVANCED_FACE('',(#3134),#1927,.T.);
#25948=ADVANCED_FACE('',(#3135),#1928,.T.);
#25949=ADVANCED_FACE('',(#3136),#1929,.T.);
#25950=ADVANCED_FACE('',(#3137),#1930,.F.);
#25951=ADVANCED_FACE('',(#3138),#1931,.T.);
#25952=ADVANCED_FACE('',(#3139),#1932,.T.);
#25953=ADVANCED_FACE('',(#3140),#1933,.T.);
#25954=ADVANCED_FACE('',(#3141),#1934,.T.);
#25955=ADVANCED_FACE('',(#3142),#1935,.T.);
#25956=ADVANCED_FACE('',(#3143),#1936,.T.);
#25957=ADVANCED_FACE('',(#3144),#1937,.T.);
#25958=ADVANCED_FACE('',(#3145),#1938,.T.);
#25959=ADVANCED_FACE('',(#3146),#1939,.T.);
#25960=ADVANCED_FACE('',(#3147),#1940,.T.);
#25961=ADVANCED_FACE('',(#3148),#1941,.T.);
#25962=ADVANCED_FACE('',(#3149),#1942,.T.);
#25963=ADVANCED_FACE('',(#3150),#1943,.F.);
#25964=ADVANCED_FACE('',(#3151),#1944,.T.);
#25965=ADVANCED_FACE('',(#3152),#1945,.T.);
#25966=ADVANCED_FACE('',(#3153),#1946,.T.);
#25967=ADVANCED_FACE('',(#3154),#1947,.T.);
#25968=ADVANCED_FACE('',(#3155),#1948,.T.);
#25969=ADVANCED_FACE('',(#3156),#1949,.T.);
#25970=ADVANCED_FACE('',(#3157),#1950,.T.);
#25971=ADVANCED_FACE('',(#3158),#1951,.T.);
#25972=ADVANCED_FACE('',(#3159),#1952,.T.);
#25973=ADVANCED_FACE('',(#3160),#1953,.T.);
#25974=ADVANCED_FACE('',(#3161),#1954,.T.);
#25975=ADVANCED_FACE('',(#3162),#1955,.T.);
#25976=ADVANCED_FACE('',(#3163),#1956,.T.);
#25977=ADVANCED_FACE('',(#3164),#1957,.F.);
#25978=ADVANCED_FACE('',(#3165),#1958,.T.);
#25979=ADVANCED_FACE('',(#3166),#1959,.T.);
#25980=ADVANCED_FACE('',(#3167),#1960,.T.);
#25981=ADVANCED_FACE('',(#3168),#1961,.T.);
#25982=ADVANCED_FACE('',(#3169),#1962,.T.);
#25983=ADVANCED_FACE('',(#3170),#1963,.T.);
#25984=ADVANCED_FACE('',(#3171),#1964,.T.);
#25985=ADVANCED_FACE('',(#3172),#1965,.T.);
#25986=ADVANCED_FACE('',(#3173),#1966,.T.);
#25987=ADVANCED_FACE('',(#3174),#1967,.F.);
#25988=ADVANCED_FACE('',(#3175),#1968,.T.);
#25989=ADVANCED_FACE('',(#3176),#1969,.T.);
#25990=ADVANCED_FACE('',(#3177),#1970,.T.);
#25991=ADVANCED_FACE('',(#3178),#1971,.F.);
#25992=ADVANCED_FACE('',(#3179),#1972,.T.);
#25993=ADVANCED_FACE('',(#3180),#1973,.T.);
#25994=ADVANCED_FACE('',(#3181),#1974,.T.);
#25995=ADVANCED_FACE('',(#3182),#1975,.T.);
#25996=ADVANCED_FACE('',(#3183),#1976,.T.);
#25997=ADVANCED_FACE('',(#3184),#1977,.T.);
#25998=ADVANCED_FACE('',(#3185),#1978,.T.);
#25999=ADVANCED_FACE('',(#3186),#1979,.T.);
#26000=ADVANCED_FACE('',(#3187),#1980,.T.);
#26001=ADVANCED_FACE('',(#3188),#1981,.T.);
#26002=ADVANCED_FACE('',(#3189),#1982,.T.);
#26003=ADVANCED_FACE('',(#3190),#1983,.T.);
#26004=ADVANCED_FACE('',(#3191),#1984,.T.);
#26005=ADVANCED_FACE('',(#3192),#1985,.T.);
#26006=ADVANCED_FACE('',(#3193),#1986,.T.);
#26007=ADVANCED_FACE('',(#3194),#1987,.T.);
#26008=ADVANCED_FACE('',(#3195),#1988,.F.);
#26009=ADVANCED_FACE('',(#3196),#1989,.T.);
#26010=ADVANCED_FACE('',(#3197),#1990,.T.);
#26011=ADVANCED_FACE('',(#3198),#1991,.T.);
#26012=ADVANCED_FACE('',(#3199),#1992,.T.);
#26013=ADVANCED_FACE('',(#3200),#1993,.T.);
#26014=ADVANCED_FACE('',(#3201),#1994,.T.);
#26015=ADVANCED_FACE('',(#3202),#1995,.T.);
#26016=ADVANCED_FACE('',(#3203),#1996,.T.);
#26017=ADVANCED_FACE('',(#3204),#1997,.T.);
#26018=ADVANCED_FACE('',(#3205),#1998,.T.);
#26019=ADVANCED_FACE('',(#3206),#1999,.T.);
#26020=ADVANCED_FACE('',(#3207),#2000,.T.);
#26021=ADVANCED_FACE('',(#3208),#2001,.T.);
#26022=ADVANCED_FACE('',(#3209),#2002,.T.);
#26023=ADVANCED_FACE('',(#3210),#2003,.T.);
#26024=ADVANCED_FACE('',(#3211),#2004,.F.);
#26025=ADVANCED_FACE('',(#3212),#2005,.T.);
#26026=ADVANCED_FACE('',(#3213),#2006,.T.);
#26027=ADVANCED_FACE('',(#3214,#875),#2007,.F.);
#26028=ADVANCED_FACE('',(#3215),#2008,.T.);
#26029=ADVANCED_FACE('',(#3216),#2009,.T.);
#26030=ADVANCED_FACE('',(#3217),#2010,.T.);
#26031=ADVANCED_FACE('',(#3218),#2011,.T.);
#26032=ADVANCED_FACE('',(#3219),#2012,.T.);
#26033=ADVANCED_FACE('',(#3220),#2013,.T.);
#26034=ADVANCED_FACE('',(#3221),#2014,.T.);
#26035=ADVANCED_FACE('',(#3222),#2015,.T.);
#26036=ADVANCED_FACE('',(#3223),#2016,.T.);
#26037=ADVANCED_FACE('',(#3224),#2017,.T.);
#26038=ADVANCED_FACE('',(#3225),#2018,.T.);
#26039=ADVANCED_FACE('',(#3226),#2019,.T.);
#26040=ADVANCED_FACE('',(#3227),#2020,.T.);
#26041=ADVANCED_FACE('',(#3228),#2021,.T.);
#26042=ADVANCED_FACE('',(#3229),#2022,.T.);
#26043=ADVANCED_FACE('',(#3230),#2023,.T.);
#26044=ADVANCED_FACE('',(#3231),#2024,.T.);
#26045=ADVANCED_FACE('',(#3232),#2025,.T.);
#26046=ADVANCED_FACE('',(#3233),#2026,.T.);
#26047=ADVANCED_FACE('',(#3234),#2027,.T.);
#26048=ADVANCED_FACE('',(#3235),#2028,.T.);
#26049=ADVANCED_FACE('',(#3236),#2029,.T.);
#26050=ADVANCED_FACE('',(#3237),#2030,.T.);
#26051=ADVANCED_FACE('',(#3238),#2031,.T.);
#26052=ADVANCED_FACE('',(#3239),#2032,.T.);
#26053=ADVANCED_FACE('',(#3240),#2033,.T.);
#26054=ADVANCED_FACE('',(#3241),#2034,.T.);
#26055=ADVANCED_FACE('',(#3242),#2035,.T.);
#26056=ADVANCED_FACE('',(#3243),#2036,.T.);
#26057=ADVANCED_FACE('',(#3244),#2037,.T.);
#26058=ADVANCED_FACE('',(#3245),#2038,.T.);
#26059=ADVANCED_FACE('',(#3246),#2039,.T.);
#26060=ADVANCED_FACE('',(#3247),#2040,.T.);
#26061=ADVANCED_FACE('',(#3248),#2041,.T.);
#26062=ADVANCED_FACE('',(#3249),#2042,.T.);
#26063=ADVANCED_FACE('',(#3250),#2043,.F.);
#26064=ADVANCED_FACE('',(#3251),#2044,.T.);
#26065=ADVANCED_FACE('',(#3252),#2045,.T.);
#26066=ADVANCED_FACE('',(#3253),#2046,.T.);
#26067=ADVANCED_FACE('',(#3254),#2047,.F.);
#26068=ADVANCED_FACE('',(#3255),#2048,.F.);
#26069=ADVANCED_FACE('',(#3256),#2049,.T.);
#26070=ADVANCED_FACE('',(#3257),#2050,.F.);
#26071=ADVANCED_FACE('',(#3258),#2051,.F.);
#26072=ADVANCED_FACE('',(#3259),#2052,.F.);
#26073=ADVANCED_FACE('',(#3260),#2053,.T.);
#26074=ADVANCED_FACE('',(#3261),#2054,.F.);
#26075=ADVANCED_FACE('',(#3262),#2055,.F.);
#26076=ADVANCED_FACE('',(#3263),#2056,.T.);
#26077=ADVANCED_FACE('',(#3264),#2057,.T.);
#26078=ADVANCED_FACE('',(#3265),#2058,.F.);
#26079=ADVANCED_FACE('',(#3266),#2059,.F.);
#26080=ADVANCED_FACE('',(#3267),#2060,.T.);
#26081=ADVANCED_FACE('',(#3268),#2061,.F.);
#26082=ADVANCED_FACE('',(#3269),#2062,.F.);
#26083=ADVANCED_FACE('',(#3270),#2063,.F.);
#26084=ADVANCED_FACE('',(#3271),#2064,.T.);
#26085=ADVANCED_FACE('',(#3272),#2065,.F.);
#26086=ADVANCED_FACE('',(#3273),#2066,.F.);
#26087=ADVANCED_FACE('',(#3274),#2067,.F.);
#26088=ADVANCED_FACE('',(#3275),#2068,.T.);
#26089=ADVANCED_FACE('',(#3276),#2069,.F.);
#26090=ADVANCED_FACE('',(#3277),#2070,.F.);
#26091=ADVANCED_FACE('',(#3278),#2071,.F.);
#26092=ADVANCED_FACE('',(#3279),#2072,.T.);
#26093=ADVANCED_FACE('',(#3280),#2073,.F.);
#26094=ADVANCED_FACE('',(#3281),#2074,.F.);
#26095=ADVANCED_FACE('',(#3282),#2075,.T.);
#26096=ADVANCED_FACE('',(#3283),#2076,.T.);
#26097=ADVANCED_FACE('',(#3284),#2077,.T.);
#26098=ADVANCED_FACE('',(#3285),#2078,.T.);
#26099=ADVANCED_FACE('',(#3286),#2079,.T.);
#26100=ADVANCED_FACE('',(#3287),#2080,.T.);
#26101=ADVANCED_FACE('',(#3288),#2081,.T.);
#26102=ADVANCED_FACE('',(#3289),#2082,.T.);
#26103=ADVANCED_FACE('',(#3290),#2083,.T.);
#26104=ADVANCED_FACE('',(#3291),#2084,.T.);
#26105=ADVANCED_FACE('',(#3292),#2085,.T.);
#26106=ADVANCED_FACE('',(#3293),#2086,.T.);
#26107=ADVANCED_FACE('',(#3294),#2087,.T.);
#26108=ADVANCED_FACE('',(#3295),#2088,.T.);
#26109=ADVANCED_FACE('',(#3296),#2089,.F.);
#26110=ADVANCED_FACE('',(#3297),#2090,.T.);
#26111=ADVANCED_FACE('',(#3298),#2091,.F.);
#26112=ADVANCED_FACE('',(#3299),#2092,.F.);
#26113=ADVANCED_FACE('',(#3300),#2093,.F.);
#26114=ADVANCED_FACE('',(#3301),#2094,.T.);
#26115=ADVANCED_FACE('',(#3302),#2095,.F.);
#26116=ADVANCED_FACE('',(#3303),#2096,.F.);
#26117=ADVANCED_FACE('',(#3304),#2097,.T.);
#26118=ADVANCED_FACE('',(#3305),#2098,.F.);
#26119=ADVANCED_FACE('',(#3306),#2099,.F.);
#26120=ADVANCED_FACE('',(#3307),#2100,.F.);
#26121=ADVANCED_FACE('',(#3308),#2101,.T.);
#26122=ADVANCED_FACE('',(#3309),#2102,.T.);
#26123=ADVANCED_FACE('',(#3310),#2103,.F.);
#26124=ADVANCED_FACE('',(#3311),#2104,.F.);
#26125=ADVANCED_FACE('',(#3312),#2105,.T.);
#26126=ADVANCED_FACE('',(#3313),#2106,.F.);
#26127=ADVANCED_FACE('',(#3314),#2107,.F.);
#26128=ADVANCED_FACE('',(#3315),#2108,.T.);
#26129=ADVANCED_FACE('',(#3316),#2109,.F.);
#26130=ADVANCED_FACE('',(#3317),#2110,.F.);
#26131=ADVANCED_FACE('',(#3318),#2111,.T.);
#26132=ADVANCED_FACE('',(#3319),#2112,.F.);
#26133=ADVANCED_FACE('',(#3320),#2113,.F.);
#26134=ADVANCED_FACE('',(#3321),#2114,.T.);
#26135=ADVANCED_FACE('',(#3322),#2115,.F.);
#26136=ADVANCED_FACE('',(#3323),#2116,.F.);
#26137=ADVANCED_FACE('',(#3324),#2117,.F.);
#26138=ADVANCED_FACE('',(#3325),#2118,.T.);
#26139=ADVANCED_FACE('',(#3326),#2119,.T.);
#26140=ADVANCED_FACE('',(#3327),#2120,.T.);
#26141=ADVANCED_FACE('',(#3328),#2121,.T.);
#26142=ADVANCED_FACE('',(#3329),#2122,.T.);
#26143=ADVANCED_FACE('',(#3330),#2123,.T.);
#26144=ADVANCED_FACE('',(#3331),#2124,.T.);
#26145=ADVANCED_FACE('',(#3332),#2125,.T.);
#26146=ADVANCED_FACE('',(#3333),#2126,.T.);
#26147=ADVANCED_FACE('',(#3334),#2127,.T.);
#26148=ADVANCED_FACE('',(#3335),#2128,.T.);
#26149=ADVANCED_FACE('',(#3336),#2129,.T.);
#26150=ADVANCED_FACE('',(#3337),#2130,.T.);
#26151=ADVANCED_FACE('',(#3338),#2131,.T.);
#26152=ADVANCED_FACE('',(#3339),#2132,.T.);
#26153=ADVANCED_FACE('',(#3340),#2133,.T.);
#26154=ADVANCED_FACE('',(#3341),#2134,.T.);
#26155=ADVANCED_FACE('',(#3342),#2135,.T.);
#26156=ADVANCED_FACE('',(#3343),#2136,.T.);
#26157=ADVANCED_FACE('',(#3344),#2137,.F.);
#26158=ADVANCED_FACE('',(#3345),#2138,.T.);
#26159=ADVANCED_FACE('',(#3346),#2139,.T.);
#26160=ADVANCED_FACE('',(#3347),#2140,.T.);
#26161=ADVANCED_FACE('',(#3348),#2141,.F.);
#26162=ADVANCED_FACE('',(#3349),#2142,.T.);
#26163=ADVANCED_FACE('',(#3350),#2143,.T.);
#26164=ADVANCED_FACE('',(#3351),#2144,.T.);
#26165=ADVANCED_FACE('',(#3352),#2145,.T.);
#26166=ADVANCED_FACE('',(#3353),#2146,.T.);
#26167=ADVANCED_FACE('',(#3354),#2147,.T.);
#26168=ADVANCED_FACE('',(#3355),#2148,.T.);
#26169=ADVANCED_FACE('',(#3356),#2149,.T.);
#26170=ADVANCED_FACE('',(#3357),#2150,.T.);
#26171=ADVANCED_FACE('',(#3358),#2151,.T.);
#26172=ADVANCED_FACE('',(#3359),#2152,.T.);
#26173=ADVANCED_FACE('',(#3360),#2153,.T.);
#26174=ADVANCED_FACE('',(#3361),#2154,.T.);
#26175=ADVANCED_FACE('',(#3362),#2155,.T.);
#26176=ADVANCED_FACE('',(#3363),#2156,.T.);
#26177=ADVANCED_FACE('',(#3364),#2157,.T.);
#26178=ADVANCED_FACE('',(#3365),#2158,.F.);
#26179=ADVANCED_FACE('',(#3366),#2159,.T.);
#26180=ADVANCED_FACE('',(#3367),#2160,.T.);
#26181=ADVANCED_FACE('',(#3368),#2161,.F.);
#26182=ADVANCED_FACE('',(#3369),#2162,.F.);
#26183=ADVANCED_FACE('',(#3370),#2163,.T.);
#26184=ADVANCED_FACE('',(#3371),#2164,.F.);
#26185=ADVANCED_FACE('',(#3372),#2165,.F.);
#26186=ADVANCED_FACE('',(#3373),#2166,.F.);
#26187=ADVANCED_FACE('',(#3374),#2167,.T.);
#26188=ADVANCED_FACE('',(#3375),#2168,.T.);
#26189=ADVANCED_FACE('',(#3376),#2169,.F.);
#26190=ADVANCED_FACE('',(#3377),#2170,.F.);
#26191=ADVANCED_FACE('',(#3378),#2171,.T.);
#26192=ADVANCED_FACE('',(#3379),#2172,.F.);
#26193=ADVANCED_FACE('',(#3380),#2173,.F.);
#26194=ADVANCED_FACE('',(#3381),#2174,.T.);
#26195=ADVANCED_FACE('',(#3382),#2175,.F.);
#26196=ADVANCED_FACE('',(#3383),#2176,.F.);
#26197=ADVANCED_FACE('',(#3384),#2177,.F.);
#26198=ADVANCED_FACE('',(#3385),#2178,.T.);
#26199=ADVANCED_FACE('',(#3386),#2179,.F.);
#26200=ADVANCED_FACE('',(#3387),#2180,.F.);
#26201=ADVANCED_FACE('',(#3388),#2181,.F.);
#26202=ADVANCED_FACE('',(#3389),#2182,.T.);
#26203=ADVANCED_FACE('',(#3390),#2183,.F.);
#26204=ADVANCED_FACE('',(#3391),#2184,.F.);
#26205=ADVANCED_FACE('',(#3392),#2185,.T.);
#26206=ADVANCED_FACE('',(#3393),#2186,.F.);
#26207=ADVANCED_FACE('',(#3394),#2187,.F.);
#26208=ADVANCED_FACE('',(#3395),#2188,.T.);
#26209=ADVANCED_FACE('',(#3396),#2189,.F.);
#26210=ADVANCED_FACE('',(#3397),#2190,.F.);
#26211=ADVANCED_FACE('',(#3398),#2191,.F.);
#26212=ADVANCED_FACE('',(#3399),#2192,.T.);
#26213=ADVANCED_FACE('',(#3400),#2193,.T.);
#26214=ADVANCED_FACE('',(#3401),#2194,.T.);
#26215=ADVANCED_FACE('',(#3402),#2195,.T.);
#26216=ADVANCED_FACE('',(#3403),#2196,.T.);
#26217=ADVANCED_FACE('',(#3404),#2197,.T.);
#26218=ADVANCED_FACE('',(#3405),#2198,.T.);
#26219=ADVANCED_FACE('',(#3406),#2199,.T.);
#26220=ADVANCED_FACE('',(#3407),#2200,.T.);
#26221=ADVANCED_FACE('',(#3408),#2201,.T.);
#26222=ADVANCED_FACE('',(#3409),#2202,.T.);
#26223=ADVANCED_FACE('',(#3410),#2203,.T.);
#26224=ADVANCED_FACE('',(#3411),#2204,.T.);
#26225=ADVANCED_FACE('',(#3412),#2205,.T.);
#26226=ADVANCED_FACE('',(#3413),#2206,.T.);
#26227=ADVANCED_FACE('',(#3414),#2207,.T.);
#26228=ADVANCED_FACE('',(#3415),#2208,.T.);
#26229=ADVANCED_FACE('',(#3416),#2209,.T.);
#26230=ADVANCED_FACE('',(#3417),#2210,.T.);
#26231=ADVANCED_FACE('',(#3418),#2211,.T.);
#26232=ADVANCED_FACE('',(#3419),#2212,.T.);
#26233=ADVANCED_FACE('',(#3420),#2213,.T.);
#26234=ADVANCED_FACE('',(#3421),#2214,.T.);
#26235=ADVANCED_FACE('',(#3422),#2215,.T.);
#26236=ADVANCED_FACE('',(#3423),#2216,.T.);
#26237=ADVANCED_FACE('',(#3424),#2217,.T.);
#26238=ADVANCED_FACE('',(#3425),#2218,.T.);
#26239=ADVANCED_FACE('',(#3426),#2219,.T.);
#26240=ADVANCED_FACE('',(#3427),#2220,.T.);
#26241=ADVANCED_FACE('',(#3428),#2221,.T.);
#26242=ADVANCED_FACE('',(#3429),#2222,.T.);
#26243=ADVANCED_FACE('',(#3430),#2223,.T.);
#26244=ADVANCED_FACE('',(#3431),#2224,.T.);
#26245=ADVANCED_FACE('',(#3432),#2225,.T.);
#26246=ADVANCED_FACE('',(#3433),#2226,.T.);
#26247=ADVANCED_FACE('',(#3434),#2227,.T.);
#26248=ADVANCED_FACE('',(#3435),#2228,.T.);
#26249=ADVANCED_FACE('',(#3436),#2229,.T.);
#26250=ADVANCED_FACE('',(#3437),#2230,.F.);
#26251=ADVANCED_FACE('',(#3438),#2231,.T.);
#26252=ADVANCED_FACE('',(#3439),#2232,.T.);
#26253=ADVANCED_FACE('',(#3440),#2233,.F.);
#26254=ADVANCED_FACE('',(#3441),#2234,.F.);
#26255=ADVANCED_FACE('',(#3442),#2235,.T.);
#26256=ADVANCED_FACE('',(#3443),#2236,.F.);
#26257=ADVANCED_FACE('',(#3444),#2237,.F.);
#26258=ADVANCED_FACE('',(#3445),#2238,.F.);
#26259=ADVANCED_FACE('',(#3446),#2239,.T.);
#26260=ADVANCED_FACE('',(#3447),#2240,.F.);
#26261=ADVANCED_FACE('',(#3448),#2241,.F.);
#26262=ADVANCED_FACE('',(#3449),#2242,.F.);
#26263=ADVANCED_FACE('',(#3450),#2243,.T.);
#26264=ADVANCED_FACE('',(#3451),#2244,.F.);
#26265=ADVANCED_FACE('',(#3452),#2245,.F.);
#26266=ADVANCED_FACE('',(#3453),#2246,.F.);
#26267=ADVANCED_FACE('',(#3454),#2247,.T.);
#26268=ADVANCED_FACE('',(#3455),#2248,.F.);
#26269=ADVANCED_FACE('',(#3456),#2249,.F.);
#26270=ADVANCED_FACE('',(#3457),#2250,.F.);
#26271=ADVANCED_FACE('',(#3458),#2251,.T.);
#26272=ADVANCED_FACE('',(#3459),#2252,.F.);
#26273=ADVANCED_FACE('',(#3460),#2253,.F.);
#26274=ADVANCED_FACE('',(#3461),#2254,.F.);
#26275=ADVANCED_FACE('',(#3462),#2255,.T.);
#26276=ADVANCED_FACE('',(#3463),#2256,.F.);
#26277=ADVANCED_FACE('',(#3464),#2257,.F.);
#26278=ADVANCED_FACE('',(#3465),#2258,.T.);
#26279=ADVANCED_FACE('',(#3466),#2259,.T.);
#26280=ADVANCED_FACE('',(#3467),#2260,.T.);
#26281=ADVANCED_FACE('',(#3468),#2261,.T.);
#26282=ADVANCED_FACE('',(#3469,#876),#2262,.T.);
#26283=ADVANCED_FACE('',(#3470),#2263,.T.);
#26284=ADVANCED_FACE('',(#3471),#2264,.T.);
#26285=ADVANCED_FACE('',(#3472),#2265,.T.);
#26286=ADVANCED_FACE('',(#3473),#2266,.T.);
#26287=ADVANCED_FACE('',(#3474),#2267,.T.);
#26288=ADVANCED_FACE('',(#3475),#2268,.T.);
#26289=ADVANCED_FACE('',(#3476),#2269,.T.);
#26290=ADVANCED_FACE('',(#3477),#2270,.T.);
#26291=ADVANCED_FACE('',(#3478),#2271,.T.);
#26292=ADVANCED_FACE('',(#3479),#2272,.T.);
#26293=ADVANCED_FACE('',(#3480),#2273,.T.);
#26294=ADVANCED_FACE('',(#3481),#2274,.T.);
#26295=ADVANCED_FACE('',(#3482),#2275,.T.);
#26296=ADVANCED_FACE('',(#3483),#2276,.T.);
#26297=ADVANCED_FACE('',(#3484),#2277,.T.);
#26298=ADVANCED_FACE('',(#3485),#2278,.T.);
#26299=ADVANCED_FACE('',(#3486),#2279,.T.);
#26300=ADVANCED_FACE('',(#3487),#2280,.T.);
#26301=ADVANCED_FACE('',(#3488),#2281,.T.);
#26302=ADVANCED_FACE('',(#3489),#2282,.T.);
#26303=ADVANCED_FACE('',(#3490),#2283,.T.);
#26304=ADVANCED_FACE('',(#3491),#2284,.T.);
#26305=ADVANCED_FACE('',(#3492),#2285,.T.);
#26306=ADVANCED_FACE('',(#3493),#2286,.T.);
#26307=ADVANCED_FACE('',(#3494),#2287,.T.);
#26308=ADVANCED_FACE('',(#3495),#2288,.T.);
#26309=ADVANCED_FACE('',(#3496),#2289,.T.);
#26310=ADVANCED_FACE('',(#3497),#2290,.T.);
#26311=ADVANCED_FACE('',(#3498),#2291,.T.);
#26312=ADVANCED_FACE('',(#3499),#2292,.T.);
#26313=ADVANCED_FACE('',(#3500),#2293,.T.);
#26314=ADVANCED_FACE('',(#3501),#2294,.T.);
#26315=ADVANCED_FACE('',(#3502),#2295,.T.);
#26316=ADVANCED_FACE('',(#3503),#2296,.T.);
#26317=ADVANCED_FACE('',(#3504),#2297,.T.);
#26318=ADVANCED_FACE('',(#3505),#2298,.T.);
#26319=ADVANCED_FACE('',(#3506),#2299,.T.);
#26320=ADVANCED_FACE('',(#3507),#2300,.T.);
#26321=ADVANCED_FACE('',(#3508),#2301,.T.);
#26322=ADVANCED_FACE('',(#3509),#2302,.T.);
#26323=ADVANCED_FACE('',(#3510),#2303,.T.);
#26324=ADVANCED_FACE('',(#3511),#2304,.T.);
#26325=ADVANCED_FACE('',(#3512),#2305,.T.);
#26326=ADVANCED_FACE('',(#3513),#2306,.T.);
#26327=ADVANCED_FACE('',(#3514),#2307,.T.);
#26328=ADVANCED_FACE('',(#3515),#2308,.T.);
#26329=ADVANCED_FACE('',(#3516),#2309,.T.);
#26330=ADVANCED_FACE('',(#3517),#2310,.T.);
#26331=ADVANCED_FACE('',(#3518),#2311,.T.);
#26332=ADVANCED_FACE('',(#3519),#2312,.T.);
#26333=ADVANCED_FACE('',(#3520),#2313,.T.);
#26334=ADVANCED_FACE('',(#3521),#2314,.T.);
#26335=ADVANCED_FACE('',(#3522),#2315,.T.);
#26336=ADVANCED_FACE('',(#3523),#2316,.T.);
#26337=ADVANCED_FACE('',(#3524),#2317,.T.);
#26338=ADVANCED_FACE('',(#3525),#2318,.T.);
#26339=ADVANCED_FACE('',(#3526),#2319,.T.);
#26340=ADVANCED_FACE('',(#3527),#2320,.T.);
#26341=ADVANCED_FACE('',(#3528),#2321,.T.);
#26342=ADVANCED_FACE('',(#3529),#2322,.T.);
#26343=ADVANCED_FACE('',(#3530),#2323,.T.);
#26344=ADVANCED_FACE('',(#3531),#2324,.T.);
#26345=ADVANCED_FACE('',(#3532),#2325,.T.);
#26346=ADVANCED_FACE('',(#3533),#2326,.T.);
#26347=ADVANCED_FACE('',(#3534),#2327,.T.);
#26348=ADVANCED_FACE('',(#3535),#2328,.T.);
#26349=ADVANCED_FACE('',(#3536),#2329,.T.);
#26350=ADVANCED_FACE('',(#3537),#2330,.T.);
#26351=ADVANCED_FACE('',(#3538),#2331,.T.);
#26352=ADVANCED_FACE('',(#3539),#2332,.T.);
#26353=ADVANCED_FACE('',(#3540),#2333,.T.);
#26354=ADVANCED_FACE('',(#3541),#2334,.T.);
#26355=ADVANCED_FACE('',(#3542),#2335,.T.);
#26356=ADVANCED_FACE('',(#3543),#2336,.T.);
#26357=ADVANCED_FACE('',(#3544),#2337,.T.);
#26358=ADVANCED_FACE('',(#3545),#2338,.T.);
#26359=ADVANCED_FACE('',(#3546),#2339,.T.);
#26360=ADVANCED_FACE('',(#3547),#2340,.T.);
#26361=ADVANCED_FACE('',(#3548),#2341,.T.);
#26362=ADVANCED_FACE('',(#3549),#2342,.T.);
#26363=ADVANCED_FACE('',(#3550),#2343,.T.);
#26364=ADVANCED_FACE('',(#3551),#2344,.T.);
#26365=ADVANCED_FACE('',(#3552),#2345,.T.);
#26366=ADVANCED_FACE('',(#3553),#2346,.T.);
#26367=ADVANCED_FACE('',(#3554),#2347,.T.);
#26368=ADVANCED_FACE('',(#3555),#2348,.T.);
#26369=ADVANCED_FACE('',(#3556),#2349,.T.);
#26370=ADVANCED_FACE('',(#3557),#2350,.T.);
#26371=ADVANCED_FACE('',(#3558),#2351,.T.);
#26372=ADVANCED_FACE('',(#3559),#2352,.T.);
#26373=ADVANCED_FACE('',(#3560),#2353,.T.);
#26374=ADVANCED_FACE('',(#3561),#2354,.T.);
#26375=ADVANCED_FACE('',(#3562),#2355,.T.);
#26376=ADVANCED_FACE('',(#3563),#2356,.T.);
#26377=ADVANCED_FACE('',(#3564),#2357,.T.);
#26378=ADVANCED_FACE('',(#3565),#2358,.T.);
#26379=ADVANCED_FACE('',(#3566),#2359,.T.);
#26380=ADVANCED_FACE('',(#3567),#2360,.T.);
#26381=ADVANCED_FACE('',(#3568),#2361,.T.);
#26382=ADVANCED_FACE('',(#3569),#2362,.T.);
#26383=ADVANCED_FACE('',(#3570),#2363,.T.);
#26384=ADVANCED_FACE('',(#3571),#2364,.T.);
#26385=ADVANCED_FACE('',(#3572),#2365,.T.);
#26386=ADVANCED_FACE('',(#3573),#2366,.T.);
#26387=ADVANCED_FACE('',(#3574),#2367,.T.);
#26388=ADVANCED_FACE('',(#3575),#2368,.T.);
#26389=ADVANCED_FACE('',(#3576),#2369,.T.);
#26390=ADVANCED_FACE('',(#3577),#2370,.T.);
#26391=ADVANCED_FACE('',(#3578),#2371,.T.);
#26392=ADVANCED_FACE('',(#3579),#2372,.T.);
#26393=ADVANCED_FACE('',(#3580),#286,.T.);
#26394=ADVANCED_FACE('',(#3581),#728,.F.);
#26395=ADVANCED_FACE('',(#3582,#877),#729,.F.);
#26396=ADVANCED_FACE('',(#3583),#25344,.F.);
#26397=ADVANCED_FACE('',(#3584),#25345,.F.);
#26398=ADVANCED_FACE('',(#3585),#25346,.F.);
#26399=ADVANCED_FACE('',(#3586),#2373,.T.);
#26400=ADVANCED_FACE('',(#3587),#2374,.T.);
#26401=ADVANCED_FACE('',(#3588),#2375,.T.);
#26402=ADVANCED_FACE('',(#3589),#2376,.T.);
#26403=ADVANCED_FACE('',(#3590),#2377,.T.);
#26404=ADVANCED_FACE('',(#3591),#2378,.T.);
#26405=ADVANCED_FACE('',(#3592),#2379,.T.);
#26406=ADVANCED_FACE('',(#3593),#2380,.T.);
#26407=ADVANCED_FACE('',(#3594),#2381,.T.);
#26408=ADVANCED_FACE('',(#3595),#2382,.T.);
#26409=ADVANCED_FACE('',(#3596),#2383,.T.);
#26410=ADVANCED_FACE('',(#3597),#2384,.T.);
#26411=ADVANCED_FACE('',(#3598),#2385,.T.);
#26412=ADVANCED_FACE('',(#3599),#2386,.T.);
#26413=ADVANCED_FACE('',(#3600),#2387,.T.);
#26414=ADVANCED_FACE('',(#3601),#2388,.T.);
#26415=ADVANCED_FACE('',(#3602),#2389,.T.);
#26416=ADVANCED_FACE('',(#3603),#2390,.T.);
#26417=ADVANCED_FACE('',(#3604),#2391,.T.);
#26883=CLOSED_SHELL('',(#25936,#25937,#25938,#25939,#25940,#25941,#25942,
#25943,#25944,#25945,#25946,#25947,#25948,#25949,#25950,#25951,#25952,#25953,
#25954,#25955,#25956,#25957,#25958,#25959,#25960,#25961,#25962,#25963,#25964,
#25965,#25966,#25967,#25968,#25969,#25970,#25971,#25972,#25973,#25974,#25975,
#25976,#25977,#25978,#25979,#25980,#25981,#25982,#25983,#25984,#25985,#25986,
#25987,#25988,#25989,#25990,#25991,#25992,#25993,#25994,#25995,#25996,#25997,
#25998,#25999,#26000,#26001,#26002,#26003,#26004,#26005,#26006,#26007,#26008,
#26009,#26010,#26011,#26012,#26013,#26014,#26015,#26016,#26017,#26018,#26019,
#26020,#26021,#26022,#26023,#26024,#26025,#26026,#26027,#26028,#26029,#26030,
#26031,#26032,#26033,#26034,#26035,#26036,#26037,#26038,#26039,#26040,#26041,
#26042,#26043,#26044,#26045,#26046,#26047,#26048,#26049,#26050,#26051,#26052,
#26053,#26054,#26055,#26056,#26057,#26058,#26059,#26060,#26061,#26062,#26063,
#26064,#26065,#26066,#26067,#26068,#26069,#26070,#26071,#26072,#26073,#26074,
#26075,#26076,#26077,#26078,#26079,#26080,#26081,#26082,#26083,#26084,#26085,
#26086,#26087,#26088,#26089,#26090,#26091,#26092,#26093,#26094,#26095,#26096,
#26097,#26098,#26099,#26100,#26101,#26102,#26103,#26104,#26105,#26106,#26107,
#26108,#26109,#26110,#26111,#26112,#26113,#26114,#26115,#26116,#26117,#26118,
#26119,#26120,#26121,#26122,#26123,#26124,#26125,#26126,#26127,#26128,#26129,
#26130,#26131,#26132,#26133,#26134,#26135,#26136,#26137,#26138,#26139,#26140,
#26141,#26142,#26143,#26144,#26145,#26146,#26147,#26148,#26149,#26150,#26151,
#26152,#26153,#26154,#26155,#26156,#26157,#26158,#26159,#26160,#26161,#26162,
#26163,#26164,#26165,#26166,#26167,#26168,#26169,#26170,#26171,#26172,#26173,
#26174,#26175,#26176,#26177,#26178,#26179,#26180,#26181,#26182,#26183,#26184,
#26185,#26186,#26187,#26188,#26189,#26190,#26191,#26192,#26193,#26194,#26195,
#26196,#26197,#26198,#26199,#26200,#26201,#26202,#26203,#26204,#26205,#26206,
#26207,#26208,#26209,#26210,#26211,#26212,#26213,#26214,#26215,#26216,#26217,
#26218,#26219,#26220,#26221,#26222,#26223,#26224,#26225,#26226,#26227,#26228,
#26229,#26230,#26231,#26232,#26233,#26234,#26235,#26236,#26237,#26238,#26239,
#26240,#26241,#26242,#26243,#26244,#26245,#26246,#26247,#26248,#26249,#26250,
#26251,#26252,#26253,#26254,#26255,#26256,#26257,#26258,#26259,#26260,#26261,
#26262,#26263,#26264,#26265,#26266,#26267,#26268,#26269,#26270,#26271,#26272,
#26273,#26274,#26275,#26276,#26277,#26278,#26279,#26280,#26281,#26282,#26283,
#26284,#26285,#26286,#26287,#26288,#26289,#26290,#26291,#26292,#26293,#26294,
#26295,#26296,#26297,#26298,#26299,#26300,#26301,#26302,#26303,#26304,#26305,
#26306,#26307,#26308,#26309,#26310,#26311,#26312,#26313,#26314,#26315,#26316,
#26317,#26318,#26319,#26320,#26321,#26322,#26323,#26324,#26325,#26326,#26327,
#26328,#26329,#26330,#26331,#26332,#26333,#26334,#26335,#26336,#26337,#26338,
#26339,#26340,#26341,#26342,#26343,#26344,#26345,#26346,#26347,#26348,#26349,
#26350,#26351,#26352,#26353,#26354,#26355,#26356,#26357,#26358,#26359,#26360,
#26361,#26362,#26363,#26364,#26365,#26366,#26367,#26368,#26369,#26370,#26371,
#26372,#26373,#26374,#26375,#26376,#26377,#26378,#26379,#26380,#26381,#26382,
#26383,#26384,#26385,#26386,#26387,#26388,#26389,#26390,#26391,#26392,#26393,
#26394,#26395,#26396,#26397,#26398,#26399,#26400,#26401,#26402,#26403,#26404,
#26405,#26406,#26407,#26408,#26409,#26410,#26411,#26412,#26413,#26414,#26415,
#26416,#26417));
#27818=AXIS2_PLACEMENT_3D('',#60846,#31134,#31135);
#27819=AXIS2_PLACEMENT_3D('',#60847,#31136,#31137);
#27820=AXIS2_PLACEMENT_3D('',#60860,#31144,#31145);
#27821=AXIS2_PLACEMENT_3D('',#60868,#31150,#31151);
#27822=AXIS2_PLACEMENT_3D('',#60872,#31154,#31155);
#27823=AXIS2_PLACEMENT_3D('',#60878,#31159,#31160);
#27824=AXIS2_PLACEMENT_3D('',#60891,#31167,#31168);
#27825=AXIS2_PLACEMENT_3D('',#60899,#31173,#31174);
#27826=AXIS2_PLACEMENT_3D('',#60903,#31177,#31178);
#27827=AXIS2_PLACEMENT_3D('',#60909,#31182,#31183);
#27828=AXIS2_PLACEMENT_3D('',#60922,#31190,#31191);
#27829=AXIS2_PLACEMENT_3D('',#60928,#31195,#31196);
#27830=AXIS2_PLACEMENT_3D('',#60934,#31200,#31201);
#27831=AXIS2_PLACEMENT_3D('',#60942,#31206,#31207);
#27832=AXIS2_PLACEMENT_3D('',#60955,#31214,#31215);
#27833=AXIS2_PLACEMENT_3D('',#60963,#31220,#31221);
#27834=AXIS2_PLACEMENT_3D('',#60967,#31224,#31225);
#27835=AXIS2_PLACEMENT_3D('',#60973,#31229,#31230);
#27836=AXIS2_PLACEMENT_3D('',#60986,#31237,#31238);
#27837=AXIS2_PLACEMENT_3D('',#60992,#31242,#31243);
#27838=AXIS2_PLACEMENT_3D('',#61000,#31248,#31249);
#27839=AXIS2_PLACEMENT_3D('',#61006,#31253,#31254);
#27840=AXIS2_PLACEMENT_3D('',#61019,#31261,#31262);
#27841=AXIS2_PLACEMENT_3D('',#61027,#31267,#31268);
#27842=AXIS2_PLACEMENT_3D('',#61035,#31273,#31274);
#27843=AXIS2_PLACEMENT_3D('',#61039,#31277,#31278);
#27844=AXIS2_PLACEMENT_3D('',#61047,#31283,#31284);
#27845=AXIS2_PLACEMENT_3D('',#61053,#31288,#31289);
#27846=AXIS2_PLACEMENT_3D('',#61066,#31296,#31297);
#27847=AXIS2_PLACEMENT_3D('',#61072,#31301,#31302);
#27848=AXIS2_PLACEMENT_3D('',#61078,#31306,#31307);
#27849=AXIS2_PLACEMENT_3D('',#61081,#31310,#31311);
#27850=AXIS2_PLACEMENT_3D('',#61094,#31318,#31319);
#27851=AXIS2_PLACEMENT_3D('',#61100,#31323,#31324);
#27852=AXIS2_PLACEMENT_3D('',#61108,#31329,#31330);
#27853=AXIS2_PLACEMENT_3D('',#61114,#31334,#31335);
#27854=AXIS2_PLACEMENT_3D('',#61127,#31342,#31343);
#27855=AXIS2_PLACEMENT_3D('',#61135,#31348,#31349);
#27856=AXIS2_PLACEMENT_3D('',#61143,#31354,#31355);
#27857=AXIS2_PLACEMENT_3D('',#61147,#31358,#31359);
#27858=AXIS2_PLACEMENT_3D('',#61155,#31364,#31365);
#27859=AXIS2_PLACEMENT_3D('',#61161,#31369,#31370);
#27860=AXIS2_PLACEMENT_3D('',#61174,#31377,#31378);
#27861=AXIS2_PLACEMENT_3D('',#61180,#31382,#31383);
#27862=AXIS2_PLACEMENT_3D('',#61186,#31387,#31388);
#27863=AXIS2_PLACEMENT_3D('',#61189,#31391,#31392);
#27864=AXIS2_PLACEMENT_3D('',#61202,#31399,#31400);
#27865=AXIS2_PLACEMENT_3D('',#61210,#31405,#31406);
#27866=AXIS2_PLACEMENT_3D('',#61218,#31411,#31412);
#27867=AXIS2_PLACEMENT_3D('',#61222,#31415,#31416);
#27868=AXIS2_PLACEMENT_3D('',#61230,#31421,#31422);
#27869=AXIS2_PLACEMENT_3D('',#61236,#31426,#31427);
#27870=AXIS2_PLACEMENT_3D('',#61249,#31434,#31435);
#27871=AXIS2_PLACEMENT_3D('',#61255,#31439,#31440);
#27872=AXIS2_PLACEMENT_3D('',#61261,#31444,#31445);
#27873=AXIS2_PLACEMENT_3D('',#61269,#31450,#31451);
#27874=AXIS2_PLACEMENT_3D('',#61279,#31457,#31458);
#27875=AXIS2_PLACEMENT_3D('',#61285,#31462,#31463);
#27876=AXIS2_PLACEMENT_3D('',#61291,#31467,#31468);
#27877=AXIS2_PLACEMENT_3D('',#61296,#31472,#31473);
#27878=AXIS2_PLACEMENT_3D('',#61309,#31480,#31481);
#27879=AXIS2_PLACEMENT_3D('',#61317,#31486,#31487);
#27880=AXIS2_PLACEMENT_3D('',#61325,#31492,#31493);
#27881=AXIS2_PLACEMENT_3D('',#61329,#31496,#31497);
#27882=AXIS2_PLACEMENT_3D('',#61337,#31502,#31503);
#27883=AXIS2_PLACEMENT_3D('',#61343,#31507,#31508);
#27884=AXIS2_PLACEMENT_3D('',#61356,#31515,#31516);
#27885=AXIS2_PLACEMENT_3D('',#61364,#31521,#31522);
#27886=AXIS2_PLACEMENT_3D('',#61372,#31527,#31528);
#27887=AXIS2_PLACEMENT_3D('',#61376,#31531,#31532);
#27888=AXIS2_PLACEMENT_3D('',#61384,#31537,#31538);
#27889=AXIS2_PLACEMENT_3D('',#61390,#31542,#31543);
#27890=AXIS2_PLACEMENT_3D('',#61403,#31550,#31551);
#27891=AXIS2_PLACEMENT_3D('',#61411,#31556,#31557);
#27892=AXIS2_PLACEMENT_3D('',#61415,#31560,#31561);
#27893=AXIS2_PLACEMENT_3D('',#61421,#31565,#31566);
#27894=AXIS2_PLACEMENT_3D('',#61434,#31573,#31574);
#27895=AXIS2_PLACEMENT_3D('',#61442,#31579,#31580);
#27896=AXIS2_PLACEMENT_3D('',#61450,#31585,#31586);
#27897=AXIS2_PLACEMENT_3D('',#61454,#31589,#31590);
#27898=AXIS2_PLACEMENT_3D('',#61462,#31595,#31596);
#27899=AXIS2_PLACEMENT_3D('',#61468,#31600,#31601);
#27900=AXIS2_PLACEMENT_3D('',#61481,#31608,#31609);
#27901=AXIS2_PLACEMENT_3D('',#61489,#31614,#31615);
#27902=AXIS2_PLACEMENT_3D('',#61497,#31620,#31621);
#27903=AXIS2_PLACEMENT_3D('',#61501,#31624,#31625);
#27904=AXIS2_PLACEMENT_3D('',#61509,#31630,#31631);
#27905=AXIS2_PLACEMENT_3D('',#61515,#31635,#31636);
#27906=AXIS2_PLACEMENT_3D('',#61525,#31642,#31643);
#27907=AXIS2_PLACEMENT_3D('',#61531,#31647,#31648);
#27908=AXIS2_PLACEMENT_3D('',#61535,#31651,#31652);
#27909=AXIS2_PLACEMENT_3D('',#61541,#31656,#31657);
#27910=AXIS2_PLACEMENT_3D('',#61550,#31662,#31663);
#27911=AXIS2_PLACEMENT_3D('',#61557,#31667,#31668);
#27912=AXIS2_PLACEMENT_3D('',#61558,#31669,#31670);
#27913=AXIS2_PLACEMENT_3D('',#61566,#31675,#31676);
#27914=AXIS2_PLACEMENT_3D('',#61578,#31683,#31684);
#27915=AXIS2_PLACEMENT_3D('',#61582,#31687,#31688);
#27916=AXIS2_PLACEMENT_3D('',#61592,#31694,#31695);
#27917=AXIS2_PLACEMENT_3D('',#61600,#31700,#31701);
#27918=AXIS2_PLACEMENT_3D('',#61602,#31703,#31704);
#27919=AXIS2_PLACEMENT_3D('',#61615,#31711,#31712);
#27920=AXIS2_PLACEMENT_3D('',#61622,#31717,#31718);
#27921=AXIS2_PLACEMENT_3D('',#61630,#31723,#31724);
#27922=AXIS2_PLACEMENT_3D('',#61634,#31727,#31728);
#27923=AXIS2_PLACEMENT_3D('',#61647,#31735,#31736);
#27924=AXIS2_PLACEMENT_3D('',#61655,#31741,#31742);
#27925=AXIS2_PLACEMENT_3D('',#61663,#31747,#31748);
#27926=AXIS2_PLACEMENT_3D('',#61667,#31751,#31752);
#27927=AXIS2_PLACEMENT_3D('',#61675,#31757,#31758);
#27928=AXIS2_PLACEMENT_3D('',#61681,#31762,#31763);
#27929=AXIS2_PLACEMENT_3D('',#61694,#31770,#31771);
#27930=AXIS2_PLACEMENT_3D('',#61702,#31776,#31777);
#27931=AXIS2_PLACEMENT_3D('',#61710,#31782,#31783);
#27932=AXIS2_PLACEMENT_3D('',#61714,#31786,#31787);
#27933=AXIS2_PLACEMENT_3D('',#61722,#31792,#31793);
#27934=AXIS2_PLACEMENT_3D('',#61728,#31797,#31798);
#27935=AXIS2_PLACEMENT_3D('',#61741,#31805,#31806);
#27936=AXIS2_PLACEMENT_3D('',#61749,#31811,#31812);
#27937=AXIS2_PLACEMENT_3D('',#61757,#31817,#31818);
#27938=AXIS2_PLACEMENT_3D('',#61761,#31821,#31822);
#27939=AXIS2_PLACEMENT_3D('',#61769,#31827,#31828);
#27940=AXIS2_PLACEMENT_3D('',#61775,#31832,#31833);
#27941=AXIS2_PLACEMENT_3D('',#61788,#31840,#31841);
#27942=AXIS2_PLACEMENT_3D('',#61796,#31846,#31847);
#27943=AXIS2_PLACEMENT_3D('',#61804,#31852,#31853);
#27944=AXIS2_PLACEMENT_3D('',#61808,#31856,#31857);
#27945=AXIS2_PLACEMENT_3D('',#61816,#31862,#31863);
#27946=AXIS2_PLACEMENT_3D('',#61822,#31867,#31868);
#27947=AXIS2_PLACEMENT_3D('',#61835,#31875,#31876);
#27948=AXIS2_PLACEMENT_3D('',#61841,#31880,#31881);
#27949=AXIS2_PLACEMENT_3D('',#61847,#31885,#31886);
#27950=AXIS2_PLACEMENT_3D('',#61850,#31889,#31890);
#27951=AXIS2_PLACEMENT_3D('',#61853,#31893,#31894);
#27952=AXIS2_PLACEMENT_3D('',#61857,#31897,#31898);
#27953=AXIS2_PLACEMENT_3D('',#61859,#31900,#31901);
#27954=AXIS2_PLACEMENT_3D('',#61862,#31904,#31905);
#27955=AXIS2_PLACEMENT_3D('',#61866,#31908,#31909);
#27956=AXIS2_PLACEMENT_3D('',#61870,#31912,#31913);
#27957=AXIS2_PLACEMENT_3D('',#61872,#31915,#31916);
#27958=AXIS2_PLACEMENT_3D('',#61875,#31919,#31920);
#27959=AXIS2_PLACEMENT_3D('',#61879,#31923,#31924);
#27960=AXIS2_PLACEMENT_3D('',#61881,#31926,#31927);
#27961=AXIS2_PLACEMENT_3D('',#62015,#32003,#32004);
#27962=AXIS2_PLACEMENT_3D('',#62017,#32006,#32007);
#27963=AXIS2_PLACEMENT_3D('',#62021,#32010,#32011);
#27964=AXIS2_PLACEMENT_3D('',#62023,#32013,#32014);
#27965=AXIS2_PLACEMENT_3D('',#62025,#32016,#32017);
#27966=AXIS2_PLACEMENT_3D('',#62029,#32020,#32021);
#27967=AXIS2_PLACEMENT_3D('',#62033,#32024,#32025);
#27968=AXIS2_PLACEMENT_3D('',#62035,#32027,#32028);
#27969=AXIS2_PLACEMENT_3D('',#62037,#32030,#32031);
#27970=AXIS2_PLACEMENT_3D('',#62041,#32034,#32035);
#27971=AXIS2_PLACEMENT_3D('',#62045,#32038,#32039);
#27972=AXIS2_PLACEMENT_3D('',#62047,#32041,#32042);
#27973=AXIS2_PLACEMENT_3D('',#62049,#32044,#32045);
#27974=AXIS2_PLACEMENT_3D('',#62053,#32048,#32049);
#27975=AXIS2_PLACEMENT_3D('',#62057,#32052,#32053);
#27976=AXIS2_PLACEMENT_3D('',#62059,#32055,#32056);
#27977=AXIS2_PLACEMENT_3D('',#62063,#32059,#32060);
#27978=AXIS2_PLACEMENT_3D('',#62067,#32063,#32064);
#27979=AXIS2_PLACEMENT_3D('',#62071,#32067,#32068);
#27980=AXIS2_PLACEMENT_3D('',#62080,#32073,#32074);
#27981=AXIS2_PLACEMENT_3D('',#62087,#32079,#32080);
#27982=AXIS2_PLACEMENT_3D('',#62090,#32083,#32084);
#27983=AXIS2_PLACEMENT_3D('',#62096,#32088,#32089);
#27984=AXIS2_PLACEMENT_3D('',#62102,#32093,#32094);
#27985=AXIS2_PLACEMENT_3D('',#62107,#32098,#32099);
#27986=AXIS2_PLACEMENT_3D('',#62115,#32104,#32105);
#27987=AXIS2_PLACEMENT_3D('',#62119,#32108,#32109);
#27988=AXIS2_PLACEMENT_3D('',#62132,#32116,#32117);
#27989=AXIS2_PLACEMENT_3D('',#62137,#32121,#32122);
#27990=AXIS2_PLACEMENT_3D('',#62143,#32126,#32127);
#27991=AXIS2_PLACEMENT_3D('',#62147,#32130,#32131);
#27992=AXIS2_PLACEMENT_3D('',#62155,#32136,#32137);
#27993=AXIS2_PLACEMENT_3D('',#62157,#32139,#32140);
#27994=AXIS2_PLACEMENT_3D('',#62159,#32142,#32143);
#27995=AXIS2_PLACEMENT_3D('',#62161,#32145,#32146);
#27996=AXIS2_PLACEMENT_3D('',#62165,#32149,#32150);
#27997=AXIS2_PLACEMENT_3D('',#62169,#32153,#32154);
#27998=AXIS2_PLACEMENT_3D('',#62171,#32156,#32157);
#27999=AXIS2_PLACEMENT_3D('',#62173,#32159,#32160);
#28000=AXIS2_PLACEMENT_3D('',#62177,#32163,#32164);
#28001=AXIS2_PLACEMENT_3D('',#62179,#32166,#32167);
#28002=AXIS2_PLACEMENT_3D('',#62181,#32169,#32170);
#28003=AXIS2_PLACEMENT_3D('',#62185,#32173,#32174);
#28004=AXIS2_PLACEMENT_3D('',#62189,#32177,#32178);
#28005=AXIS2_PLACEMENT_3D('',#62191,#32180,#32181);
#28006=AXIS2_PLACEMENT_3D('',#62193,#32183,#32184);
#28007=AXIS2_PLACEMENT_3D('',#62195,#32186,#32187);
#28008=AXIS2_PLACEMENT_3D('',#62199,#32190,#32191);
#28009=AXIS2_PLACEMENT_3D('',#62201,#32193,#32194);
#28010=AXIS2_PLACEMENT_3D('',#62203,#32196,#32197);
#28011=AXIS2_PLACEMENT_3D('',#62207,#32200,#32201);
#28012=AXIS2_PLACEMENT_3D('',#62209,#32203,#32204);
#28013=AXIS2_PLACEMENT_3D('',#62211,#32206,#32207);
#28014=AXIS2_PLACEMENT_3D('',#62215,#32210,#32211);
#28015=AXIS2_PLACEMENT_3D('',#62217,#32213,#32214);
#28016=AXIS2_PLACEMENT_3D('',#62219,#32216,#32217);
#28017=AXIS2_PLACEMENT_3D('',#62223,#32220,#32221);
#28018=AXIS2_PLACEMENT_3D('',#62225,#32223,#32224);
#28019=AXIS2_PLACEMENT_3D('',#62227,#32226,#32227);
#28020=AXIS2_PLACEMENT_3D('',#62231,#32230,#32231);
#28021=AXIS2_PLACEMENT_3D('',#62235,#32234,#32235);
#28022=AXIS2_PLACEMENT_3D('',#62237,#32237,#32238);
#28023=AXIS2_PLACEMENT_3D('',#62250,#32245,#32246);
#28024=AXIS2_PLACEMENT_3D('',#62255,#32250,#32251);
#28025=AXIS2_PLACEMENT_3D('',#62261,#32255,#32256);
#28026=AXIS2_PLACEMENT_3D('',#62265,#32259,#32260);
#28027=AXIS2_PLACEMENT_3D('',#62273,#32265,#32266);
#28028=AXIS2_PLACEMENT_3D('',#62277,#32269,#32270);
#28029=AXIS2_PLACEMENT_3D('',#62290,#32277,#32278);
#28030=AXIS2_PLACEMENT_3D('',#62295,#32282,#32283);
#28031=AXIS2_PLACEMENT_3D('',#62301,#32287,#32288);
#28032=AXIS2_PLACEMENT_3D('',#62305,#32291,#32292);
#28033=AXIS2_PLACEMENT_3D('',#62313,#32297,#32298);
#28034=AXIS2_PLACEMENT_3D('',#62317,#32301,#32302);
#28035=AXIS2_PLACEMENT_3D('',#62330,#32309,#32310);
#28036=AXIS2_PLACEMENT_3D('',#62335,#32314,#32315);
#28037=AXIS2_PLACEMENT_3D('',#62341,#32319,#32320);
#28038=AXIS2_PLACEMENT_3D('',#62345,#32323,#32324);
#28039=AXIS2_PLACEMENT_3D('',#62353,#32329,#32330);
#28040=AXIS2_PLACEMENT_3D('',#62357,#32333,#32334);
#28041=AXIS2_PLACEMENT_3D('',#62370,#32341,#32342);
#28042=AXIS2_PLACEMENT_3D('',#62376,#32346,#32347);
#28043=AXIS2_PLACEMENT_3D('',#62379,#32350,#32351);
#28044=AXIS2_PLACEMENT_3D('',#62385,#32355,#32356);
#28045=AXIS2_PLACEMENT_3D('',#62395,#32362,#32363);
#28046=AXIS2_PLACEMENT_3D('',#62401,#32367,#32368);
#28047=AXIS2_PLACEMENT_3D('',#62407,#32372,#32373);
#28048=AXIS2_PLACEMENT_3D('',#62412,#32377,#32378);
#28049=AXIS2_PLACEMENT_3D('',#62425,#32385,#32386);
#28050=AXIS2_PLACEMENT_3D('',#62430,#32390,#32391);
#28051=AXIS2_PLACEMENT_3D('',#62436,#32395,#32396);
#28052=AXIS2_PLACEMENT_3D('',#62440,#32399,#32400);
#28053=AXIS2_PLACEMENT_3D('',#62448,#32405,#32406);
#28054=AXIS2_PLACEMENT_3D('',#62452,#32409,#32410);
#28055=AXIS2_PLACEMENT_3D('',#62465,#32417,#32418);
#28056=AXIS2_PLACEMENT_3D('',#62470,#32422,#32423);
#28057=AXIS2_PLACEMENT_3D('',#62476,#32427,#32428);
#28058=AXIS2_PLACEMENT_3D('',#62480,#32431,#32432);
#28059=AXIS2_PLACEMENT_3D('',#62488,#32437,#32438);
#28060=AXIS2_PLACEMENT_3D('',#62492,#32441,#32442);
#28061=AXIS2_PLACEMENT_3D('',#62500,#32447,#32448);
#28062=AXIS2_PLACEMENT_3D('',#62508,#32453,#32454);
#28063=AXIS2_PLACEMENT_3D('',#62512,#32457,#32458);
#28064=AXIS2_PLACEMENT_3D('',#62514,#32460,#32461);
#28065=AXIS2_PLACEMENT_3D('',#62516,#32463,#32464);
#28066=AXIS2_PLACEMENT_3D('',#62520,#32467,#32468);
#28067=AXIS2_PLACEMENT_3D('',#62522,#32470,#32471);
#28068=AXIS2_PLACEMENT_3D('',#62524,#32473,#32474);
#28069=AXIS2_PLACEMENT_3D('',#62528,#32477,#32478);
#28070=AXIS2_PLACEMENT_3D('',#62532,#32481,#32482);
#28071=AXIS2_PLACEMENT_3D('',#62534,#32484,#32485);
#28072=AXIS2_PLACEMENT_3D('',#62536,#32487,#32488);
#28073=AXIS2_PLACEMENT_3D('',#62538,#32490,#32491);
#28074=AXIS2_PLACEMENT_3D('',#62542,#32494,#32495);
#28075=AXIS2_PLACEMENT_3D('',#62544,#32497,#32498);
#28076=AXIS2_PLACEMENT_3D('',#62546,#32500,#32501);
#28077=AXIS2_PLACEMENT_3D('',#62550,#32504,#32505);
#28078=AXIS2_PLACEMENT_3D('',#62552,#32507,#32508);
#28079=AXIS2_PLACEMENT_3D('',#62554,#32510,#32511);
#28080=AXIS2_PLACEMENT_3D('',#62558,#32514,#32515);
#28081=AXIS2_PLACEMENT_3D('',#62562,#32518,#32519);
#28082=AXIS2_PLACEMENT_3D('',#62564,#32521,#32522);
#28083=AXIS2_PLACEMENT_3D('',#62566,#32524,#32525);
#28084=AXIS2_PLACEMENT_3D('',#62570,#32528,#32529);
#28085=AXIS2_PLACEMENT_3D('',#62574,#32532,#32533);
#28086=AXIS2_PLACEMENT_3D('',#62576,#32535,#32536);
#28087=AXIS2_PLACEMENT_3D('',#62578,#32538,#32539);
#28088=AXIS2_PLACEMENT_3D('',#62582,#32542,#32543);
#28089=AXIS2_PLACEMENT_3D('',#62584,#32545,#32546);
#28090=AXIS2_PLACEMENT_3D('',#62586,#32548,#32549);
#28091=AXIS2_PLACEMENT_3D('',#62590,#32552,#32553);
#28092=AXIS2_PLACEMENT_3D('',#62592,#32555,#32556);
#28093=AXIS2_PLACEMENT_3D('',#62594,#32558,#32559);
#28094=AXIS2_PLACEMENT_3D('',#62598,#32562,#32563);
#28095=AXIS2_PLACEMENT_3D('',#62602,#32566,#32567);
#28096=AXIS2_PLACEMENT_3D('',#62604,#32569,#32570);
#28097=AXIS2_PLACEMENT_3D('',#62617,#32577,#32578);
#28098=AXIS2_PLACEMENT_3D('',#62622,#32582,#32583);
#28099=AXIS2_PLACEMENT_3D('',#62628,#32587,#32588);
#28100=AXIS2_PLACEMENT_3D('',#62632,#32591,#32592);
#28101=AXIS2_PLACEMENT_3D('',#62640,#32597,#32598);
#28102=AXIS2_PLACEMENT_3D('',#62644,#32601,#32602);
#28103=AXIS2_PLACEMENT_3D('',#62657,#32609,#32610);
#28104=AXIS2_PLACEMENT_3D('',#62662,#32614,#32615);
#28105=AXIS2_PLACEMENT_3D('',#62668,#32619,#32620);
#28106=AXIS2_PLACEMENT_3D('',#62672,#32623,#32624);
#28107=AXIS2_PLACEMENT_3D('',#62680,#32629,#32630);
#28108=AXIS2_PLACEMENT_3D('',#62684,#32633,#32634);
#28109=AXIS2_PLACEMENT_3D('',#62697,#32641,#32642);
#28110=AXIS2_PLACEMENT_3D('',#62702,#32646,#32647);
#28111=AXIS2_PLACEMENT_3D('',#62708,#32651,#32652);
#28112=AXIS2_PLACEMENT_3D('',#62712,#32655,#32656);
#28113=AXIS2_PLACEMENT_3D('',#62720,#32661,#32662);
#28114=AXIS2_PLACEMENT_3D('',#62724,#32665,#32666);
#28115=AXIS2_PLACEMENT_3D('',#62737,#32673,#32674);
#28116=AXIS2_PLACEMENT_3D('',#62742,#32678,#32679);
#28117=AXIS2_PLACEMENT_3D('',#62748,#32683,#32684);
#28118=AXIS2_PLACEMENT_3D('',#62752,#32687,#32688);
#28119=AXIS2_PLACEMENT_3D('',#62760,#32693,#32694);
#28120=AXIS2_PLACEMENT_3D('',#62764,#32697,#32698);
#28121=AXIS2_PLACEMENT_3D('',#62777,#32705,#32706);
#28122=AXIS2_PLACEMENT_3D('',#62782,#32710,#32711);
#28123=AXIS2_PLACEMENT_3D('',#62788,#32715,#32716);
#28124=AXIS2_PLACEMENT_3D('',#62792,#32719,#32720);
#28125=AXIS2_PLACEMENT_3D('',#62800,#32725,#32726);
#28126=AXIS2_PLACEMENT_3D('',#62804,#32729,#32730);
#28127=AXIS2_PLACEMENT_3D('',#62817,#32737,#32738);
#28128=AXIS2_PLACEMENT_3D('',#62822,#32742,#32743);
#28129=AXIS2_PLACEMENT_3D('',#62828,#32747,#32748);
#28130=AXIS2_PLACEMENT_3D('',#62832,#32751,#32752);
#28131=AXIS2_PLACEMENT_3D('',#62840,#32757,#32758);
#28132=AXIS2_PLACEMENT_3D('',#62844,#32761,#32762);
#28133=AXIS2_PLACEMENT_3D('',#62852,#32767,#32768);
#28134=AXIS2_PLACEMENT_3D('',#62860,#32773,#32774);
#28135=AXIS2_PLACEMENT_3D('',#62864,#32777,#32778);
#28136=AXIS2_PLACEMENT_3D('',#62866,#32780,#32781);
#28137=AXIS2_PLACEMENT_3D('',#62868,#32783,#32784);
#28138=AXIS2_PLACEMENT_3D('',#62872,#32787,#32788);
#28139=AXIS2_PLACEMENT_3D('',#62874,#32790,#32791);
#28140=AXIS2_PLACEMENT_3D('',#62876,#32793,#32794);
#28141=AXIS2_PLACEMENT_3D('',#62880,#32797,#32798);
#28142=AXIS2_PLACEMENT_3D('',#62884,#32801,#32802);
#28143=AXIS2_PLACEMENT_3D('',#62886,#32804,#32805);
#28144=AXIS2_PLACEMENT_3D('',#62888,#32807,#32808);
#28145=AXIS2_PLACEMENT_3D('',#62892,#32811,#32812);
#28146=AXIS2_PLACEMENT_3D('',#62896,#32815,#32816);
#28147=AXIS2_PLACEMENT_3D('',#62898,#32818,#32819);
#28148=AXIS2_PLACEMENT_3D('',#62900,#32821,#32822);
#28149=AXIS2_PLACEMENT_3D('',#62904,#32825,#32826);
#28150=AXIS2_PLACEMENT_3D('',#62908,#32829,#32830);
#28151=AXIS2_PLACEMENT_3D('',#62910,#32832,#32833);
#28152=AXIS2_PLACEMENT_3D('',#62912,#32835,#32836);
#28153=AXIS2_PLACEMENT_3D('',#62916,#32839,#32840);
#28154=AXIS2_PLACEMENT_3D('',#62920,#32843,#32844);
#28155=AXIS2_PLACEMENT_3D('',#62922,#32846,#32847);
#28156=AXIS2_PLACEMENT_3D('',#62924,#32849,#32850);
#28157=AXIS2_PLACEMENT_3D('',#62928,#32853,#32854);
#28158=AXIS2_PLACEMENT_3D('',#62932,#32857,#32858);
#28159=AXIS2_PLACEMENT_3D('',#62934,#32860,#32861);
#28160=AXIS2_PLACEMENT_3D('',#62937,#32864,#32865);
#28161=AXIS2_PLACEMENT_3D('',#62941,#32868,#32869);
#28162=AXIS2_PLACEMENT_3D('',#62943,#32871,#32872);
#28163=AXIS2_PLACEMENT_3D('',#62945,#32874,#32875);
#28164=AXIS2_PLACEMENT_3D('',#62951,#32879,#32880);
#28165=AXIS2_PLACEMENT_3D('',#62955,#32883,#32884);
#28166=AXIS2_PLACEMENT_3D('',#62959,#32887,#32888);
#28167=AXIS2_PLACEMENT_3D('',#63178,#33003,#33004);
#28168=AXIS2_PLACEMENT_3D('',#63179,#33005,#33006);
#28169=AXIS2_PLACEMENT_3D('',#63181,#33008,#33009);
#28170=AXIS2_PLACEMENT_3D('',#63184,#33012,#33013);
#28171=AXIS2_PLACEMENT_3D('',#63186,#33015,#33016);
#28172=AXIS2_PLACEMENT_3D('',#63188,#33018,#33019);
#28173=AXIS2_PLACEMENT_3D('',#63189,#33020,#33021);
#28174=AXIS2_PLACEMENT_3D('',#63192,#33024,#33025);
#28175=AXIS2_PLACEMENT_3D('',#63194,#33027,#33028);
#28176=AXIS2_PLACEMENT_3D('',#63196,#33030,#33031);
#28177=AXIS2_PLACEMENT_3D('',#63197,#33032,#33033);
#28178=AXIS2_PLACEMENT_3D('',#63200,#33036,#33037);
#28179=AXIS2_PLACEMENT_3D('',#63202,#33039,#33040);
#28180=AXIS2_PLACEMENT_3D('',#63204,#33042,#33043);
#28181=AXIS2_PLACEMENT_3D('',#63205,#33044,#33045);
#28182=AXIS2_PLACEMENT_3D('',#63207,#33047,#33048);
#28183=AXIS2_PLACEMENT_3D('',#63209,#33050,#33051);
#28184=AXIS2_PLACEMENT_3D('',#63211,#33053,#33054);
#28185=AXIS2_PLACEMENT_3D('',#63214,#33057,#33058);
#28186=AXIS2_PLACEMENT_3D('',#63216,#33060,#33061);
#28187=AXIS2_PLACEMENT_3D('',#63218,#33063,#33064);
#28188=AXIS2_PLACEMENT_3D('',#63219,#33065,#33066);
#28189=AXIS2_PLACEMENT_3D('',#63222,#33069,#33070);
#28190=AXIS2_PLACEMENT_3D('',#63223,#33071,#33072);
#28191=AXIS2_PLACEMENT_3D('',#63225,#33074,#33075);
#28192=AXIS2_PLACEMENT_3D('',#63227,#33077,#33078);
#28193=AXIS2_PLACEMENT_3D('',#63230,#33081,#33082);
#28194=AXIS2_PLACEMENT_3D('',#63232,#33084,#33085);
#28195=AXIS2_PLACEMENT_3D('',#63234,#33087,#33088);
#28196=AXIS2_PLACEMENT_3D('',#63235,#33089,#33090);
#28197=AXIS2_PLACEMENT_3D('',#63238,#33093,#33094);
#28198=AXIS2_PLACEMENT_3D('',#63240,#33096,#33097);
#28199=AXIS2_PLACEMENT_3D('',#63242,#33099,#33100);
#28200=AXIS2_PLACEMENT_3D('',#63243,#33101,#33102);
#28201=AXIS2_PLACEMENT_3D('',#63246,#33105,#33106);
#28202=AXIS2_PLACEMENT_3D('',#63248,#33108,#33109);
#28203=AXIS2_PLACEMENT_3D('',#63250,#33111,#33112);
#28204=AXIS2_PLACEMENT_3D('',#63251,#33113,#33114);
#28205=AXIS2_PLACEMENT_3D('',#63254,#33117,#33118);
#28206=AXIS2_PLACEMENT_3D('',#63256,#33120,#33121);
#28207=AXIS2_PLACEMENT_3D('',#63258,#33123,#33124);
#28208=AXIS2_PLACEMENT_3D('',#63259,#33125,#33126);
#28209=AXIS2_PLACEMENT_3D('',#63262,#33129,#33130);
#28210=AXIS2_PLACEMENT_3D('',#63264,#33132,#33133);
#28211=AXIS2_PLACEMENT_3D('',#63266,#33135,#33136);
#28212=AXIS2_PLACEMENT_3D('',#63267,#33137,#33138);
#28213=AXIS2_PLACEMENT_3D('',#63270,#33141,#33142);
#28214=AXIS2_PLACEMENT_3D('',#63271,#33143,#33144);
#28215=AXIS2_PLACEMENT_3D('',#63272,#33145,#33146);
#28216=AXIS2_PLACEMENT_3D('',#63275,#33149,#33150);
#28217=AXIS2_PLACEMENT_3D('',#63277,#33152,#33153);
#28218=AXIS2_PLACEMENT_3D('',#63279,#33155,#33156);
#28219=AXIS2_PLACEMENT_3D('',#63280,#33157,#33158);
#28220=AXIS2_PLACEMENT_3D('',#63283,#33161,#33162);
#28221=AXIS2_PLACEMENT_3D('',#63285,#33164,#33165);
#28222=AXIS2_PLACEMENT_3D('',#63287,#33167,#33168);
#28223=AXIS2_PLACEMENT_3D('',#63288,#33169,#33170);
#28224=AXIS2_PLACEMENT_3D('',#63290,#33172,#33173);
#28225=AXIS2_PLACEMENT_3D('',#63292,#33175,#33176);
#28226=AXIS2_PLACEMENT_3D('',#63294,#33178,#33179);
#28227=AXIS2_PLACEMENT_3D('',#63297,#33182,#33183);
#28228=AXIS2_PLACEMENT_3D('',#63299,#33185,#33186);
#28229=AXIS2_PLACEMENT_3D('',#63301,#33188,#33189);
#28230=AXIS2_PLACEMENT_3D('',#63302,#33190,#33191);
#28231=AXIS2_PLACEMENT_3D('',#63305,#33194,#33195);
#28232=AXIS2_PLACEMENT_3D('',#63307,#33197,#33198);
#28233=AXIS2_PLACEMENT_3D('',#63309,#33200,#33201);
#28234=AXIS2_PLACEMENT_3D('',#63310,#33202,#33203);
#28235=AXIS2_PLACEMENT_3D('',#63313,#33206,#33207);
#28236=AXIS2_PLACEMENT_3D('',#63315,#33209,#33210);
#28237=AXIS2_PLACEMENT_3D('',#63316,#33211,#33212);
#28238=AXIS2_PLACEMENT_3D('',#63318,#33214,#33215);
#28239=AXIS2_PLACEMENT_3D('',#63320,#33217,#33218);
#28240=AXIS2_PLACEMENT_3D('',#63323,#33221,#33222);
#28241=AXIS2_PLACEMENT_3D('',#63325,#33224,#33225);
#28242=AXIS2_PLACEMENT_3D('',#63327,#33227,#33228);
#28243=AXIS2_PLACEMENT_3D('',#63328,#33229,#33230);
#28244=AXIS2_PLACEMENT_3D('',#63331,#33233,#33234);
#28245=AXIS2_PLACEMENT_3D('',#63332,#33235,#33236);
#28246=AXIS2_PLACEMENT_3D('',#63333,#33237,#33238);
#28247=AXIS2_PLACEMENT_3D('',#63336,#33241,#33242);
#28248=AXIS2_PLACEMENT_3D('',#63338,#33244,#33245);
#28249=AXIS2_PLACEMENT_3D('',#63340,#33247,#33248);
#28250=AXIS2_PLACEMENT_3D('',#63341,#33249,#33250);
#28251=AXIS2_PLACEMENT_3D('',#63344,#33253,#33254);
#28252=AXIS2_PLACEMENT_3D('',#63346,#33256,#33257);
#28253=AXIS2_PLACEMENT_3D('',#63348,#33259,#33260);
#28254=AXIS2_PLACEMENT_3D('',#63349,#33261,#33262);
#28255=AXIS2_PLACEMENT_3D('',#63351,#33264,#33265);
#28256=AXIS2_PLACEMENT_3D('',#63353,#33267,#33268);
#28257=AXIS2_PLACEMENT_3D('',#63355,#33270,#33271);
#28258=AXIS2_PLACEMENT_3D('',#63358,#33274,#33275);
#28259=AXIS2_PLACEMENT_3D('',#63360,#33277,#33278);
#28260=AXIS2_PLACEMENT_3D('',#63361,#33279,#33280);
#28261=AXIS2_PLACEMENT_3D('',#63363,#33282,#33283);
#28262=AXIS2_PLACEMENT_3D('',#63365,#33285,#33286);
#28263=AXIS2_PLACEMENT_3D('',#63368,#33289,#33290);
#28264=AXIS2_PLACEMENT_3D('',#63370,#33292,#33293);
#28265=AXIS2_PLACEMENT_3D('',#63372,#33295,#33296);
#28266=AXIS2_PLACEMENT_3D('',#63373,#33297,#33298);
#28267=AXIS2_PLACEMENT_3D('',#63376,#33301,#33302);
#28268=AXIS2_PLACEMENT_3D('',#63377,#33303,#33304);
#28269=AXIS2_PLACEMENT_3D('',#63378,#33305,#33306);
#28270=AXIS2_PLACEMENT_3D('',#63382,#33309,#33310);
#28271=AXIS2_PLACEMENT_3D('',#63385,#33313,#33314);
#28272=AXIS2_PLACEMENT_3D('',#63387,#33316,#33317);
#28273=AXIS2_PLACEMENT_3D('',#63389,#33319,#33320);
#28274=AXIS2_PLACEMENT_3D('',#63390,#33321,#33322);
#28275=AXIS2_PLACEMENT_3D('',#63393,#33325,#33326);
#28276=AXIS2_PLACEMENT_3D('',#63395,#33328,#33329);
#28277=AXIS2_PLACEMENT_3D('',#63396,#33330,#33331);
#28278=AXIS2_PLACEMENT_3D('',#63645,#33333,#33334);
#28279=AXIS2_PLACEMENT_3D('',#63647,#33335,#33336);
#28280=AXIS2_PLACEMENT_3D('',#63649,#33338,#33339);
#28281=AXIS2_PLACEMENT_3D('',#63651,#33340,#33341);
#28282=AXIS2_PLACEMENT_3D('',#63654,#33343,#33344);
#28283=AXIS2_PLACEMENT_3D('',#63655,#33345,#33346);
#28284=AXIS2_PLACEMENT_3D('',#63657,#33348,#33349);
#28285=AXIS2_PLACEMENT_3D('',#63659,#33351,#33352);
#28286=AXIS2_PLACEMENT_3D('',#63662,#33354,#33355);
#28287=AXIS2_PLACEMENT_3D('',#63666,#33358,#33359);
#28288=AXIS2_PLACEMENT_3D('',#63668,#33361,#33362);
#28289=AXIS2_PLACEMENT_3D('',#63672,#33365,#33366);
#28290=AXIS2_PLACEMENT_3D('',#63673,#33367,#33368);
#28291=AXIS2_PLACEMENT_3D('',#63674,#33369,#33370);
#28292=AXIS2_PLACEMENT_3D('',#63675,#33371,#33372);
#28293=AXIS2_PLACEMENT_3D('',#63676,#33373,#33374);
#28294=AXIS2_PLACEMENT_3D('',#63677,#33375,#33376);
#28295=AXIS2_PLACEMENT_3D('',#63678,#33377,#33378);
#28296=AXIS2_PLACEMENT_3D('',#63680,#33380,#33381);
#28297=AXIS2_PLACEMENT_3D('',#63681,#33382,#33383);
#28298=AXIS2_PLACEMENT_3D('',#63682,#33384,#33385);
#28299=AXIS2_PLACEMENT_3D('',#63683,#33386,#33387);
#28300=AXIS2_PLACEMENT_3D('',#63687,#33390,#33391);
#28301=AXIS2_PLACEMENT_3D('',#63689,#33393,#33394);
#28302=AXIS2_PLACEMENT_3D('',#63691,#33396,#33397);
#28303=AXIS2_PLACEMENT_3D('',#63692,#33398,#33399);
#28304=AXIS2_PLACEMENT_3D('',#63693,#33400,#33401);
#31134=DIRECTION('axis',(0.,0.,1.));
#31135=DIRECTION('refdir',(1.,0.,0.));
#31136=DIRECTION('center_axis',(0.819152044289004,0.,-0.573576436351029));
#31137=DIRECTION('ref_axis',(-0.573576436351029,0.,-0.819152044289004));
#31138=DIRECTION('',(0.497542812164512,-0.497542812164512,0.710564775461646));
#31139=DIRECTION('',(0.,-1.,0.));
#31140=DIRECTION('',(-0.497542812164512,-0.497542812164512,-0.710564775461646));
#31141=DIRECTION('',(-0.497542812164487,0.497542812164587,-0.71056477546161));
#31142=DIRECTION('',(0.,1.,0.));
#31143=DIRECTION('',(0.4975428121645,0.497542812164547,0.710564775461629));
#31144=DIRECTION('center_axis',(0.24184476264798,0.707106781186536,-0.664463024388686));
#31145=DIRECTION('ref_axis',(-0.939692620785908,0.,-0.342020143325669));
#31146=DIRECTION('',(-0.939692620785908,0.,-0.342020143325669));
#31147=DIRECTION('',(-0.633687274224646,0.63368727422465,0.443712606279642));
#31148=DIRECTION('',(0.939692620785908,0.,0.342020143325669));
#31149=DIRECTION('',(0.633687274224648,-0.633687274224648,-0.44371260627964));
#31150=DIRECTION('center_axis',(-0.342020143325669,0.,0.939692620785908));
#31151=DIRECTION('ref_axis',(0.939692620785908,0.,0.342020143325669));
#31152=DIRECTION('',(0.939692620785908,0.,0.342020143325669));
#31153=DIRECTION('',(0.,1.,0.));
#31154=DIRECTION('center_axis',(0.241844762647992,-0.707106781186498,-0.664463024388721));
#31155=DIRECTION('ref_axis',(-0.939692620785908,0.,-0.342020143325669));
#31156=DIRECTION('',(-0.633687274224669,-0.633687274224669,0.443712606279582));
#31157=DIRECTION('',(-0.939692620785908,0.,-0.342020143325669));
#31158=DIRECTION('',(0.633687274224669,0.633687274224671,-0.443712606279578));
#31159=DIRECTION('center_axis',(0.819152044289004,0.,-0.573576436351029));
#31160=DIRECTION('ref_axis',(-0.573576436351029,0.,-0.819152044289004));
#31161=DIRECTION('',(0.497542812164512,-0.497542812164512,0.710564775461646));
#31162=DIRECTION('',(0.,-1.,0.));
#31163=DIRECTION('',(-0.497542812164512,-0.497542812164512,-0.710564775461646));
#31164=DIRECTION('',(-0.497542812164499,0.497542812164549,-0.710564775461628));
#31165=DIRECTION('',(0.,1.,0.));
#31166=DIRECTION('',(0.4975428121645,0.497542812164547,0.710564775461629));
#31167=DIRECTION('center_axis',(0.24184476264798,0.707106781186535,-0.664463024388686));
#31168=DIRECTION('ref_axis',(-0.939692620785908,0.,-0.342020143325669));
#31169=DIRECTION('',(-0.939692620785908,0.,-0.342020143325669));
#31170=DIRECTION('',(-0.633687274224646,0.63368727422465,0.443712606279641));
#31171=DIRECTION('',(0.939692620785908,0.,0.342020143325669));
#31172=DIRECTION('',(0.633687274224649,-0.633687274224649,-0.443712606279638));
#31173=DIRECTION('center_axis',(-0.342020143325669,0.,0.939692620785908));
#31174=DIRECTION('ref_axis',(0.939692620785908,0.,0.342020143325669));
#31175=DIRECTION('',(0.939692620785908,0.,0.342020143325669));
#31176=DIRECTION('',(0.,1.,0.));
#31177=DIRECTION('center_axis',(0.24184476264798,-0.707106781186533,-0.664463024388688));
#31178=DIRECTION('ref_axis',(-0.939692620785908,0.,-0.342020143325669));
#31179=DIRECTION('',(-0.63368727422465,-0.63368727422465,0.443712606279635));
#31180=DIRECTION('',(-0.939692620785908,0.,-0.342020143325669));
#31181=DIRECTION('',(0.633687274224652,0.633687274224654,-0.443712606279627));
#31182=DIRECTION('center_axis',(0.819152044289004,0.,-0.573576436351029));
#31183=DIRECTION('ref_axis',(-0.573576436351029,0.,-0.819152044289004));
#31184=DIRECTION('',(0.497542812164512,-0.497542812164512,0.710564775461646));
#31185=DIRECTION('',(0.,-1.,0.));
#31186=DIRECTION('',(-0.497542812164512,-0.497542812164512,-0.710564775461646));
#31187=DIRECTION('',(-0.497542812164502,0.497542812164542,-0.710564775461631));
#31188=DIRECTION('',(0.,1.,0.));
#31189=DIRECTION('',(0.497542812164502,0.49754281216454,0.710564775461632));
#31190=DIRECTION('center_axis',(-0.342020143325678,0.,0.939692620785905));
#31191=DIRECTION('ref_axis',(0.939692620785905,0.,0.342020143325678));
#31192=DIRECTION('',(0.939692620785905,0.,0.342020143325678));
#31193=DIRECTION('',(0.,1.,0.));
#31194=DIRECTION('',(-0.939692620785905,0.,-0.342020143325678));
#31195=DIRECTION('center_axis',(0.241844762647986,-0.707106781186536,-0.664463024388684));
#31196=DIRECTION('ref_axis',(-0.939692620785905,0.,-0.342020143325678));
#31197=DIRECTION('',(-0.63368727422465,-0.63368727422465,0.443712606279636));
#31198=DIRECTION('',(-0.939692620785905,0.,-0.342020143325678));
#31199=DIRECTION('',(0.633687274224652,0.633687274224654,-0.443712606279627));
#31200=DIRECTION('center_axis',(0.707106781186548,-0.707106781186548,0.));
#31201=DIRECTION('ref_axis',(0.,0.,-1.));
#31202=DIRECTION('',(0.,0.,1.));
#31203=DIRECTION('',(0.497542812164512,0.497542812164512,-0.710564775461646));
#31204=DIRECTION('',(0.63368727422465,0.63368727422465,0.443712606279634));
#31205=DIRECTION('',(0.,0.,-1.));
#31206=DIRECTION('center_axis',(0.819152044289001,0.,-0.573576436351034));
#31207=DIRECTION('ref_axis',(-0.573576436351034,0.,-0.819152044289001));
#31208=DIRECTION('',(0.497542812164515,-0.497542812164515,0.710564775461641));
#31209=DIRECTION('',(0.,-1.,0.));
#31210=DIRECTION('',(-0.497542812164515,-0.497542812164515,-0.710564775461641));
#31211=DIRECTION('',(-0.497542812164508,0.497542812164537,-0.710564775461631));
#31212=DIRECTION('',(0.,1.,0.));
#31213=DIRECTION('',(0.49754281216452,0.497542812164499,0.710564775461649));
#31214=DIRECTION('center_axis',(0.241844762647973,0.707106781186573,-0.664463024388649));
#31215=DIRECTION('ref_axis',(-0.939692620785905,0.,-0.342020143325678));
#31216=DIRECTION('',(-0.939692620785905,0.,-0.342020143325678));
#31217=DIRECTION('',(-0.633687274224627,0.633687274224631,0.443712606279695));
#31218=DIRECTION('',(0.939692620785905,0.,0.342020143325678));
#31219=DIRECTION('',(0.63368727422463,-0.63368727422463,-0.443712606279693));
#31220=DIRECTION('center_axis',(-0.342020143325678,0.,0.939692620785905));
#31221=DIRECTION('ref_axis',(0.939692620785905,0.,0.342020143325678));
#31222=DIRECTION('',(0.939692620785905,0.,0.342020143325678));
#31223=DIRECTION('',(0.,1.,0.));
#31224=DIRECTION('center_axis',(0.241844762647985,-0.707106781186537,-0.664463024388682));
#31225=DIRECTION('ref_axis',(-0.939692620785905,0.,-0.342020143325678));
#31226=DIRECTION('',(-0.633687274224649,-0.633687274224649,0.443712606279638));
#31227=DIRECTION('',(-0.939692620785905,0.,-0.342020143325678));
#31228=DIRECTION('',(0.633687274224652,0.633687274224654,-0.443712606279627));
#31229=DIRECTION('center_axis',(0.819152044289004,0.,-0.573576436351029));
#31230=DIRECTION('ref_axis',(-0.573576436351029,0.,-0.819152044289004));
#31231=DIRECTION('',(0.497542812164512,-0.497542812164512,0.710564775461646));
#31232=DIRECTION('',(0.,-1.,0.));
#31233=DIRECTION('',(-0.497542812164512,-0.497542812164512,-0.710564775461646));
#31234=DIRECTION('',(-0.4975428121645,0.497542812164547,-0.710564775461629));
#31235=DIRECTION('',(0.,1.,0.));
#31236=DIRECTION('',(0.497542812164501,0.497542812164546,0.71056477546163));
#31237=DIRECTION('center_axis',(1.,0.,0.));
#31238=DIRECTION('ref_axis',(0.,1.,0.));
#31239=DIRECTION('',(0.,0.,-1.));
#31240=DIRECTION('',(0.,1.,0.));
#31241=DIRECTION('',(0.,0.,1.));
#31242=DIRECTION('center_axis',(0.707106781186548,0.707106781186548,0.));
#31243=DIRECTION('ref_axis',(0.,0.,-1.));
#31244=DIRECTION('',(0.633687274224648,-0.633687274224648,-0.443712606279641));
#31245=DIRECTION('',(0.,0.,1.));
#31246=DIRECTION('',(-0.633687274224686,0.633687274224686,-0.443712606279532));
#31247=DIRECTION('',(-0.497542812164537,0.497542812164537,0.71056477546161));
#31248=DIRECTION('center_axis',(0.241844762647979,0.707106781186536,-0.664463024388685));
#31249=DIRECTION('ref_axis',(-0.939692620785908,0.,-0.342020143325669));
#31250=DIRECTION('',(-0.939692620785908,0.,-0.342020143325669));
#31251=DIRECTION('',(-0.633687274224634,0.633687274224638,0.443712606279675));
#31252=DIRECTION('',(0.939692620785908,0.,0.342020143325669));
#31253=DIRECTION('center_axis',(0.819152044289002,0.,0.573576436351031));
#31254=DIRECTION('ref_axis',(0.573576436351031,0.,-0.819152044289002));
#31255=DIRECTION('',(0.497542812164513,0.497542812164513,-0.710564775461643));
#31256=DIRECTION('',(0.,1.,0.));
#31257=DIRECTION('',(-0.497542812164513,0.497542812164513,0.710564775461643));
#31258=DIRECTION('',(-0.497542812164503,-0.497542812164545,0.710564775461628));
#31259=DIRECTION('',(0.,-1.,0.));
#31260=DIRECTION('',(0.497542812164502,-0.497542812164547,-0.710564775461627));
#31261=DIRECTION('center_axis',(0.24184476264798,0.707106781186536,0.664463024388686));
#31262=DIRECTION('ref_axis',(0.939692620785908,0.,-0.342020143325669));
#31263=DIRECTION('',(-0.633687274224648,0.633687274224648,-0.44371260627964));
#31264=DIRECTION('',(-0.939692620785908,0.,0.342020143325669));
#31265=DIRECTION('',(-0.633687274224657,0.633687274224651,-0.443712606279624));
#31266=DIRECTION('',(0.939692620785908,0.,-0.342020143325669));
#31267=DIRECTION('center_axis',(0.707106781186548,0.707106781186548,0.));
#31268=DIRECTION('ref_axis',(0.,0.,-1.));
#31269=DIRECTION('',(0.,0.,-1.));
#31270=DIRECTION('',(0.497542812164488,-0.497542812164488,0.710564775461679));
#31271=DIRECTION('',(0.633687274224649,-0.633687274224649,-0.443712606279638));
#31272=DIRECTION('',(0.,0.,1.));
#31273=DIRECTION('center_axis',(1.,0.,0.));
#31274=DIRECTION('ref_axis',(0.,1.,0.));
#31275=DIRECTION('',(0.,0.,1.));
#31276=DIRECTION('',(0.,-1.,0.));
#31277=DIRECTION('center_axis',(0.81915204428903,0.,-0.573576436350992));
#31278=DIRECTION('ref_axis',(-0.573576436350992,0.,-0.81915204428903));
#31279=DIRECTION('',(-0.497542812164488,-0.497542812164488,-0.710564775461679));
#31280=DIRECTION('',(-0.497542812164461,0.49754281216457,-0.710564775461641));
#31281=DIRECTION('',(0.,1.,0.));
#31282=DIRECTION('',(0.49754281216446,0.497542812164572,0.71056477546164));
#31283=DIRECTION('center_axis',(0.24184476264798,0.707106781186534,-0.664463024388687));
#31284=DIRECTION('ref_axis',(-0.939692620785908,0.,-0.342020143325669));
#31285=DIRECTION('',(-0.939692620785908,0.,-0.342020143325669));
#31286=DIRECTION('',(-0.633687274224651,0.633687274224655,0.443712606279627));
#31287=DIRECTION('',(0.939692620785908,0.,0.342020143325669));
#31288=DIRECTION('center_axis',(0.819152044289004,0.,0.573576436351029));
#31289=DIRECTION('ref_axis',(0.573576436351029,0.,-0.819152044289004));
#31290=DIRECTION('',(0.497542812164512,0.497542812164512,-0.710564775461646));
#31291=DIRECTION('',(0.,1.,0.));
#31292=DIRECTION('',(-0.497542812164512,0.497542812164512,0.710564775461646));
#31293=DIRECTION('',(-0.4975428121645,-0.497542812164548,0.710564775461629));
#31294=DIRECTION('',(0.,-1.,0.));
#31295=DIRECTION('',(0.497542812164488,-0.497542812164584,-0.710564775461612));
#31296=DIRECTION('center_axis',(-0.342020143325669,0.,-0.939692620785908));
#31297=DIRECTION('ref_axis',(-0.939692620785908,0.,0.342020143325669));
#31298=DIRECTION('',(0.939692620785908,0.,-0.342020143325669));
#31299=DIRECTION('',(0.,1.,0.));
#31300=DIRECTION('',(-0.939692620785908,0.,0.342020143325669));
#31301=DIRECTION('center_axis',(0.24184476264798,0.707106781186534,0.664463024388687));
#31302=DIRECTION('ref_axis',(0.939692620785908,0.,-0.342020143325669));
#31303=DIRECTION('',(-0.633687274224649,0.633687274224649,-0.443712606279638));
#31304=DIRECTION('',(-0.939692620785908,0.,0.342020143325669));
#31305=DIRECTION('',(-0.633687274224654,0.633687274224652,-0.443712606279625));
#31306=DIRECTION('center_axis',(0.707106781186548,0.707106781186548,0.));
#31307=DIRECTION('ref_axis',(0.,0.,-1.));
#31308=DIRECTION('',(0.,0.,1.));
#31309=DIRECTION('',(0.,0.,-1.));
#31310=DIRECTION('center_axis',(0.819152044288976,0.,-0.573576436351068));
#31311=DIRECTION('ref_axis',(-0.573576436351068,0.,-0.819152044288976));
#31312=DIRECTION('',(0.497542812164537,-0.497542812164537,0.71056477546161));
#31313=DIRECTION('',(0.,-1.,0.));
#31314=DIRECTION('',(-0.497542812164537,-0.497542812164537,-0.71056477546161));
#31315=DIRECTION('',(-0.497542812164543,0.497542812164522,-0.710564775461617));
#31316=DIRECTION('',(0.,1.,0.));
#31317=DIRECTION('',(0.497542812164529,0.497542812164561,0.710564775461598));
#31318=DIRECTION('center_axis',(1.,0.,0.));
#31319=DIRECTION('ref_axis',(0.,1.,0.));
#31320=DIRECTION('',(0.,0.,-1.));
#31321=DIRECTION('',(0.,1.,0.));
#31322=DIRECTION('',(0.,0.,1.));
#31323=DIRECTION('center_axis',(0.707106781186548,0.707106781186548,0.));
#31324=DIRECTION('ref_axis',(0.,0.,-1.));
#31325=DIRECTION('',(0.633687274224669,-0.633687274224669,-0.443712606279581));
#31326=DIRECTION('',(0.,0.,1.));
#31327=DIRECTION('',(-0.633687274224648,0.633687274224648,-0.44371260627964));
#31328=DIRECTION('',(-0.497542812164512,0.497542812164512,0.710564775461646));
#31329=DIRECTION('center_axis',(0.241844762647993,0.707106781186498,-0.664463024388722));
#31330=DIRECTION('ref_axis',(-0.939692620785908,0.,-0.342020143325669));
#31331=DIRECTION('',(-0.939692620785908,0.,-0.342020143325669));
#31332=DIRECTION('',(-0.633687274224668,0.633687274224672,0.443712606279579));
#31333=DIRECTION('',(0.939692620785908,0.,0.342020143325669));
#31334=DIRECTION('center_axis',(0.819152044289004,0.,0.573576436351029));
#31335=DIRECTION('ref_axis',(0.573576436351029,0.,-0.819152044289004));
#31336=DIRECTION('',(0.497542812164512,0.497542812164512,-0.710564775461646));
#31337=DIRECTION('',(0.,1.,0.));
#31338=DIRECTION('',(-0.497542812164512,0.497542812164512,0.710564775461646));
#31339=DIRECTION('',(-0.4975428121645,-0.497542812164547,0.710564775461629));
#31340=DIRECTION('',(0.,-1.,0.));
#31341=DIRECTION('',(0.497542812164487,-0.497542812164587,-0.71056477546161));
#31342=DIRECTION('center_axis',(0.24184476264798,0.707106781186535,0.664463024388686));
#31343=DIRECTION('ref_axis',(0.939692620785908,0.,-0.342020143325669));
#31344=DIRECTION('',(-0.633687274224649,0.633687274224649,-0.443712606279638));
#31345=DIRECTION('',(-0.939692620785908,0.,0.342020143325669));
#31346=DIRECTION('',(-0.633687274224652,0.633687274224654,-0.443712606279627));
#31347=DIRECTION('',(0.939692620785908,0.,-0.342020143325669));
#31348=DIRECTION('center_axis',(0.707106781186548,0.707106781186548,0.));
#31349=DIRECTION('ref_axis',(0.,0.,-1.));
#31350=DIRECTION('',(0.,0.,-1.));
#31351=DIRECTION('',(0.497542812164512,-0.497542812164512,0.710564775461646));
#31352=DIRECTION('',(0.633687274224649,-0.633687274224649,-0.443712606279638));
#31353=DIRECTION('',(0.,0.,1.));
#31354=DIRECTION('center_axis',(1.,0.,0.));
#31355=DIRECTION('ref_axis',(0.,1.,0.));
#31356=DIRECTION('',(0.,0.,1.));
#31357=DIRECTION('',(0.,-1.,0.));
#31358=DIRECTION('center_axis',(0.819152044289004,0.,-0.573576436351029));
#31359=DIRECTION('ref_axis',(-0.573576436351029,0.,-0.819152044289004));
#31360=DIRECTION('',(-0.497542812164512,-0.497542812164512,-0.710564775461646));
#31361=DIRECTION('',(-0.497542812164501,0.497542812164546,-0.71056477546163));
#31362=DIRECTION('',(0.,1.,0.));
#31363=DIRECTION('',(0.4975428121645,0.497542812164548,0.710564775461629));
#31364=DIRECTION('center_axis',(0.24184476264798,0.707106781186535,-0.664463024388687));
#31365=DIRECTION('ref_axis',(-0.939692620785908,0.,-0.342020143325669));
#31366=DIRECTION('',(-0.939692620785908,0.,-0.342020143325669));
#31367=DIRECTION('',(-0.633687274224651,0.633687274224655,0.443712606279627));
#31368=DIRECTION('',(0.939692620785908,0.,0.342020143325669));
#31369=DIRECTION('center_axis',(0.819152044289004,0.,0.573576436351029));
#31370=DIRECTION('ref_axis',(0.573576436351029,0.,-0.819152044289004));
#31371=DIRECTION('',(0.497542812164512,0.497542812164512,-0.710564775461646));
#31372=DIRECTION('',(0.,1.,0.));
#31373=DIRECTION('',(-0.497542812164512,0.497542812164512,0.710564775461646));
#31374=DIRECTION('',(-0.4975428121645,-0.497542812164549,0.710564775461628));
#31375=DIRECTION('',(0.,-1.,0.));
#31376=DIRECTION('',(0.4975428121645,-0.497542812164546,-0.710564775461629));
#31377=DIRECTION('center_axis',(-0.342020143325669,0.,-0.939692620785908));
#31378=DIRECTION('ref_axis',(-0.939692620785908,0.,0.342020143325669));
#31379=DIRECTION('',(0.939692620785908,0.,-0.342020143325669));
#31380=DIRECTION('',(0.,1.,0.));
#31381=DIRECTION('',(-0.939692620785908,0.,0.342020143325669));
#31382=DIRECTION('center_axis',(0.24184476264798,0.707106781186534,0.664463024388688));
#31383=DIRECTION('ref_axis',(0.939692620785908,0.,-0.342020143325669));
#31384=DIRECTION('',(-0.63368727422465,0.63368727422465,-0.443712606279636));
#31385=DIRECTION('',(-0.939692620785908,0.,0.342020143325669));
#31386=DIRECTION('',(-0.63368727422465,0.633687274224655,-0.443712606279628));
#31387=DIRECTION('center_axis',(0.707106781186548,0.707106781186548,0.));
#31388=DIRECTION('ref_axis',(0.,0.,-1.));
#31389=DIRECTION('',(0.,0.,1.));
#31390=DIRECTION('',(0.,0.,-1.));
#31391=DIRECTION('center_axis',(0.819152044289004,0.,0.573576436351029));
#31392=DIRECTION('ref_axis',(0.573576436351029,0.,-0.819152044289004));
#31393=DIRECTION('',(0.497542812164512,0.497542812164512,-0.710564775461646));
#31394=DIRECTION('',(0.,1.,0.));
#31395=DIRECTION('',(-0.497542812164512,0.497542812164512,0.710564775461646));
#31396=DIRECTION('',(-0.4975428121645,-0.497542812164546,0.710564775461629));
#31397=DIRECTION('',(0.,-1.,0.));
#31398=DIRECTION('',(0.4975428121645,-0.497542812164548,-0.710564775461629));
#31399=DIRECTION('center_axis',(0.24184476264798,0.707106781186536,0.664463024388686));
#31400=DIRECTION('ref_axis',(0.939692620785908,0.,-0.342020143325669));
#31401=DIRECTION('',(-0.633687274224648,0.633687274224648,-0.44371260627964));
#31402=DIRECTION('',(-0.939692620785908,0.,0.342020143325669));
#31403=DIRECTION('',(-0.633687274224659,0.633687274224649,-0.443712606279623));
#31404=DIRECTION('',(0.939692620785908,0.,-0.342020143325669));
#31405=DIRECTION('center_axis',(0.707106781186548,0.707106781186548,0.));
#31406=DIRECTION('ref_axis',(0.,0.,-1.));
#31407=DIRECTION('',(0.,0.,-1.));
#31408=DIRECTION('',(0.497542812164537,-0.497542812164537,0.71056477546161));
#31409=DIRECTION('',(0.633687274224667,-0.633687274224667,-0.443712606279587));
#31410=DIRECTION('',(0.,0.,1.));
#31411=DIRECTION('center_axis',(1.,0.,0.));
#31412=DIRECTION('ref_axis',(0.,1.,0.));
#31413=DIRECTION('',(0.,0.,1.));
#31414=DIRECTION('',(0.,-1.,0.));
#31415=DIRECTION('center_axis',(0.819152044288976,0.,-0.573576436351068));
#31416=DIRECTION('ref_axis',(-0.573576436351068,0.,-0.819152044288976));
#31417=DIRECTION('',(-0.497542812164537,-0.497542812164537,-0.71056477546161));
#31418=DIRECTION('',(-0.49754281216453,0.497542812164559,-0.710564775461599));
#31419=DIRECTION('',(0.,1.,0.));
#31420=DIRECTION('',(0.497542812164531,0.497542812164557,0.7105647754616));
#31421=DIRECTION('center_axis',(0.241844762647991,0.707106781186501,-0.664463024388718));
#31422=DIRECTION('ref_axis',(-0.939692620785908,0.,-0.342020143325669));
#31423=DIRECTION('',(-0.939692620785908,0.,-0.342020143325669));
#31424=DIRECTION('',(-0.633687274224651,0.633687274224655,0.443712606279627));
#31425=DIRECTION('',(0.939692620785908,0.,0.342020143325669));
#31426=DIRECTION('center_axis',(0.819152044289004,0.,0.573576436351029));
#31427=DIRECTION('ref_axis',(0.573576436351029,0.,-0.819152044289004));
#31428=DIRECTION('',(0.497542812164512,0.497542812164512,-0.710564775461646));
#31429=DIRECTION('',(0.,1.,0.));
#31430=DIRECTION('',(-0.497542812164512,0.497542812164512,0.710564775461646));
#31431=DIRECTION('',(-0.4975428121645,-0.497542812164548,0.710564775461629));
#31432=DIRECTION('',(0.,-1.,0.));
#31433=DIRECTION('',(0.497542812164488,-0.497542812164583,-0.710564775461612));
#31434=DIRECTION('center_axis',(-0.342020143325669,0.,-0.939692620785908));
#31435=DIRECTION('ref_axis',(-0.939692620785908,0.,0.342020143325669));
#31436=DIRECTION('',(0.939692620785908,0.,-0.342020143325669));
#31437=DIRECTION('',(0.,1.,0.));
#31438=DIRECTION('',(-0.939692620785908,0.,0.342020143325669));
#31439=DIRECTION('center_axis',(0.24184476264798,0.707106781186534,0.664463024388687));
#31440=DIRECTION('ref_axis',(0.939692620785908,0.,-0.342020143325669));
#31441=DIRECTION('',(-0.633687274224649,0.633687274224649,-0.443712606279638));
#31442=DIRECTION('',(-0.939692620785908,0.,0.342020143325669));
#31443=DIRECTION('',(-0.633687274224652,0.633687274224654,-0.443712606279627));
#31444=DIRECTION('center_axis',(0.707106781186548,0.707106781186548,0.));
#31445=DIRECTION('ref_axis',(0.,0.,-1.));
#31446=DIRECTION('',(0.,0.,-1.));
#31447=DIRECTION('',(0.497542812164512,-0.497542812164512,0.710564775461646));
#31448=DIRECTION('',(0.633687274224649,-0.633687274224649,-0.443712606279638));
#31449=DIRECTION('',(0.,0.,1.));
#31450=DIRECTION('center_axis',(0.819152044289004,0.,-0.573576436351029));
#31451=DIRECTION('ref_axis',(-0.573576436351029,0.,-0.819152044289004));
#31452=DIRECTION('',(0.,-1.,0.));
#31453=DIRECTION('',(-0.497542812164512,-0.497542812164512,-0.710564775461646));
#31454=DIRECTION('',(-0.497542812164501,0.497542812164545,-0.71056477546163));
#31455=DIRECTION('',(0.,1.,0.));
#31456=DIRECTION('',(0.4975428121645,0.497542812164548,0.710564775461629));
#31457=DIRECTION('center_axis',(-0.342020143325669,0.,0.939692620785908));
#31458=DIRECTION('ref_axis',(0.939692620785908,0.,0.342020143325669));
#31459=DIRECTION('',(0.939692620785908,0.,0.342020143325669));
#31460=DIRECTION('',(0.,1.,0.));
#31461=DIRECTION('',(-0.939692620785908,0.,-0.342020143325669));
#31462=DIRECTION('center_axis',(0.241844762647979,-0.707106781186537,-0.664463024388685));
#31463=DIRECTION('ref_axis',(-0.939692620785908,0.,-0.342020143325669));
#31464=DIRECTION('',(-0.633687274224648,-0.633687274224648,0.443712606279641));
#31465=DIRECTION('',(-0.939692620785908,0.,-0.342020143325669));
#31466=DIRECTION('',(0.633687274224635,0.633687274224637,-0.443712606279675));
#31467=DIRECTION('center_axis',(0.707106781186548,-0.707106781186548,0.));
#31468=DIRECTION('ref_axis',(0.,0.,-1.));
#31469=DIRECTION('',(0.633687274224667,0.633687274224667,0.443712606279586));
#31470=DIRECTION('',(0.,0.,-1.));
#31471=DIRECTION('',(0.,0.,1.));
#31472=DIRECTION('center_axis',(0.819152044289004,0.,0.573576436351029));
#31473=DIRECTION('ref_axis',(0.573576436351029,0.,-0.819152044289004));
#31474=DIRECTION('',(0.497542812164512,0.497542812164512,-0.710564775461646));
#31475=DIRECTION('',(0.,1.,0.));
#31476=DIRECTION('',(-0.497542812164512,0.497542812164512,0.710564775461646));
#31477=DIRECTION('',(-0.4975428121645,-0.497542812164549,0.710564775461628));
#31478=DIRECTION('',(0.,-1.,0.));
#31479=DIRECTION('',(0.4975428121645,-0.497542812164546,-0.710564775461629));
#31480=DIRECTION('center_axis',(0.24184476264798,0.707106781186534,0.664463024388688));
#31481=DIRECTION('ref_axis',(0.939692620785908,0.,-0.342020143325669));
#31482=DIRECTION('',(-0.63368727422465,0.63368727422465,-0.443712606279636));
#31483=DIRECTION('',(-0.939692620785908,0.,0.342020143325669));
#31484=DIRECTION('',(-0.63368727422465,0.633687274224655,-0.443712606279628));
#31485=DIRECTION('',(0.939692620785908,0.,-0.342020143325669));
#31486=DIRECTION('center_axis',(0.707106781186548,0.707106781186548,0.));
#31487=DIRECTION('ref_axis',(0.,0.,-1.));
#31488=DIRECTION('',(0.,0.,-1.));
#31489=DIRECTION('',(0.497542812164512,-0.497542812164512,0.710564775461646));
#31490=DIRECTION('',(0.633687274224648,-0.633687274224648,-0.44371260627964));
#31491=DIRECTION('',(0.,0.,1.));
#31492=DIRECTION('center_axis',(1.,0.,0.));
#31493=DIRECTION('ref_axis',(0.,1.,0.));
#31494=DIRECTION('',(0.,0.,1.));
#31495=DIRECTION('',(0.,-1.,0.));
#31496=DIRECTION('center_axis',(0.819152044289004,0.,-0.573576436351029));
#31497=DIRECTION('ref_axis',(-0.573576436351029,0.,-0.819152044289004));
#31498=DIRECTION('',(-0.497542812164512,-0.497542812164512,-0.710564775461646));
#31499=DIRECTION('',(-0.497542812164512,0.49754281216451,-0.710564775461646));
#31500=DIRECTION('',(0.,1.,0.));
#31501=DIRECTION('',(0.4975428121645,0.497542812164546,0.710564775461629));
#31502=DIRECTION('center_axis',(0.241844762647979,0.707106781186536,-0.664463024388685));
#31503=DIRECTION('ref_axis',(-0.939692620785908,0.,-0.342020143325669));
#31504=DIRECTION('',(-0.939692620785908,0.,-0.342020143325669));
#31505=DIRECTION('',(-0.633687274224634,0.633687274224638,0.443712606279675));
#31506=DIRECTION('',(0.939692620785908,0.,0.342020143325669));
#31507=DIRECTION('center_axis',(0.819152044289004,0.,0.573576436351029));
#31508=DIRECTION('ref_axis',(0.573576436351029,0.,-0.819152044289004));
#31509=DIRECTION('',(0.497542812164512,0.497542812164512,-0.710564775461646));
#31510=DIRECTION('',(0.,1.,0.));
#31511=DIRECTION('',(-0.497542812164512,0.497542812164512,0.710564775461646));
#31512=DIRECTION('',(-0.4975428121645,-0.497542812164546,0.710564775461629));
#31513=DIRECTION('',(0.,-1.,0.));
#31514=DIRECTION('',(0.4975428121645,-0.497542812164549,-0.710564775461628));
#31515=DIRECTION('center_axis',(0.24184476264798,0.707106781186536,0.664463024388686));
#31516=DIRECTION('ref_axis',(0.939692620785908,0.,-0.342020143325669));
#31517=DIRECTION('',(-0.633687274224648,0.633687274224648,-0.44371260627964));
#31518=DIRECTION('',(-0.939692620785908,0.,0.342020143325669));
#31519=DIRECTION('',(-0.633687274224658,0.63368727422465,-0.443712606279624));
#31520=DIRECTION('',(0.939692620785908,0.,-0.342020143325669));
#31521=DIRECTION('center_axis',(0.707106781186548,0.707106781186548,0.));
#31522=DIRECTION('ref_axis',(0.,0.,-1.));
#31523=DIRECTION('',(0.,0.,-1.));
#31524=DIRECTION('',(0.497542812164537,-0.497542812164537,0.71056477546161));
#31525=DIRECTION('',(0.633687274224669,-0.633687274224669,-0.443712606279581));
#31526=DIRECTION('',(0.,0.,1.));
#31527=DIRECTION('center_axis',(1.,0.,0.));
#31528=DIRECTION('ref_axis',(0.,1.,0.));
#31529=DIRECTION('',(0.,0.,1.));
#31530=DIRECTION('',(0.,-1.,0.));
#31531=DIRECTION('center_axis',(0.819152044288976,0.,-0.573576436351068));
#31532=DIRECTION('ref_axis',(-0.573576436351068,0.,-0.819152044288976));
#31533=DIRECTION('',(-0.497542812164537,-0.497542812164537,-0.71056477546161));
#31534=DIRECTION('',(-0.49754281216453,0.497542812164559,-0.7105647754616));
#31535=DIRECTION('',(0.,1.,0.));
#31536=DIRECTION('',(0.49754281216453,0.497542812164561,0.710564775461598));
#31537=DIRECTION('center_axis',(0.241844762647993,0.707106781186498,-0.664463024388722));
#31538=DIRECTION('ref_axis',(-0.939692620785908,0.,-0.342020143325669));
#31539=DIRECTION('',(-0.939692620785908,0.,-0.342020143325669));
#31540=DIRECTION('',(-0.633687274224668,0.633687274224672,0.443712606279579));
#31541=DIRECTION('',(0.939692620785908,0.,0.342020143325669));
#31542=DIRECTION('center_axis',(0.819152044289004,0.,0.573576436351029));
#31543=DIRECTION('ref_axis',(0.573576436351029,0.,-0.819152044289004));
#31544=DIRECTION('',(0.497542812164512,0.497542812164512,-0.710564775461646));
#31545=DIRECTION('',(0.,1.,0.));
#31546=DIRECTION('',(-0.497542812164512,0.497542812164512,0.710564775461646));
#31547=DIRECTION('',(-0.4975428121645,-0.497542812164548,0.710564775461629));
#31548=DIRECTION('',(0.,-1.,0.));
#31549=DIRECTION('',(0.497542812164476,-0.497542812164621,-0.710564775461594));
#31550=DIRECTION('center_axis',(0.241844762648004,-0.707106781186466,0.664463024388752));
#31551=DIRECTION('ref_axis',(0.939692620785908,0.,-0.342020143325669));
#31552=DIRECTION('',(-0.939692620785908,0.,0.342020143325669));
#31553=DIRECTION('',(0.633687274224663,0.633687274224675,0.443712606279581));
#31554=DIRECTION('',(0.939692620785908,0.,-0.342020143325669));
#31555=DIRECTION('',(0.633687274224686,0.633687274224686,0.443712606279532));
#31556=DIRECTION('center_axis',(-0.342020143325669,0.,-0.939692620785908));
#31557=DIRECTION('ref_axis',(-0.939692620785908,0.,0.342020143325669));
#31558=DIRECTION('',(0.939692620785908,0.,-0.342020143325669));
#31559=DIRECTION('',(0.,1.,0.));
#31560=DIRECTION('center_axis',(0.24184476264798,0.707106781186534,0.664463024388687));
#31561=DIRECTION('ref_axis',(0.939692620785908,0.,-0.342020143325669));
#31562=DIRECTION('',(-0.633687274224649,0.633687274224649,-0.443712606279638));
#31563=DIRECTION('',(-0.939692620785908,0.,0.342020143325669));
#31564=DIRECTION('',(-0.633687274224652,0.633687274224654,-0.443712606279627));
#31565=DIRECTION('center_axis',(0.819152044289004,0.,0.573576436351029));
#31566=DIRECTION('ref_axis',(0.573576436351029,0.,-0.819152044289004));
#31567=DIRECTION('',(0.497542812164512,0.497542812164512,-0.710564775461646));
#31568=DIRECTION('',(0.,1.,0.));
#31569=DIRECTION('',(-0.497542812164512,0.497542812164512,0.710564775461646));
#31570=DIRECTION('',(-0.497542812164502,-0.497542812164542,0.710564775461631));
#31571=DIRECTION('',(0.,-1.,0.));
#31572=DIRECTION('',(0.497542812164501,-0.497542812164543,-0.710564775461631));
#31573=DIRECTION('center_axis',(0.241844762647986,0.707106781186536,0.664463024388684));
#31574=DIRECTION('ref_axis',(0.939692620785905,0.,-0.342020143325678));
#31575=DIRECTION('',(-0.63368727422465,0.63368727422465,-0.443712606279636));
#31576=DIRECTION('',(-0.939692620785905,0.,0.342020143325678));
#31577=DIRECTION('',(-0.633687274224657,0.633687274224651,-0.443712606279624));
#31578=DIRECTION('',(0.939692620785905,0.,-0.342020143325678));
#31579=DIRECTION('center_axis',(0.707106781186548,0.707106781186548,0.));
#31580=DIRECTION('ref_axis',(0.,0.,-1.));
#31581=DIRECTION('',(0.,0.,-1.));
#31582=DIRECTION('',(0.497542812164512,-0.497542812164512,0.710564775461646));
#31583=DIRECTION('',(0.633687274224648,-0.633687274224648,-0.44371260627964));
#31584=DIRECTION('',(0.,0.,1.));
#31585=DIRECTION('center_axis',(1.,0.,0.));
#31586=DIRECTION('ref_axis',(0.,1.,0.));
#31587=DIRECTION('',(0.,0.,1.));
#31588=DIRECTION('',(0.,-1.,0.));
#31589=DIRECTION('center_axis',(0.819152044289004,0.,-0.573576436351029));
#31590=DIRECTION('ref_axis',(-0.573576436351029,0.,-0.819152044289004));
#31591=DIRECTION('',(-0.497542812164512,-0.497542812164512,-0.710564775461646));
#31592=DIRECTION('',(-0.497542812164515,0.497542812164502,-0.71056477546165));
#31593=DIRECTION('',(0.,1.,0.));
#31594=DIRECTION('',(0.497542812164503,0.497542812164539,0.710564775461633));
#31595=DIRECTION('center_axis',(0.241844762647985,0.707106781186538,-0.664463024388682));
#31596=DIRECTION('ref_axis',(-0.939692620785905,0.,-0.342020143325678));
#31597=DIRECTION('',(-0.939692620785905,0.,-0.342020143325678));
#31598=DIRECTION('',(-0.633687274224634,0.633687274224638,0.443712606279675));
#31599=DIRECTION('',(0.939692620785905,0.,0.342020143325678));
#31600=DIRECTION('center_axis',(0.819152044289007,0.,0.573576436351024));
#31601=DIRECTION('ref_axis',(0.573576436351024,0.,-0.819152044289007));
#31602=DIRECTION('',(0.497542812164509,0.497542812164509,-0.71056477546165));
#31603=DIRECTION('',(0.,1.,0.));
#31604=DIRECTION('',(-0.497542812164509,0.497542812164509,0.71056477546165));
#31605=DIRECTION('',(-0.497542812164497,-0.497542812164545,0.710564775461633));
#31606=DIRECTION('',(0.,-1.,0.));
#31607=DIRECTION('',(0.497542812164509,-0.497542812164509,-0.71056477546165));
#31608=DIRECTION('center_axis',(0.241844762647986,0.707106781186536,0.664463024388684));
#31609=DIRECTION('ref_axis',(0.939692620785905,0.,-0.342020143325678));
#31610=DIRECTION('',(-0.63368727422465,0.63368727422465,-0.443712606279636));
#31611=DIRECTION('',(-0.939692620785905,0.,0.342020143325678));
#31612=DIRECTION('',(-0.633687274224657,0.633687274224651,-0.443712606279624));
#31613=DIRECTION('',(0.939692620785905,0.,-0.342020143325678));
#31614=DIRECTION('center_axis',(0.707106781186548,0.707106781186548,0.));
#31615=DIRECTION('ref_axis',(0.,0.,-1.));
#31616=DIRECTION('',(0.,0.,-1.));
#31617=DIRECTION('',(0.497542812164539,-0.497542812164539,0.710564775461607));
#31618=DIRECTION('',(0.63368727422465,-0.63368727422465,-0.443712606279635));
#31619=DIRECTION('',(0.,0.,1.));
#31620=DIRECTION('center_axis',(1.,0.,0.));
#31621=DIRECTION('ref_axis',(0.,1.,0.));
#31622=DIRECTION('',(0.,0.,1.));
#31623=DIRECTION('',(0.,-1.,0.));
#31624=DIRECTION('center_axis',(0.819152044288975,0.,-0.573576436351071));
#31625=DIRECTION('ref_axis',(-0.573576436351071,0.,-0.819152044288975));
#31626=DIRECTION('',(-0.497542812164539,-0.497542812164539,-0.710564775461607));
#31627=DIRECTION('',(-0.497542812164545,0.497542812164519,-0.710564775461617));
#31628=DIRECTION('',(0.,1.,0.));
#31629=DIRECTION('',(0.497542812164545,0.497542812164522,0.710564775461615));
#31630=DIRECTION('center_axis',(0.24184476264798,0.707106781186533,-0.664463024388688));
#31631=DIRECTION('ref_axis',(-0.939692620785908,0.,-0.342020143325669));
#31632=DIRECTION('',(-0.939692620785908,0.,-0.342020143325669));
#31633=DIRECTION('',(-0.633687274224651,0.633687274224655,0.443712606279627));
#31634=DIRECTION('',(0.939692620785908,0.,0.342020143325669));
#31635=DIRECTION('center_axis',(0.819152044289004,0.,0.573576436351029));
#31636=DIRECTION('ref_axis',(0.573576436351029,0.,-0.819152044289004));
#31637=DIRECTION('',(0.,1.,0.));
#31638=DIRECTION('',(-0.497542812164512,0.497542812164512,0.710564775461646));
#31639=DIRECTION('',(-0.497542812164502,-0.497542812164542,0.710564775461631));
#31640=DIRECTION('',(0.,-1.,0.));
#31641=DIRECTION('',(0.497542812164501,-0.497542812164543,-0.710564775461631));
#31642=DIRECTION('center_axis',(0.241844762647986,-0.707106781186534,0.664463024388685));
#31643=DIRECTION('ref_axis',(0.939692620785905,0.,-0.342020143325678));
#31644=DIRECTION('',(-0.939692620785905,0.,0.342020143325678));
#31645=DIRECTION('',(0.633687274224652,0.633687274224654,0.443712606279627));
#31646=DIRECTION('',(0.939692620785905,0.,-0.342020143325678));
#31647=DIRECTION('center_axis',(-0.342020143325678,0.,-0.939692620785905));
#31648=DIRECTION('ref_axis',(-0.939692620785905,0.,0.342020143325678));
#31649=DIRECTION('',(0.939692620785905,0.,-0.342020143325678));
#31650=DIRECTION('',(0.,1.,0.));
#31651=DIRECTION('center_axis',(0.241844762647986,0.707106781186536,0.664463024388684));
#31652=DIRECTION('ref_axis',(0.939692620785905,0.,-0.342020143325678));
#31653=DIRECTION('',(-0.63368727422465,0.63368727422465,-0.443712606279636));
#31654=DIRECTION('',(-0.939692620785905,0.,0.342020143325678));
#31655=DIRECTION('',(-0.633687274224657,0.633687274224651,-0.443712606279624));
#31656=DIRECTION('center_axis',(0.382683432365109,0.,-0.923879532511279));
#31657=DIRECTION('ref_axis',(-0.923879532511279,0.,-0.382683432365109));
#31658=DIRECTION('',(0.862856209461003,0.357406744336612,0.357406744336608));
#31659=DIRECTION('',(0.,-1.,0.));
#31660=DIRECTION('',(-0.862856209461003,0.357406744336612,-0.357406744336608));
#31661=DIRECTION('',(0.,1.,0.));
#31662=DIRECTION('center_axis',(0.,0.,1.));
#31663=DIRECTION('ref_axis',(1.,0.,0.));
#31664=DIRECTION('',(1.,0.,0.));
#31665=DIRECTION('',(0.,-1.,0.));
#31666=DIRECTION('',(-1.,0.,0.));
#31667=DIRECTION('center_axis',(0.,0.,-1.));
#31668=DIRECTION('ref_axis',(1.,0.,0.));
#31669=DIRECTION('center_axis',(0.,-0.707106781186544,-0.707106781186551));
#31670=DIRECTION('ref_axis',(-1.,0.,0.));
#31671=DIRECTION('',(0.577350269189628,-0.577350269189628,0.577350269189622));
#31672=DIRECTION('',(1.,0.,0.));
#31673=DIRECTION('',(-0.577350269189628,-0.577350269189628,0.577350269189622));
#31674=DIRECTION('',(-0.862856209461003,-0.357406744336612,0.357406744336608));
#31675=DIRECTION('center_axis',(-0.923879532511285,0.,-0.382683432365094));
#31676=DIRECTION('ref_axis',(-0.382683432365094,0.,0.923879532511285));
#31677=DIRECTION('',(0.357406744336596,-0.357406744336596,-0.862856209461014));
#31678=DIRECTION('',(0.,-1.,0.));
#31679=DIRECTION('',(-0.357406744336596,-0.357406744336596,0.862856209461014));
#31680=DIRECTION('',(-0.357406744336596,0.357406744336596,0.862856209461014));
#31681=DIRECTION('',(0.,1.,0.));
#31682=DIRECTION('',(0.357406744336596,0.357406744336596,-0.862856209461014));
#31683=DIRECTION('center_axis',(-0.707106781186544,0.,-0.707106781186551));
#31684=DIRECTION('ref_axis',(-0.707106781186551,0.,0.707106781186544));
#31685=DIRECTION('',(0.577350269189628,-0.577350269189628,-0.577350269189622));
#31686=DIRECTION('',(0.,1.,0.));
#31687=DIRECTION('center_axis',(0.,0.923879532511285,-0.382683432365094));
#31688=DIRECTION('ref_axis',(0.,0.382683432365094,0.923879532511285));
#31689=DIRECTION('',(0.357406744336596,0.357406744336596,0.862856209461014));
#31690=DIRECTION('',(1.,0.,0.));
#31691=DIRECTION('',(0.357406744336596,-0.357406744336596,-0.862856209461014));
#31692=DIRECTION('',(-0.67859834454585,-0.281084637714822,-0.678598344545844));
#31693=DIRECTION('',(-1.,0.,0.));
#31694=DIRECTION('center_axis',(-0.707106781186548,0.707106781186548,0.));
#31695=DIRECTION('ref_axis',(0.,0.,1.));
#31696=DIRECTION('',(0.,0.,1.));
#31697=DIRECTION('',(-0.357406744336592,-0.357406744336592,-0.862856209461018));
#31698=DIRECTION('',(-0.357406744336592,-0.357406744336592,0.862856209461018));
#31699=DIRECTION('',(0.,0.,-1.));
#31700=DIRECTION('center_axis',(-0.382683432365109,0.,-0.923879532511279));
#31701=DIRECTION('ref_axis',(-0.923879532511279,0.,0.382683432365109));
#31702=DIRECTION('',(0.862856209461003,-0.357406744336612,-0.357406744336608));
#31703=DIRECTION('center_axis',(0.923879532511288,0.,0.382683432365088));
#31704=DIRECTION('ref_axis',(0.382683432365088,0.,-0.923879532511288));
#31705=DIRECTION('',(-0.357406744336592,-0.357406744336592,0.862856209461018));
#31706=DIRECTION('',(0.,-1.,0.));
#31707=DIRECTION('',(0.357406744336592,-0.357406744336592,-0.862856209461018));
#31708=DIRECTION('',(0.357406744336592,0.357406744336592,-0.862856209461018));
#31709=DIRECTION('',(0.,1.,0.));
#31710=DIRECTION('',(-0.357406744336592,0.357406744336592,0.862856209461018));
#31711=DIRECTION('center_axis',(0.,0.923879532511288,0.382683432365088));
#31712=DIRECTION('ref_axis',(0.,-0.382683432365088,0.923879532511288));
#31713=DIRECTION('',(-0.357406744336592,0.357406744336592,-0.862856209461018));
#31714=DIRECTION('',(-1.,0.,0.));
#31715=DIRECTION('',(-0.357406744336592,0.357406744336592,-0.862856209461018));
#31716=DIRECTION('',(1.,0.,0.));
#31717=DIRECTION('center_axis',(0.707106781186548,0.707106781186548,0.));
#31718=DIRECTION('ref_axis',(0.,0.,-1.));
#31719=DIRECTION('',(0.,0.,-1.));
#31720=DIRECTION('',(0.497542812164509,-0.497542812164509,0.71056477546165));
#31721=DIRECTION('',(0.633687274224649,-0.633687274224649,-0.443712606279638));
#31722=DIRECTION('',(0.,0.,1.));
#31723=DIRECTION('center_axis',(1.,0.,0.));
#31724=DIRECTION('ref_axis',(0.,1.,0.));
#31725=DIRECTION('',(0.,0.,1.));
#31726=DIRECTION('',(0.,-1.,0.));
#31727=DIRECTION('center_axis',(0.819152044289009,0.,0.573576436351022));
#31728=DIRECTION('ref_axis',(0.573576436351022,0.,-0.819152044289009));
#31729=DIRECTION('',(0.497542812164507,0.497542812164507,-0.710564775461652));
#31730=DIRECTION('',(0.,1.,0.));
#31731=DIRECTION('',(-0.497542812164507,0.497542812164507,0.710564775461652));
#31732=DIRECTION('',(-0.497542812164506,-0.49754281216451,0.710564775461651));
#31733=DIRECTION('',(0.,-1.,0.));
#31734=DIRECTION('',(0.497542812164493,-0.497542812164548,-0.710564775461633));
#31735=DIRECTION('center_axis',(0.241844762647974,0.70710678118657,0.664463024388651));
#31736=DIRECTION('ref_axis',(0.939692620785905,0.,-0.342020143325678));
#31737=DIRECTION('',(-0.633687274224631,0.633687274224631,-0.443712606279689));
#31738=DIRECTION('',(-0.939692620785905,0.,0.342020143325678));
#31739=DIRECTION('',(-0.633687274224635,0.633687274224637,-0.443712606279675));
#31740=DIRECTION('',(0.939692620785905,0.,-0.342020143325678));
#31741=DIRECTION('center_axis',(0.707106781186548,0.707106781186548,0.));
#31742=DIRECTION('ref_axis',(0.,0.,-1.));
#31743=DIRECTION('',(0.,0.,-1.));
#31744=DIRECTION('',(0.497542812164534,-0.497542812164534,0.710564775461614));
#31745=DIRECTION('',(0.633687274224667,-0.633687274224667,-0.443712606279587));
#31746=DIRECTION('',(0.,0.,1.));
#31747=DIRECTION('center_axis',(1.,0.,0.));
#31748=DIRECTION('ref_axis',(0.,1.,0.));
#31749=DIRECTION('',(0.,0.,1.));
#31750=DIRECTION('',(0.,-1.,0.));
#31751=DIRECTION('center_axis',(0.81915204428898,0.,-0.573576436351063));
#31752=DIRECTION('ref_axis',(-0.573576436351063,0.,-0.81915204428898));
#31753=DIRECTION('',(-0.497542812164534,-0.497542812164534,-0.710564775461614));
#31754=DIRECTION('',(-0.497542812164537,0.497542812164526,-0.710564775461618));
#31755=DIRECTION('',(0.,1.,0.));
#31756=DIRECTION('',(0.497542812164526,0.49754281216456,0.710564775461602));
#31757=DIRECTION('center_axis',(0.241844762647991,0.707106781186501,-0.664463024388718));
#31758=DIRECTION('ref_axis',(-0.939692620785908,0.,-0.342020143325669));
#31759=DIRECTION('',(-0.939692620785908,0.,-0.342020143325669));
#31760=DIRECTION('',(-0.633687274224651,0.633687274224655,0.443712606279627));
#31761=DIRECTION('',(0.939692620785908,0.,0.342020143325669));
#31762=DIRECTION('center_axis',(0.819152044289004,0.,0.573576436351029));
#31763=DIRECTION('ref_axis',(0.573576436351029,0.,-0.819152044289004));
#31764=DIRECTION('',(0.497542812164512,0.497542812164512,-0.710564775461646));
#31765=DIRECTION('',(0.,1.,0.));
#31766=DIRECTION('',(-0.497542812164512,0.497542812164512,0.710564775461646));
#31767=DIRECTION('',(-0.497542812164501,-0.497542812164543,0.710564775461631));
#31768=DIRECTION('',(0.,-1.,0.));
#31769=DIRECTION('',(0.49754281216449,-0.497542812164577,-0.710564775461615));
#31770=DIRECTION('center_axis',(0.241844762647986,0.707106781186534,0.664463024388685));
#31771=DIRECTION('ref_axis',(0.939692620785905,0.,-0.342020143325678));
#31772=DIRECTION('',(-0.63368727422465,0.63368727422465,-0.443712606279634));
#31773=DIRECTION('',(-0.939692620785905,0.,0.342020143325678));
#31774=DIRECTION('',(-0.633687274224652,0.633687274224654,-0.443712606279627));
#31775=DIRECTION('',(0.939692620785905,0.,-0.342020143325678));
#31776=DIRECTION('center_axis',(0.707106781186548,0.707106781186548,0.));
#31777=DIRECTION('ref_axis',(0.,0.,-1.));
#31778=DIRECTION('',(0.,0.,-1.));
#31779=DIRECTION('',(0.497542812164509,-0.497542812164509,0.71056477546165));
#31780=DIRECTION('',(0.633687274224631,-0.633687274224631,-0.443712606279689));
#31781=DIRECTION('',(0.,0.,1.));
#31782=DIRECTION('center_axis',(1.,0.,0.));
#31783=DIRECTION('ref_axis',(0.,1.,0.));
#31784=DIRECTION('',(0.,0.,1.));
#31785=DIRECTION('',(0.,-1.,0.));
#31786=DIRECTION('center_axis',(0.819152044289007,0.,-0.573576436351024));
#31787=DIRECTION('ref_axis',(-0.573576436351024,0.,-0.819152044289007));
#31788=DIRECTION('',(-0.497542812164509,-0.497542812164509,-0.71056477546165));
#31789=DIRECTION('',(-0.497542812164497,0.497542812164543,-0.710564775461634));
#31790=DIRECTION('',(0.,1.,0.));
#31791=DIRECTION('',(0.497542812164509,0.497542812164509,0.71056477546165));
#31792=DIRECTION('center_axis',(0.241844762647974,0.70710678118657,-0.664463024388651));
#31793=DIRECTION('ref_axis',(-0.939692620785905,0.,-0.342020143325678));
#31794=DIRECTION('',(-0.939692620785905,0.,-0.342020143325678));
#31795=DIRECTION('',(-0.633687274224634,0.633687274224638,0.443712606279675));
#31796=DIRECTION('',(0.939692620785905,0.,0.342020143325678));
#31797=DIRECTION('center_axis',(0.819152044289007,0.,0.573576436351024));
#31798=DIRECTION('ref_axis',(0.573576436351024,0.,-0.819152044289007));
#31799=DIRECTION('',(0.497542812164509,0.497542812164509,-0.71056477546165));
#31800=DIRECTION('',(0.,1.,0.));
#31801=DIRECTION('',(-0.497542812164509,0.497542812164509,0.71056477546165));
#31802=DIRECTION('',(-0.497542812164497,-0.497542812164545,0.710564775461633));
#31803=DIRECTION('',(0.,-1.,0.));
#31804=DIRECTION('',(0.497542812164498,-0.497542812164542,-0.710564775461634));
#31805=DIRECTION('center_axis',(0.241844762647986,0.707106781186536,0.664463024388684));
#31806=DIRECTION('ref_axis',(0.939692620785905,0.,-0.342020143325678));
#31807=DIRECTION('',(-0.63368727422465,0.63368727422465,-0.443712606279636));
#31808=DIRECTION('',(-0.939692620785905,0.,0.342020143325678));
#31809=DIRECTION('',(-0.633687274224652,0.633687274224654,-0.443712606279627));
#31810=DIRECTION('',(0.939692620785905,0.,-0.342020143325678));
#31811=DIRECTION('center_axis',(0.707106781186548,0.707106781186548,0.));
#31812=DIRECTION('ref_axis',(0.,0.,-1.));
#31813=DIRECTION('',(0.,0.,-1.));
#31814=DIRECTION('',(0.497542812164515,-0.497542812164515,0.710564775461641));
#31815=DIRECTION('',(0.633687274224629,-0.633687274224629,-0.443712606279694));
#31816=DIRECTION('',(0.,0.,1.));
#31817=DIRECTION('center_axis',(1.,0.,0.));
#31818=DIRECTION('ref_axis',(0.,1.,0.));
#31819=DIRECTION('',(0.,0.,1.));
#31820=DIRECTION('',(0.,-1.,0.));
#31821=DIRECTION('center_axis',(0.819152044289001,0.,-0.573576436351034));
#31822=DIRECTION('ref_axis',(-0.573576436351034,0.,-0.819152044289001));
#31823=DIRECTION('',(-0.497542812164515,-0.497542812164515,-0.710564775461641));
#31824=DIRECTION('',(-0.49754281216452,0.497542812164499,-0.710564775461649));
#31825=DIRECTION('',(0.,1.,0.));
#31826=DIRECTION('',(0.49754281216452,0.497542812164498,0.710564775461649));
#31827=DIRECTION('center_axis',(0.241844762647973,0.707106781186574,-0.664463024388648));
#31828=DIRECTION('ref_axis',(-0.939692620785905,0.,-0.342020143325678));
#31829=DIRECTION('',(-0.939692620785905,0.,-0.342020143325678));
#31830=DIRECTION('',(-0.633687274224617,0.633687274224621,0.443712606279724));
#31831=DIRECTION('',(0.939692620785905,0.,0.342020143325678));
#31832=DIRECTION('center_axis',(0.819152044289033,0.,0.573576436350987));
#31833=DIRECTION('ref_axis',(0.573576436350987,0.,-0.819152044289033));
#31834=DIRECTION('',(0.497542812164485,0.497542812164485,-0.710564775461684));
#31835=DIRECTION('',(0.,1.,0.));
#31836=DIRECTION('',(-0.497542812164485,0.497542812164485,0.710564775461684));
#31837=DIRECTION('',(-0.497542812164469,-0.497542812164533,0.710564775461661));
#31838=DIRECTION('',(0.,-1.,0.));
#31839=DIRECTION('',(0.497542812164469,-0.497542812164533,-0.710564775461661));
#31840=DIRECTION('center_axis',(0.241844762647974,0.70710678118657,0.664463024388651));
#31841=DIRECTION('ref_axis',(0.939692620785905,0.,-0.342020143325678));
#31842=DIRECTION('',(-0.633687274224631,0.633687274224631,-0.443712606279689));
#31843=DIRECTION('',(-0.939692620785905,0.,0.342020143325678));
#31844=DIRECTION('',(-0.63368727422464,0.633687274224634,-0.443712606279673));
#31845=DIRECTION('',(0.939692620785905,0.,-0.342020143325678));
#31846=DIRECTION('center_axis',(0.707106781186548,0.707106781186548,0.));
#31847=DIRECTION('ref_axis',(0.,0.,-1.));
#31848=DIRECTION('',(0.,0.,-1.));
#31849=DIRECTION('',(0.497542812164539,-0.497542812164539,0.710564775461607));
#31850=DIRECTION('',(0.63368727422465,-0.63368727422465,-0.443712606279635));
#31851=DIRECTION('',(0.,0.,1.));
#31852=DIRECTION('center_axis',(1.,0.,0.));
#31853=DIRECTION('ref_axis',(0.,1.,0.));
#31854=DIRECTION('',(0.,0.,1.));
#31855=DIRECTION('',(0.,-1.,0.));
#31856=DIRECTION('center_axis',(0.819152044288975,0.,-0.573576436351071));
#31857=DIRECTION('ref_axis',(-0.573576436351071,0.,-0.819152044288975));
#31858=DIRECTION('',(-0.497542812164539,-0.497542812164539,-0.710564775461607));
#31859=DIRECTION('',(-0.497542812164545,0.497542812164521,-0.710564775461616));
#31860=DIRECTION('',(0.,1.,0.));
#31861=DIRECTION('',(0.497542812164545,0.497542812164522,0.710564775461615));
#31862=DIRECTION('center_axis',(0.24184476264798,0.707106781186533,-0.664463024388688));
#31863=DIRECTION('ref_axis',(-0.939692620785908,0.,-0.342020143325669));
#31864=DIRECTION('',(-0.939692620785908,0.,-0.342020143325669));
#31865=DIRECTION('',(-0.633687274224651,0.633687274224655,0.443712606279627));
#31866=DIRECTION('',(0.939692620785908,0.,0.342020143325669));
#31867=DIRECTION('center_axis',(0.819152044289007,0.,0.573576436351024));
#31868=DIRECTION('ref_axis',(0.573576436351024,0.,-0.819152044289007));
#31869=DIRECTION('',(0.497542812164509,0.497542812164509,-0.71056477546165));
#31870=DIRECTION('',(0.,1.,0.));
#31871=DIRECTION('',(-0.497542812164509,0.497542812164509,0.71056477546165));
#31872=DIRECTION('',(-0.497542812164497,-0.497542812164545,0.710564775461633));
#31873=DIRECTION('',(0.,-1.,0.));
#31874=DIRECTION('',(0.497542812164496,-0.497542812164546,-0.710564775461632));
#31875=DIRECTION('center_axis',(-0.342020143325678,0.,-0.939692620785905));
#31876=DIRECTION('ref_axis',(-0.939692620785905,0.,0.342020143325678));
#31877=DIRECTION('',(0.939692620785905,0.,-0.342020143325678));
#31878=DIRECTION('',(0.,1.,0.));
#31879=DIRECTION('',(-0.939692620785905,0.,0.342020143325678));
#31880=DIRECTION('center_axis',(0.241844762647986,0.707106781186536,0.664463024388684));
#31881=DIRECTION('ref_axis',(0.939692620785905,0.,-0.342020143325678));
#31882=DIRECTION('',(-0.63368727422465,0.63368727422465,-0.443712606279636));
#31883=DIRECTION('',(-0.939692620785905,0.,0.342020143325678));
#31884=DIRECTION('',(-0.633687274224652,0.633687274224654,-0.443712606279627));
#31885=DIRECTION('center_axis',(0.707106781186548,0.707106781186548,0.));
#31886=DIRECTION('ref_axis',(0.,0.,-1.));
#31887=DIRECTION('',(0.,0.,1.));
#31888=DIRECTION('',(0.,0.,-1.));
#31889=DIRECTION('center_axis',(0.70710678118655,0.707106781186545,0.));
#31890=DIRECTION('ref_axis',(0.,0.,-1.));
#31891=DIRECTION('',(0.,0.,1.));
#31892=DIRECTION('',(0.,0.,-1.));
#31893=DIRECTION('center_axis',(-1.,0.,0.));
#31894=DIRECTION('ref_axis',(0.,0.,1.));
#31895=DIRECTION('',(0.,1.,0.));
#31896=DIRECTION('',(0.,0.,1.));
#31897=DIRECTION('center_axis',(-0.342020143325669,0.,0.939692620785908));
#31898=DIRECTION('ref_axis',(0.939692620785908,0.,0.342020143325669));
#31899=DIRECTION('',(0.939692620785908,0.,0.342020143325669));
#31900=DIRECTION('center_axis',(0.70710678118655,0.707106781186545,0.));
#31901=DIRECTION('ref_axis',(0.,0.,-1.));
#31902=DIRECTION('',(0.,0.,1.));
#31903=DIRECTION('',(0.,0.,-1.));
#31904=DIRECTION('center_axis',(-0.342020143325678,0.,-0.939692620785905));
#31905=DIRECTION('ref_axis',(-0.939692620785905,0.,0.342020143325678));
#31906=DIRECTION('',(0.,1.,0.));
#31907=DIRECTION('',(-0.939692620785905,0.,0.342020143325678));
#31908=DIRECTION('center_axis',(-1.,0.,0.));
#31909=DIRECTION('ref_axis',(0.,0.,1.));
#31910=DIRECTION('',(0.,1.,0.));
#31911=DIRECTION('',(0.,0.,1.));
#31912=DIRECTION('center_axis',(-0.342020143325678,0.,0.939692620785905));
#31913=DIRECTION('ref_axis',(0.939692620785905,0.,0.342020143325678));
#31914=DIRECTION('',(0.939692620785905,0.,0.342020143325678));
#31915=DIRECTION('center_axis',(0.70710678118655,0.707106781186545,0.));
#31916=DIRECTION('ref_axis',(0.,0.,-1.));
#31917=DIRECTION('',(0.,0.,1.));
#31918=DIRECTION('',(0.,0.,-1.));
#31919=DIRECTION('center_axis',(-0.342020143325678,0.,-0.939692620785905));
#31920=DIRECTION('ref_axis',(-0.939692620785905,0.,0.342020143325678));
#31921=DIRECTION('',(0.,1.,0.));
#31922=DIRECTION('',(-0.939692620785905,0.,0.342020143325678));
#31923=DIRECTION('center_axis',(-1.,0.,0.));
#31924=DIRECTION('ref_axis',(0.,0.,1.));
#31925=DIRECTION('',(0.,0.,1.));
#31926=DIRECTION('center_axis',(0.,1.,0.));
#31927=DIRECTION('ref_axis',(-1.,0.,0.));
#31928=DIRECTION('',(0.,0.,1.));
#31929=DIRECTION('',(0.939692620785905,0.,0.342020143325678));
#31930=DIRECTION('',(0.,0.,1.));
#31931=DIRECTION('',(-0.939692620785905,0.,0.342020143325678));
#31932=DIRECTION('',(0.,0.,1.));
#31933=DIRECTION('',(0.939692620785905,0.,0.342020143325678));
#31934=DIRECTION('',(0.,0.,1.));
#31935=DIRECTION('',(-0.939692620785905,0.,0.342020143325678));
#31936=DIRECTION('',(0.,0.,1.));
#31937=DIRECTION('',(0.939692620785908,0.,0.342020143325669));
#31938=DIRECTION('',(0.,0.,1.));
#31939=DIRECTION('',(-0.939692620785905,0.,0.342020143325678));
#31940=DIRECTION('',(0.,0.,1.));
#31941=DIRECTION('',(0.939692620785905,0.,0.342020143325678));
#31942=DIRECTION('',(0.,0.,1.));
#31943=DIRECTION('',(-0.939692620785905,0.,0.342020143325678));
#31944=DIRECTION('',(0.,0.,1.));
#31945=DIRECTION('',(0.939692620785905,0.,0.342020143325678));
#31946=DIRECTION('',(0.,0.,1.));
#31947=DIRECTION('',(-0.939692620785905,0.,0.342020143325678));
#31948=DIRECTION('',(0.,0.,1.));
#31949=DIRECTION('',(0.939692620785905,0.,0.342020143325678));
#31950=DIRECTION('',(0.,0.,1.));
#31951=DIRECTION('',(-0.939692620785908,0.,0.342020143325669));
#31952=DIRECTION('',(0.,0.,1.));
#31953=DIRECTION('',(0.939692620785908,0.,0.342020143325669));
#31954=DIRECTION('',(0.,0.,1.));
#31955=DIRECTION('',(-0.939692620785908,0.,0.342020143325669));
#31956=DIRECTION('',(0.,0.,1.));
#31957=DIRECTION('',(0.,0.,1.));
#31958=DIRECTION('',(0.,0.,1.));
#31959=DIRECTION('',(-0.939692620785908,0.,0.342020143325669));
#31960=DIRECTION('',(0.,0.,1.));
#31961=DIRECTION('',(0.939692620785908,0.,0.342020143325669));
#31962=DIRECTION('',(0.,0.,1.));
#31963=DIRECTION('',(-0.939692620785908,0.,0.342020143325669));
#31964=DIRECTION('',(0.,0.,1.));
#31965=DIRECTION('',(0.939692620785908,0.,0.342020143325669));
#31966=DIRECTION('',(0.,0.,1.));
#31967=DIRECTION('',(-0.939692620785908,0.,0.342020143325669));
#31968=DIRECTION('',(0.,0.,1.));
#31969=DIRECTION('',(0.939692620785908,0.,0.342020143325669));
#31970=DIRECTION('',(0.,0.,1.));
#31971=DIRECTION('',(-0.939692620785908,0.,0.342020143325669));
#31972=DIRECTION('',(0.,0.,1.));
#31973=DIRECTION('',(0.939692620785908,0.,0.342020143325669));
#31974=DIRECTION('',(0.,0.,1.));
#31975=DIRECTION('',(-0.939692620785908,0.,0.342020143325669));
#31976=DIRECTION('',(0.,0.,1.));
#31977=DIRECTION('',(0.939692620785908,0.,0.342020143325669));
#31978=DIRECTION('',(0.,0.,1.));
#31979=DIRECTION('',(-0.939692620785908,0.,0.342020143325669));
#31980=DIRECTION('',(0.,0.,1.));
#31981=DIRECTION('',(0.939692620785908,0.,0.342020143325669));
#31982=DIRECTION('',(0.,0.,1.));
#31983=DIRECTION('',(-0.939692620785908,0.,0.342020143325669));
#31984=DIRECTION('',(0.,0.,1.));
#31985=DIRECTION('',(0.,0.,1.));
#31986=DIRECTION('',(0.,0.,1.));
#31987=DIRECTION('',(0.,0.,1.));
#31988=DIRECTION('',(0.939692620785908,0.,0.342020143325669));
#31989=DIRECTION('',(0.,0.,1.));
#31990=DIRECTION('',(0.,0.,1.));
#31991=DIRECTION('',(0.,0.,1.));
#31992=DIRECTION('',(0.,0.,1.));
#31993=DIRECTION('',(0.939692620785908,0.,0.342020143325669));
#31994=DIRECTION('',(0.,0.,1.));
#31995=DIRECTION('',(-0.939692620785908,0.,0.342020143325669));
#31996=DIRECTION('',(0.,0.,1.));
#31997=DIRECTION('',(0.939692620785905,0.,0.342020143325678));
#31998=DIRECTION('',(0.,0.,1.));
#31999=DIRECTION('',(0.,0.,1.));
#32000=DIRECTION('',(0.,0.,1.));
#32001=DIRECTION('',(0.,0.,1.));
#32002=DIRECTION('',(0.,0.,1.));
#32003=DIRECTION('center_axis',(0.70710678118655,0.707106781186545,0.));
#32004=DIRECTION('ref_axis',(0.,0.,-1.));
#32005=DIRECTION('',(0.,0.,-1.));
#32006=DIRECTION('center_axis',(-1.,0.,0.));
#32007=DIRECTION('ref_axis',(0.,0.,1.));
#32008=DIRECTION('',(0.,1.,0.));
#32009=DIRECTION('',(0.,0.,1.));
#32010=DIRECTION('center_axis',(-0.342020143325669,0.,0.939692620785908));
#32011=DIRECTION('ref_axis',(0.939692620785908,0.,0.342020143325669));
#32012=DIRECTION('',(0.939692620785908,0.,0.342020143325669));
#32013=DIRECTION('center_axis',(0.70710678118655,0.707106781186545,0.));
#32014=DIRECTION('ref_axis',(0.,0.,-1.));
#32015=DIRECTION('',(0.,0.,-1.));
#32016=DIRECTION('center_axis',(-0.342020143325678,0.,-0.939692620785905));
#32017=DIRECTION('ref_axis',(-0.939692620785905,0.,0.342020143325678));
#32018=DIRECTION('',(0.,1.,0.));
#32019=DIRECTION('',(-0.939692620785905,0.,0.342020143325678));
#32020=DIRECTION('center_axis',(-1.,0.,0.));
#32021=DIRECTION('ref_axis',(0.,0.,1.));
#32022=DIRECTION('',(0.,1.,0.));
#32023=DIRECTION('',(0.,0.,1.));
#32024=DIRECTION('center_axis',(-0.342020143325678,0.,0.939692620785905));
#32025=DIRECTION('ref_axis',(0.939692620785905,0.,0.342020143325678));
#32026=DIRECTION('',(0.939692620785905,0.,0.342020143325678));
#32027=DIRECTION('center_axis',(0.70710678118655,0.707106781186545,0.));
#32028=DIRECTION('ref_axis',(0.,0.,-1.));
#32029=DIRECTION('',(0.,0.,-1.));
#32030=DIRECTION('center_axis',(-0.342020143325678,0.,-0.939692620785905));
#32031=DIRECTION('ref_axis',(-0.939692620785905,0.,0.342020143325678));
#32032=DIRECTION('',(0.,1.,0.));
#32033=DIRECTION('',(-0.939692620785905,0.,0.342020143325678));
#32034=DIRECTION('center_axis',(-1.,0.,0.));
#32035=DIRECTION('ref_axis',(0.,0.,1.));
#32036=DIRECTION('',(0.,1.,0.));
#32037=DIRECTION('',(0.,0.,1.));
#32038=DIRECTION('center_axis',(-0.342020143325678,0.,0.939692620785905));
#32039=DIRECTION('ref_axis',(0.939692620785905,0.,0.342020143325678));
#32040=DIRECTION('',(0.939692620785905,0.,0.342020143325678));
#32041=DIRECTION('center_axis',(0.70710678118655,0.707106781186545,0.));
#32042=DIRECTION('ref_axis',(0.,0.,-1.));
#32043=DIRECTION('',(0.,0.,-1.));
#32044=DIRECTION('center_axis',(-0.342020143325678,0.,-0.939692620785905));
#32045=DIRECTION('ref_axis',(-0.939692620785905,0.,0.342020143325678));
#32046=DIRECTION('',(0.,1.,0.));
#32047=DIRECTION('',(-0.939692620785905,0.,0.342020143325678));
#32048=DIRECTION('center_axis',(-1.,0.,0.));
#32049=DIRECTION('ref_axis',(0.,0.,1.));
#32050=DIRECTION('',(0.,1.,0.));
#32051=DIRECTION('',(0.,0.,1.));
#32052=DIRECTION('center_axis',(-0.342020143325669,0.,0.939692620785908));
#32053=DIRECTION('ref_axis',(0.939692620785908,0.,0.342020143325669));
#32054=DIRECTION('',(0.939692620785908,0.,0.342020143325669));
#32055=DIRECTION('center_axis',(0.70710678118655,0.707106781186545,0.));
#32056=DIRECTION('ref_axis',(0.,0.,-1.));
#32057=DIRECTION('',(-0.633687274224609,0.633687274224613,0.443712606279746));
#32058=DIRECTION('',(0.,0.,-1.));
#32059=DIRECTION('center_axis',(-0.342020143325678,0.,-0.939692620785905));
#32060=DIRECTION('ref_axis',(-0.939692620785905,0.,0.342020143325678));
#32061=DIRECTION('',(0.,1.,0.));
#32062=DIRECTION('',(-0.939692620785905,0.,0.342020143325678));
#32063=DIRECTION('center_axis',(-1.,0.,0.));
#32064=DIRECTION('ref_axis',(0.,0.,1.));
#32065=DIRECTION('',(0.,1.,0.));
#32066=DIRECTION('',(0.,0.,1.));
#32067=DIRECTION('center_axis',(-0.382683432365118,0.,0.923879532511275));
#32068=DIRECTION('ref_axis',(0.923879532511275,0.,0.382683432365118));
#32069=DIRECTION('',(-0.862856209461002,0.357406744336604,-0.357406744336618));
#32070=DIRECTION('',(0.,-1.,0.));
#32071=DIRECTION('',(0.862856209461002,0.357406744336604,0.357406744336618));
#32072=DIRECTION('',(0.,1.,0.));
#32073=DIRECTION('center_axis',(0.,-0.707106781186561,0.707106781186534));
#32074=DIRECTION('ref_axis',(1.,0.,0.));
#32075=DIRECTION('',(-0.577350269189618,-0.577350269189618,-0.577350269189641));
#32076=DIRECTION('',(-1.,0.,0.));
#32077=DIRECTION('',(0.577350269189618,-0.577350269189618,-0.577350269189641));
#32078=DIRECTION('',(-1.,0.,0.));
#32079=DIRECTION('center_axis',(-0.707106781186561,0.,0.707106781186534));
#32080=DIRECTION('ref_axis',(0.707106781186534,0.,0.707106781186561));
#32081=DIRECTION('',(-0.577350269189618,0.577350269189618,-0.577350269189641));
#32082=DIRECTION('',(0.,1.,0.));
#32083=DIRECTION('center_axis',(-0.923879532511288,0.,0.382683432365088));
#32084=DIRECTION('ref_axis',(0.382683432365088,0.,0.923879532511288));
#32085=DIRECTION('',(0.357406744336592,0.357406744336592,0.862856209461018));
#32086=DIRECTION('',(0.,-1.,0.));
#32087=DIRECTION('',(0.357406744336592,-0.357406744336592,0.862856209461018));
#32088=DIRECTION('center_axis',(0.,-0.923879532511288,0.382683432365088));
#32089=DIRECTION('ref_axis',(0.,-0.382683432365088,-0.923879532511288));
#32090=DIRECTION('',(0.357406744336592,-0.357406744336592,-0.862856209461018));
#32091=DIRECTION('',(1.,0.,0.));
#32092=DIRECTION('',(0.357406744336592,0.357406744336592,0.862856209461018));
#32093=DIRECTION('center_axis',(-0.707106781186548,-0.707106781186548,0.));
#32094=DIRECTION('ref_axis',(0.,0.,1.));
#32095=DIRECTION('',(-0.357406744336596,0.357406744336596,-0.862856209461014));
#32096=DIRECTION('',(0.,0.,1.));
#32097=DIRECTION('',(0.,0.,-1.));
#32098=DIRECTION('center_axis',(0.819152044289007,0.,-0.573576436351024));
#32099=DIRECTION('ref_axis',(-0.573576436351024,0.,-0.819152044289007));
#32100=DIRECTION('',(-0.497542812164509,-0.497542812164509,-0.71056477546165));
#32101=DIRECTION('',(-0.49754281216452,0.497542812164474,-0.710564775461666));
#32102=DIRECTION('',(0.,1.,0.));
#32103=DIRECTION('',(0.497542812164495,0.497542812164551,0.71056477546163));
#32104=DIRECTION('center_axis',(0.24184476264798,0.707106781186534,-0.664463024388687));
#32105=DIRECTION('ref_axis',(-0.939692620785908,0.,-0.342020143325669));
#32106=DIRECTION('',(-0.939692620785908,0.,-0.342020143325669));
#32107=DIRECTION('',(-0.633687274224651,0.633687274224655,0.443712606279627));
#32108=DIRECTION('center_axis',(0.819152044289004,0.,0.573576436351029));
#32109=DIRECTION('ref_axis',(0.573576436351029,0.,-0.819152044289004));
#32110=DIRECTION('',(0.497542812164512,0.497542812164512,-0.710564775461646));
#32111=DIRECTION('',(0.,1.,0.));
#32112=DIRECTION('',(-0.497542812164512,0.497542812164512,0.710564775461646));
#32113=DIRECTION('',(-0.497542812164499,-0.497542812164549,0.710564775461628));
#32114=DIRECTION('',(0.,-1.,0.));
#32115=DIRECTION('',(0.497542812164488,-0.497542812164584,-0.710564775461611));
#32116=DIRECTION('center_axis',(0.24184476264798,0.707106781186533,0.664463024388688));
#32117=DIRECTION('ref_axis',(0.939692620785908,0.,-0.342020143325669));
#32118=DIRECTION('',(-0.63368727422465,0.63368727422465,-0.443712606279635));
#32119=DIRECTION('',(-0.633687274224657,0.633687274224651,-0.443712606279624));
#32120=DIRECTION('',(0.939692620785908,0.,-0.342020143325669));
#32121=DIRECTION('center_axis',(0.707106781186548,0.707106781186548,0.));
#32122=DIRECTION('ref_axis',(0.,0.,-1.));
#32123=DIRECTION('',(0.,0.,-1.));
#32124=DIRECTION('',(0.497542812164536,-0.497542812164536,0.710564775461612));
#32125=DIRECTION('',(0.633687274224612,-0.633687274224612,-0.443712606279744));
#32126=DIRECTION('center_axis',(1.,0.,0.));
#32127=DIRECTION('ref_axis',(0.,1.,0.));
#32128=DIRECTION('',(0.,0.,1.));
#32129=DIRECTION('',(0.,-1.,0.));
#32130=DIRECTION('center_axis',(0.819152044288978,0.,-0.573576436351066));
#32131=DIRECTION('ref_axis',(-0.573576436351066,0.,-0.819152044288978));
#32132=DIRECTION('',(-0.497542812164536,-0.497542812164536,-0.710564775461612));
#32133=DIRECTION('',(-0.497542812164555,0.497542812164478,-0.710564775461639));
#32134=DIRECTION('',(0.,1.,0.));
#32135=DIRECTION('',(0.497542812164566,0.497542812164443,0.710564775461655));
#32136=DIRECTION('center_axis',(0.241844762647962,0.707106781186606,-0.664463024388618));
#32137=DIRECTION('ref_axis',(-0.939692620785905,0.,-0.342020143325678));
#32138=DIRECTION('',(-0.939692620785905,0.,-0.342020143325678));
#32139=DIRECTION('center_axis',(-0.342020143325678,0.,0.939692620785905));
#32140=DIRECTION('ref_axis',(0.939692620785905,0.,0.342020143325678));
#32141=DIRECTION('',(0.939692620785905,0.,0.342020143325678));
#32142=DIRECTION('center_axis',(0.70710678118655,0.707106781186545,0.));
#32143=DIRECTION('ref_axis',(0.,0.,-1.));
#32144=DIRECTION('',(0.,0.,-1.));
#32145=DIRECTION('center_axis',(-0.342020143325669,0.,-0.939692620785908));
#32146=DIRECTION('ref_axis',(-0.939692620785908,0.,0.342020143325669));
#32147=DIRECTION('',(0.,1.,0.));
#32148=DIRECTION('',(-0.939692620785908,0.,0.342020143325669));
#32149=DIRECTION('center_axis',(-1.,0.,0.));
#32150=DIRECTION('ref_axis',(0.,0.,1.));
#32151=DIRECTION('',(0.,1.,0.));
#32152=DIRECTION('',(0.,0.,1.));
#32153=DIRECTION('center_axis',(-0.342020143325669,0.,0.939692620785908));
#32154=DIRECTION('ref_axis',(0.939692620785908,0.,0.342020143325669));
#32155=DIRECTION('',(0.939692620785908,0.,0.342020143325669));
#32156=DIRECTION('center_axis',(0.70710678118655,0.707106781186545,0.));
#32157=DIRECTION('ref_axis',(0.,0.,-1.));
#32158=DIRECTION('',(0.,0.,-1.));
#32159=DIRECTION('center_axis',(-1.,0.,0.));
#32160=DIRECTION('ref_axis',(0.,0.,1.));
#32161=DIRECTION('',(0.,1.,0.));
#32162=DIRECTION('',(0.,0.,1.));
#32163=DIRECTION('center_axis',(-0.342020143325669,0.,0.939692620785908));
#32164=DIRECTION('ref_axis',(0.939692620785908,0.,0.342020143325669));
#32165=DIRECTION('',(0.939692620785908,0.,0.342020143325669));
#32166=DIRECTION('center_axis',(0.70710678118655,0.707106781186545,0.));
#32167=DIRECTION('ref_axis',(0.,0.,-1.));
#32168=DIRECTION('',(0.,0.,-1.));
#32169=DIRECTION('center_axis',(-0.342020143325669,0.,-0.939692620785908));
#32170=DIRECTION('ref_axis',(-0.939692620785908,0.,0.342020143325669));
#32171=DIRECTION('',(0.,1.,0.));
#32172=DIRECTION('',(-0.939692620785908,0.,0.342020143325669));
#32173=DIRECTION('center_axis',(-1.,0.,0.));
#32174=DIRECTION('ref_axis',(0.,0.,1.));
#32175=DIRECTION('',(0.,1.,0.));
#32176=DIRECTION('',(0.,0.,1.));
#32177=DIRECTION('center_axis',(-0.342020143325669,0.,0.939692620785908));
#32178=DIRECTION('ref_axis',(0.939692620785908,0.,0.342020143325669));
#32179=DIRECTION('',(0.939692620785908,0.,0.342020143325669));
#32180=DIRECTION('center_axis',(0.24184476264798,0.707106781186535,-0.664463024388687));
#32181=DIRECTION('ref_axis',(-0.939692620785908,0.,-0.342020143325669));
#32182=DIRECTION('',(-0.633687274224651,0.633687274224655,0.443712606279627));
#32183=DIRECTION('center_axis',(0.70710678118655,0.707106781186545,0.));
#32184=DIRECTION('ref_axis',(0.,0.,-1.));
#32185=DIRECTION('',(0.,0.,-1.));
#32186=DIRECTION('center_axis',(-0.342020143325669,0.,-0.939692620785908));
#32187=DIRECTION('ref_axis',(-0.939692620785908,0.,0.342020143325669));
#32188=DIRECTION('',(0.,1.,0.));
#32189=DIRECTION('',(-0.939692620785908,0.,0.342020143325669));
#32190=DIRECTION('center_axis',(-1.,0.,0.));
#32191=DIRECTION('ref_axis',(0.,0.,1.));
#32192=DIRECTION('',(0.,0.,1.));
#32193=DIRECTION('center_axis',(0.70710678118655,0.707106781186545,0.));
#32194=DIRECTION('ref_axis',(0.,0.,-1.));
#32195=DIRECTION('',(0.,0.,-1.));
#32196=DIRECTION('center_axis',(-1.,0.,0.));
#32197=DIRECTION('ref_axis',(0.,0.,1.));
#32198=DIRECTION('',(0.,1.,0.));
#32199=DIRECTION('',(0.,0.,1.));
#32200=DIRECTION('center_axis',(-0.342020143325669,0.,0.939692620785908));
#32201=DIRECTION('ref_axis',(0.939692620785908,0.,0.342020143325669));
#32202=DIRECTION('',(0.939692620785908,0.,0.342020143325669));
#32203=DIRECTION('center_axis',(0.70710678118655,0.707106781186545,0.));
#32204=DIRECTION('ref_axis',(0.,0.,-1.));
#32205=DIRECTION('',(0.,0.,-1.));
#32206=DIRECTION('center_axis',(-0.342020143325669,0.,-0.939692620785908));
#32207=DIRECTION('ref_axis',(-0.939692620785908,0.,0.342020143325669));
#32208=DIRECTION('',(0.,1.,0.));
#32209=DIRECTION('',(-0.939692620785908,0.,0.342020143325669));
#32210=DIRECTION('center_axis',(-1.,0.,0.));
#32211=DIRECTION('ref_axis',(0.,0.,1.));
#32212=DIRECTION('',(0.,0.,1.));
#32213=DIRECTION('center_axis',(0.70710678118655,0.707106781186545,0.));
#32214=DIRECTION('ref_axis',(0.,0.,-1.));
#32215=DIRECTION('',(0.,0.,-1.));
#32216=DIRECTION('center_axis',(-1.,0.,0.));
#32217=DIRECTION('ref_axis',(0.,0.,1.));
#32218=DIRECTION('',(0.,1.,0.));
#32219=DIRECTION('',(0.,0.,1.));
#32220=DIRECTION('center_axis',(-0.342020143325669,0.,0.939692620785908));
#32221=DIRECTION('ref_axis',(0.939692620785908,0.,0.342020143325669));
#32222=DIRECTION('',(0.939692620785908,0.,0.342020143325669));
#32223=DIRECTION('center_axis',(0.70710678118655,0.707106781186545,0.));
#32224=DIRECTION('ref_axis',(0.,0.,-1.));
#32225=DIRECTION('',(0.,0.,-1.));
#32226=DIRECTION('center_axis',(-0.342020143325669,0.,-0.939692620785908));
#32227=DIRECTION('ref_axis',(-0.939692620785908,0.,0.342020143325669));
#32228=DIRECTION('',(0.,1.,0.));
#32229=DIRECTION('',(-0.939692620785908,0.,0.342020143325669));
#32230=DIRECTION('center_axis',(-1.,0.,0.));
#32231=DIRECTION('ref_axis',(0.,0.,1.));
#32232=DIRECTION('',(0.,1.,0.));
#32233=DIRECTION('',(0.,0.,1.));
#32234=DIRECTION('center_axis',(-0.342020143325669,0.,0.939692620785908));
#32235=DIRECTION('ref_axis',(0.939692620785908,0.,0.342020143325669));
#32236=DIRECTION('',(0.939692620785908,0.,0.342020143325669));
#32237=DIRECTION('center_axis',(0.819152044288976,0.,0.573576436351068));
#32238=DIRECTION('ref_axis',(0.573576436351068,0.,-0.819152044288976));
#32239=DIRECTION('',(0.497542812164537,0.497542812164537,-0.71056477546161));
#32240=DIRECTION('',(0.,1.,0.));
#32241=DIRECTION('',(-0.497542812164537,0.497542812164537,0.71056477546161));
#32242=DIRECTION('',(-0.49754281216453,-0.497542812164559,0.7105647754616));
#32243=DIRECTION('',(0.,-1.,0.));
#32244=DIRECTION('',(0.49754281216453,-0.49754281216456,-0.710564775461599));
#32245=DIRECTION('center_axis',(0.241844762647992,0.7071067811865,0.664463024388719));
#32246=DIRECTION('ref_axis',(0.939692620785908,0.,-0.342020143325669));
#32247=DIRECTION('',(-0.633687274224668,0.633687274224668,-0.443712606279585));
#32248=DIRECTION('',(-0.633687274224648,0.633687274224657,-0.443712606279629));
#32249=DIRECTION('',(0.939692620785908,0.,-0.342020143325669));
#32250=DIRECTION('center_axis',(0.707106781186548,0.707106781186548,0.));
#32251=DIRECTION('ref_axis',(0.,0.,-1.));
#32252=DIRECTION('',(0.,0.,-1.));
#32253=DIRECTION('',(0.497542812164537,-0.497542812164537,0.71056477546161));
#32254=DIRECTION('',(0.633687274224667,-0.633687274224667,-0.443712606279586));
#32255=DIRECTION('center_axis',(1.,0.,0.));
#32256=DIRECTION('ref_axis',(0.,1.,0.));
#32257=DIRECTION('',(0.,0.,1.));
#32258=DIRECTION('',(0.,-1.,0.));
#32259=DIRECTION('center_axis',(0.819152044288976,0.,-0.573576436351068));
#32260=DIRECTION('ref_axis',(-0.573576436351068,0.,-0.819152044288976));
#32261=DIRECTION('',(-0.497542812164537,-0.497542812164537,-0.71056477546161));
#32262=DIRECTION('',(-0.497542812164543,0.497542812164522,-0.710564775461617));
#32263=DIRECTION('',(0.,1.,0.));
#32264=DIRECTION('',(0.497542812164531,0.497542812164558,0.7105647754616));
#32265=DIRECTION('center_axis',(0.241844762647991,0.707106781186501,-0.664463024388718));
#32266=DIRECTION('ref_axis',(-0.939692620785908,0.,-0.342020143325669));
#32267=DIRECTION('',(-0.939692620785908,0.,-0.342020143325669));
#32268=DIRECTION('',(-0.633687274224651,0.633687274224655,0.443712606279627));
#32269=DIRECTION('center_axis',(0.819152044289004,0.,0.573576436351029));
#32270=DIRECTION('ref_axis',(0.573576436351029,0.,-0.819152044289004));
#32271=DIRECTION('',(0.497542812164512,0.497542812164512,-0.710564775461646));
#32272=DIRECTION('',(0.,1.,0.));
#32273=DIRECTION('',(-0.497542812164512,0.497542812164512,0.710564775461646));
#32274=DIRECTION('',(-0.4975428121645,-0.497542812164548,0.710564775461629));
#32275=DIRECTION('',(0.,-1.,0.));
#32276=DIRECTION('',(0.497542812164487,-0.497542812164587,-0.71056477546161));
#32277=DIRECTION('center_axis',(0.24184476264798,0.707106781186534,0.664463024388687));
#32278=DIRECTION('ref_axis',(0.939692620785908,0.,-0.342020143325669));
#32279=DIRECTION('',(-0.633687274224649,0.633687274224649,-0.443712606279638));
#32280=DIRECTION('',(-0.633687274224659,0.633687274224649,-0.443712606279623));
#32281=DIRECTION('',(0.939692620785908,0.,-0.342020143325669));
#32282=DIRECTION('center_axis',(0.707106781186548,0.707106781186548,0.));
#32283=DIRECTION('ref_axis',(0.,0.,-1.));
#32284=DIRECTION('',(0.,0.,-1.));
#32285=DIRECTION('',(0.497542812164486,-0.497542812164486,0.710564775461682));
#32286=DIRECTION('',(0.633687274224649,-0.633687274224649,-0.443712606279638));
#32287=DIRECTION('center_axis',(1.,0.,0.));
#32288=DIRECTION('ref_axis',(0.,1.,0.));
#32289=DIRECTION('',(0.,0.,1.));
#32290=DIRECTION('',(0.,-1.,0.));
#32291=DIRECTION('center_axis',(0.819152044289031,0.,-0.57357643635099));
#32292=DIRECTION('ref_axis',(-0.57357643635099,0.,-0.819152044289031));
#32293=DIRECTION('',(-0.497542812164486,-0.497542812164486,-0.710564775461682));
#32294=DIRECTION('',(-0.497542812164458,0.497542812164571,-0.710564775461641));
#32295=DIRECTION('',(0.,1.,0.));
#32296=DIRECTION('',(0.497542812164457,0.497542812164574,0.71056477546164));
#32297=DIRECTION('center_axis',(0.24184476264798,0.707106781186534,-0.664463024388687));
#32298=DIRECTION('ref_axis',(-0.939692620785908,0.,-0.342020143325669));
#32299=DIRECTION('',(-0.939692620785908,0.,-0.342020143325669));
#32300=DIRECTION('',(-0.633687274224651,0.633687274224655,0.443712606279627));
#32301=DIRECTION('center_axis',(0.819152044289031,0.,0.57357643635099));
#32302=DIRECTION('ref_axis',(0.57357643635099,0.,-0.819152044289031));
#32303=DIRECTION('',(0.497542812164486,0.497542812164486,-0.710564775461682));
#32304=DIRECTION('',(0.,1.,0.));
#32305=DIRECTION('',(-0.497542812164486,0.497542812164486,0.710564775461682));
#32306=DIRECTION('',(-0.497542812164457,-0.497542812164574,0.71056477546164));
#32307=DIRECTION('',(0.,-1.,0.));
#32308=DIRECTION('',(0.497542812164458,-0.497542812164572,-0.710564775461641));
#32309=DIRECTION('center_axis',(0.24184476264798,0.707106781186534,0.664463024388687));
#32310=DIRECTION('ref_axis',(0.939692620785908,0.,-0.342020143325669));
#32311=DIRECTION('',(-0.633687274224649,0.633687274224649,-0.443712606279638));
#32312=DIRECTION('',(-0.633687274224654,0.633687274224652,-0.443712606279625));
#32313=DIRECTION('',(0.939692620785908,0.,-0.342020143325669));
#32314=DIRECTION('center_axis',(0.707106781186548,0.707106781186548,0.));
#32315=DIRECTION('ref_axis',(0.,0.,-1.));
#32316=DIRECTION('',(0.,0.,-1.));
#32317=DIRECTION('',(0.497542812164512,-0.497542812164512,0.710564775461646));
#32318=DIRECTION('',(0.633687274224649,-0.633687274224649,-0.443712606279639));
#32319=DIRECTION('center_axis',(1.,0.,0.));
#32320=DIRECTION('ref_axis',(0.,1.,0.));
#32321=DIRECTION('',(0.,0.,1.));
#32322=DIRECTION('',(0.,-1.,0.));
#32323=DIRECTION('center_axis',(0.819152044289004,0.,-0.573576436351029));
#32324=DIRECTION('ref_axis',(-0.573576436351029,0.,-0.819152044289004));
#32325=DIRECTION('',(-0.497542812164512,-0.497542812164512,-0.710564775461646));
#32326=DIRECTION('',(-0.4975428121645,0.497542812164549,-0.710564775461628));
#32327=DIRECTION('',(0.,1.,0.));
#32328=DIRECTION('',(0.4975428121645,0.497542812164547,0.710564775461629));
#32329=DIRECTION('center_axis',(0.24184476264798,0.707106781186535,-0.664463024388686));
#32330=DIRECTION('ref_axis',(-0.939692620785908,0.,-0.342020143325669));
#32331=DIRECTION('',(-0.939692620785908,0.,-0.342020143325669));
#32332=DIRECTION('',(-0.633687274224651,0.633687274224655,0.443712606279627));
#32333=DIRECTION('center_axis',(0.819152044289004,0.,0.573576436351029));
#32334=DIRECTION('ref_axis',(0.573576436351029,0.,-0.819152044289004));
#32335=DIRECTION('',(0.497542812164512,0.497542812164512,-0.710564775461646));
#32336=DIRECTION('',(0.,1.,0.));
#32337=DIRECTION('',(-0.497542812164512,0.497542812164512,0.710564775461646));
#32338=DIRECTION('',(-0.4975428121645,-0.497542812164546,0.710564775461629));
#32339=DIRECTION('',(0.,-1.,0.));
#32340=DIRECTION('',(0.4975428121645,-0.497542812164548,-0.710564775461629));
#32341=DIRECTION('center_axis',(-0.342020143325669,0.,-0.939692620785908));
#32342=DIRECTION('ref_axis',(-0.939692620785908,0.,0.342020143325669));
#32343=DIRECTION('',(0.939692620785908,0.,-0.342020143325669));
#32344=DIRECTION('',(0.,1.,0.));
#32345=DIRECTION('',(-0.939692620785908,0.,0.342020143325669));
#32346=DIRECTION('center_axis',(0.24184476264798,0.707106781186536,0.664463024388686));
#32347=DIRECTION('ref_axis',(0.939692620785908,0.,-0.342020143325669));
#32348=DIRECTION('',(-0.633687274224648,0.633687274224648,-0.44371260627964));
#32349=DIRECTION('',(-0.633687274224633,0.633687274224639,-0.443712606279676));
#32350=DIRECTION('center_axis',(0.707106781186548,0.707106781186548,0.));
#32351=DIRECTION('ref_axis',(0.,0.,-1.));
#32352=DIRECTION('',(0.,0.,-1.));
#32353=DIRECTION('',(0.497542812164537,-0.497542812164537,0.71056477546161));
#32354=DIRECTION('',(0.633687274224667,-0.633687274224667,-0.443712606279586));
#32355=DIRECTION('center_axis',(0.819152044288976,0.,-0.573576436351068));
#32356=DIRECTION('ref_axis',(-0.573576436351068,0.,-0.819152044288976));
#32357=DIRECTION('',(0.,-1.,0.));
#32358=DIRECTION('',(-0.497542812164537,-0.497542812164537,-0.71056477546161));
#32359=DIRECTION('',(-0.49754281216453,0.49754281216456,-0.710564775461599));
#32360=DIRECTION('',(0.,1.,0.));
#32361=DIRECTION('',(0.497542812164531,0.497542812164558,0.7105647754616));
#32362=DIRECTION('center_axis',(-0.342020143325669,0.,0.939692620785908));
#32363=DIRECTION('ref_axis',(0.939692620785908,0.,0.342020143325669));
#32364=DIRECTION('',(0.939692620785908,0.,0.342020143325669));
#32365=DIRECTION('',(0.,1.,0.));
#32366=DIRECTION('',(-0.939692620785908,0.,-0.342020143325669));
#32367=DIRECTION('center_axis',(0.241844762647992,-0.707106781186499,-0.66446302438872));
#32368=DIRECTION('ref_axis',(-0.939692620785908,0.,-0.342020143325669));
#32369=DIRECTION('',(-0.633687274224668,-0.633687274224668,0.443712606279584));
#32370=DIRECTION('',(-0.939692620785908,0.,-0.342020143325669));
#32371=DIRECTION('',(0.633687274224669,0.633687274224671,-0.443712606279578));
#32372=DIRECTION('center_axis',(0.707106781186548,-0.707106781186548,0.));
#32373=DIRECTION('ref_axis',(0.,0.,-1.));
#32374=DIRECTION('',(0.633687274224649,0.633687274224649,0.443712606279638));
#32375=DIRECTION('',(0.,0.,-1.));
#32376=DIRECTION('',(0.,0.,1.));
#32377=DIRECTION('center_axis',(0.819152044289004,0.,0.573576436351029));
#32378=DIRECTION('ref_axis',(0.573576436351029,0.,-0.819152044289004));
#32379=DIRECTION('',(0.497542812164512,0.497542812164512,-0.710564775461646));
#32380=DIRECTION('',(0.,1.,0.));
#32381=DIRECTION('',(-0.497542812164512,0.497542812164512,0.710564775461646));
#32382=DIRECTION('',(-0.4975428121645,-0.497542812164548,0.710564775461629));
#32383=DIRECTION('',(0.,-1.,0.));
#32384=DIRECTION('',(0.497542812164487,-0.497542812164587,-0.71056477546161));
#32385=DIRECTION('center_axis',(0.24184476264798,0.707106781186534,0.664463024388687));
#32386=DIRECTION('ref_axis',(0.939692620785908,0.,-0.342020143325669));
#32387=DIRECTION('',(-0.633687274224649,0.633687274224649,-0.443712606279638));
#32388=DIRECTION('',(-0.633687274224657,0.633687274224651,-0.443712606279624));
#32389=DIRECTION('',(0.939692620785908,0.,-0.342020143325669));
#32390=DIRECTION('center_axis',(0.707106781186548,0.707106781186548,0.));
#32391=DIRECTION('ref_axis',(0.,0.,-1.));
#32392=DIRECTION('',(0.,0.,-1.));
#32393=DIRECTION('',(0.497542812164486,-0.497542812164486,0.710564775461682));
#32394=DIRECTION('',(0.633687274224649,-0.633687274224649,-0.443712606279638));
#32395=DIRECTION('center_axis',(1.,0.,0.));
#32396=DIRECTION('ref_axis',(0.,1.,0.));
#32397=DIRECTION('',(0.,0.,1.));
#32398=DIRECTION('',(0.,-1.,0.));
#32399=DIRECTION('center_axis',(0.819152044289031,0.,-0.57357643635099));
#32400=DIRECTION('ref_axis',(-0.57357643635099,0.,-0.819152044289031));
#32401=DIRECTION('',(-0.497542812164486,-0.497542812164486,-0.710564775461682));
#32402=DIRECTION('',(-0.497542812164458,0.497542812164571,-0.710564775461641));
#32403=DIRECTION('',(0.,1.,0.));
#32404=DIRECTION('',(0.497542812164457,0.497542812164574,0.71056477546164));
#32405=DIRECTION('center_axis',(0.24184476264798,0.707106781186534,-0.664463024388687));
#32406=DIRECTION('ref_axis',(-0.939692620785908,0.,-0.342020143325669));
#32407=DIRECTION('',(-0.939692620785908,0.,-0.342020143325669));
#32408=DIRECTION('',(-0.633687274224651,0.633687274224655,0.443712606279627));
#32409=DIRECTION('center_axis',(0.819152044289004,0.,0.573576436351029));
#32410=DIRECTION('ref_axis',(0.573576436351029,0.,-0.819152044289004));
#32411=DIRECTION('',(0.497542812164512,0.497542812164512,-0.710564775461646));
#32412=DIRECTION('',(0.,1.,0.));
#32413=DIRECTION('',(-0.497542812164512,0.497542812164512,0.710564775461646));
#32414=DIRECTION('',(-0.4975428121645,-0.497542812164548,0.710564775461629));
#32415=DIRECTION('',(0.,-1.,0.));
#32416=DIRECTION('',(0.4975428121645,-0.497542812164546,-0.710564775461629));
#32417=DIRECTION('center_axis',(0.24184476264798,0.707106781186534,0.664463024388687));
#32418=DIRECTION('ref_axis',(0.939692620785908,0.,-0.342020143325669));
#32419=DIRECTION('',(-0.633687274224649,0.633687274224649,-0.443712606279638));
#32420=DIRECTION('',(-0.633687274224654,0.633687274224652,-0.443712606279625));
#32421=DIRECTION('',(0.939692620785908,0.,-0.342020143325669));
#32422=DIRECTION('center_axis',(0.707106781186548,0.707106781186548,0.));
#32423=DIRECTION('ref_axis',(0.,0.,-1.));
#32424=DIRECTION('',(0.,0.,-1.));
#32425=DIRECTION('',(0.497542812164512,-0.497542812164512,0.710564775461646));
#32426=DIRECTION('',(0.633687274224649,-0.633687274224649,-0.443712606279639));
#32427=DIRECTION('center_axis',(1.,0.,0.));
#32428=DIRECTION('ref_axis',(0.,1.,0.));
#32429=DIRECTION('',(0.,0.,1.));
#32430=DIRECTION('',(0.,-1.,0.));
#32431=DIRECTION('center_axis',(0.819152044289004,0.,-0.573576436351029));
#32432=DIRECTION('ref_axis',(-0.573576436351029,0.,-0.819152044289004));
#32433=DIRECTION('',(-0.497542812164512,-0.497542812164512,-0.710564775461646));
#32434=DIRECTION('',(-0.497542812164487,0.497542812164587,-0.71056477546161));
#32435=DIRECTION('',(0.,1.,0.));
#32436=DIRECTION('',(0.4975428121645,0.497542812164547,0.710564775461629));
#32437=DIRECTION('center_axis',(0.24184476264798,0.707106781186536,-0.664463024388686));
#32438=DIRECTION('ref_axis',(-0.939692620785908,0.,-0.342020143325669));
#32439=DIRECTION('',(-0.939692620785908,0.,-0.342020143325669));
#32440=DIRECTION('',(-0.633687274224651,0.633687274224655,0.443712606279627));
#32441=DIRECTION('center_axis',(0.819152044289004,0.,0.573576436351029));
#32442=DIRECTION('ref_axis',(0.573576436351029,0.,-0.819152044289004));
#32443=DIRECTION('',(0.497542812164512,0.497542812164512,-0.710564775461646));
#32444=DIRECTION('',(-0.4975428121645,-0.497542812164546,0.710564775461629));
#32445=DIRECTION('',(0.,-1.,0.));
#32446=DIRECTION('',(0.4975428121645,-0.497542812164548,-0.710564775461629));
#32447=DIRECTION('center_axis',(0.24184476264798,-0.707106781186534,0.664463024388687));
#32448=DIRECTION('ref_axis',(0.939692620785908,0.,-0.342020143325669));
#32449=DIRECTION('',(-0.939692620785908,0.,0.342020143325669));
#32450=DIRECTION('',(0.633687274224654,0.633687274224652,0.443712606279625));
#32451=DIRECTION('',(0.939692620785908,0.,-0.342020143325669));
#32452=DIRECTION('',(0.633687274224649,0.633687274224649,0.443712606279638));
#32453=DIRECTION('center_axis',(-0.342020143325669,0.,-0.939692620785908));
#32454=DIRECTION('ref_axis',(-0.939692620785908,0.,0.342020143325669));
#32455=DIRECTION('',(0.939692620785908,0.,-0.342020143325669));
#32456=DIRECTION('',(0.,1.,0.));
#32457=DIRECTION('center_axis',(0.24184476264798,0.707106781186536,0.664463024388686));
#32458=DIRECTION('ref_axis',(0.939692620785908,0.,-0.342020143325669));
#32459=DIRECTION('',(-0.633687274224633,0.633687274224639,-0.443712606279676));
#32460=DIRECTION('center_axis',(0.70710678118655,0.707106781186545,0.));
#32461=DIRECTION('ref_axis',(0.,0.,-1.));
#32462=DIRECTION('',(0.,0.,-1.));
#32463=DIRECTION('center_axis',(-1.,0.,0.));
#32464=DIRECTION('ref_axis',(0.,0.,1.));
#32465=DIRECTION('',(0.,1.,0.));
#32466=DIRECTION('',(0.,0.,1.));
#32467=DIRECTION('center_axis',(-0.342020143325669,0.,0.939692620785908));
#32468=DIRECTION('ref_axis',(0.939692620785908,0.,0.342020143325669));
#32469=DIRECTION('',(0.939692620785908,0.,0.342020143325669));
#32470=DIRECTION('center_axis',(0.70710678118655,0.707106781186545,0.));
#32471=DIRECTION('ref_axis',(0.,0.,-1.));
#32472=DIRECTION('',(0.,0.,-1.));
#32473=DIRECTION('center_axis',(-0.342020143325669,0.,-0.939692620785908));
#32474=DIRECTION('ref_axis',(-0.939692620785908,0.,0.342020143325669));
#32475=DIRECTION('',(0.,1.,0.));
#32476=DIRECTION('',(-0.939692620785908,0.,0.342020143325669));
#32477=DIRECTION('center_axis',(-1.,0.,0.));
#32478=DIRECTION('ref_axis',(0.,0.,1.));
#32479=DIRECTION('',(0.,1.,0.));
#32480=DIRECTION('',(0.,0.,1.));
#32481=DIRECTION('center_axis',(-0.342020143325669,0.,0.939692620785908));
#32482=DIRECTION('ref_axis',(0.939692620785908,0.,0.342020143325669));
#32483=DIRECTION('',(0.939692620785908,0.,0.342020143325669));
#32484=DIRECTION('center_axis',(0.241844762647991,0.707106781186501,-0.664463024388718));
#32485=DIRECTION('ref_axis',(-0.939692620785908,0.,-0.342020143325669));
#32486=DIRECTION('',(-0.633687274224651,0.633687274224655,0.443712606279627));
#32487=DIRECTION('center_axis',(0.70710678118655,0.707106781186545,0.));
#32488=DIRECTION('ref_axis',(0.,0.,-1.));
#32489=DIRECTION('',(0.,0.,-1.));
#32490=DIRECTION('center_axis',(-0.342020143325669,0.,-0.939692620785908));
#32491=DIRECTION('ref_axis',(-0.939692620785908,0.,0.342020143325669));
#32492=DIRECTION('',(0.,1.,0.));
#32493=DIRECTION('',(-0.939692620785908,0.,0.342020143325669));
#32494=DIRECTION('center_axis',(-1.,0.,0.));
#32495=DIRECTION('ref_axis',(0.,0.,1.));
#32496=DIRECTION('',(0.,0.,1.));
#32497=DIRECTION('center_axis',(0.70710678118655,0.707106781186545,0.));
#32498=DIRECTION('ref_axis',(0.,0.,-1.));
#32499=DIRECTION('',(0.,0.,-1.));
#32500=DIRECTION('center_axis',(-1.,0.,0.));
#32501=DIRECTION('ref_axis',(0.,0.,1.));
#32502=DIRECTION('',(0.,1.,0.));
#32503=DIRECTION('',(0.,0.,1.));
#32504=DIRECTION('center_axis',(-0.342020143325669,0.,0.939692620785908));
#32505=DIRECTION('ref_axis',(0.939692620785908,0.,0.342020143325669));
#32506=DIRECTION('',(0.939692620785908,0.,0.342020143325669));
#32507=DIRECTION('center_axis',(0.70710678118655,0.707106781186545,0.));
#32508=DIRECTION('ref_axis',(0.,0.,-1.));
#32509=DIRECTION('',(0.,0.,-1.));
#32510=DIRECTION('center_axis',(-0.342020143325669,0.,-0.939692620785908));
#32511=DIRECTION('ref_axis',(-0.939692620785908,0.,0.342020143325669));
#32512=DIRECTION('',(0.,1.,0.));
#32513=DIRECTION('',(-0.939692620785908,0.,0.342020143325669));
#32514=DIRECTION('center_axis',(-1.,0.,0.));
#32515=DIRECTION('ref_axis',(0.,0.,1.));
#32516=DIRECTION('',(0.,1.,0.));
#32517=DIRECTION('',(0.,0.,1.));
#32518=DIRECTION('center_axis',(-0.342020143325669,0.,0.939692620785908));
#32519=DIRECTION('ref_axis',(0.939692620785908,0.,0.342020143325669));
#32520=DIRECTION('',(0.939692620785908,0.,0.342020143325669));
#32521=DIRECTION('center_axis',(0.70710678118655,0.707106781186545,0.));
#32522=DIRECTION('ref_axis',(0.,0.,-1.));
#32523=DIRECTION('',(0.,0.,-1.));
#32524=DIRECTION('center_axis',(-0.342020143325669,0.,-0.939692620785908));
#32525=DIRECTION('ref_axis',(-0.939692620785908,0.,0.342020143325669));
#32526=DIRECTION('',(0.,1.,0.));
#32527=DIRECTION('',(-0.939692620785908,0.,0.342020143325669));
#32528=DIRECTION('center_axis',(-1.,0.,0.));
#32529=DIRECTION('ref_axis',(0.,0.,1.));
#32530=DIRECTION('',(0.,1.,0.));
#32531=DIRECTION('',(0.,0.,1.));
#32532=DIRECTION('center_axis',(-0.342020143325669,0.,0.939692620785908));
#32533=DIRECTION('ref_axis',(0.939692620785908,0.,0.342020143325669));
#32534=DIRECTION('',(0.939692620785908,0.,0.342020143325669));
#32535=DIRECTION('center_axis',(0.70710678118655,0.707106781186545,0.));
#32536=DIRECTION('ref_axis',(0.,0.,-1.));
#32537=DIRECTION('',(0.,0.,-1.));
#32538=DIRECTION('center_axis',(-0.342020143325669,0.,-0.939692620785908));
#32539=DIRECTION('ref_axis',(-0.939692620785908,0.,0.342020143325669));
#32540=DIRECTION('',(0.,1.,0.));
#32541=DIRECTION('',(-0.939692620785908,0.,0.342020143325669));
#32542=DIRECTION('center_axis',(-1.,0.,0.));
#32543=DIRECTION('ref_axis',(0.,0.,1.));
#32544=DIRECTION('',(0.,0.,1.));
#32545=DIRECTION('center_axis',(0.70710678118655,0.707106781186545,0.));
#32546=DIRECTION('ref_axis',(0.,0.,-1.));
#32547=DIRECTION('',(0.,0.,-1.));
#32548=DIRECTION('center_axis',(-1.,0.,0.));
#32549=DIRECTION('ref_axis',(0.,0.,1.));
#32550=DIRECTION('',(0.,1.,0.));
#32551=DIRECTION('',(0.,0.,1.));
#32552=DIRECTION('center_axis',(-0.342020143325669,0.,0.939692620785908));
#32553=DIRECTION('ref_axis',(0.939692620785908,0.,0.342020143325669));
#32554=DIRECTION('',(0.939692620785908,0.,0.342020143325669));
#32555=DIRECTION('center_axis',(0.70710678118655,0.707106781186545,0.));
#32556=DIRECTION('ref_axis',(0.,0.,-1.));
#32557=DIRECTION('',(0.,0.,-1.));
#32558=DIRECTION('center_axis',(-0.342020143325669,0.,-0.939692620785908));
#32559=DIRECTION('ref_axis',(-0.939692620785908,0.,0.342020143325669));
#32560=DIRECTION('',(0.,1.,0.));
#32561=DIRECTION('',(-0.939692620785908,0.,0.342020143325669));
#32562=DIRECTION('center_axis',(-1.,0.,0.));
#32563=DIRECTION('ref_axis',(0.,0.,1.));
#32564=DIRECTION('',(0.,1.,0.));
#32565=DIRECTION('',(0.,0.,1.));
#32566=DIRECTION('center_axis',(-0.342020143325669,0.,0.939692620785908));
#32567=DIRECTION('ref_axis',(0.939692620785908,0.,0.342020143325669));
#32568=DIRECTION('',(0.939692620785908,0.,0.342020143325669));
#32569=DIRECTION('center_axis',(0.819152044289004,0.,0.573576436351029));
#32570=DIRECTION('ref_axis',(0.573576436351029,0.,-0.819152044289004));
#32571=DIRECTION('',(0.497542812164512,0.497542812164512,-0.710564775461646));
#32572=DIRECTION('',(0.,1.,0.));
#32573=DIRECTION('',(-0.497542812164512,0.497542812164512,0.710564775461646));
#32574=DIRECTION('',(-0.497542812164502,-0.497542812164542,0.710564775461631));
#32575=DIRECTION('',(0.,-1.,0.));
#32576=DIRECTION('',(0.497542812164502,-0.497542812164542,-0.710564775461631));
#32577=DIRECTION('center_axis',(0.241844762647986,0.707106781186536,0.664463024388684));
#32578=DIRECTION('ref_axis',(0.939692620785905,0.,-0.342020143325678));
#32579=DIRECTION('',(-0.63368727422465,0.63368727422465,-0.443712606279636));
#32580=DIRECTION('',(-0.633687274224657,0.633687274224651,-0.443712606279624));
#32581=DIRECTION('',(0.939692620785905,0.,-0.342020143325678));
#32582=DIRECTION('center_axis',(0.707106781186548,0.707106781186548,0.));
#32583=DIRECTION('ref_axis',(0.,0.,-1.));
#32584=DIRECTION('',(0.,0.,-1.));
#32585=DIRECTION('',(0.497542812164483,-0.497542812164483,0.710564775461686));
#32586=DIRECTION('',(0.63368727422463,-0.63368727422463,-0.443712606279693));
#32587=DIRECTION('center_axis',(1.,0.,0.));
#32588=DIRECTION('ref_axis',(0.,1.,0.));
#32589=DIRECTION('',(0.,0.,1.));
#32590=DIRECTION('',(0.,-1.,0.));
#32591=DIRECTION('center_axis',(0.819152044289035,0.,-0.573576436350985));
#32592=DIRECTION('ref_axis',(-0.573576436350985,0.,-0.819152044289035));
#32593=DIRECTION('',(-0.497542812164483,-0.497542812164483,-0.710564775461686));
#32594=DIRECTION('',(-0.497542812164467,0.497542812164533,-0.710564775461663));
#32595=DIRECTION('',(0.,1.,0.));
#32596=DIRECTION('',(0.497542812164467,0.497542812164531,0.710564775461663));
#32597=DIRECTION('center_axis',(0.241844762647973,0.707106781186573,-0.664463024388649));
#32598=DIRECTION('ref_axis',(-0.939692620785905,0.,-0.342020143325678));
#32599=DIRECTION('',(-0.939692620785905,0.,-0.342020143325678));
#32600=DIRECTION('',(-0.633687274224617,0.633687274224621,0.443712606279724));
#32601=DIRECTION('center_axis',(0.819152044289007,0.,0.573576436351024));
#32602=DIRECTION('ref_axis',(0.573576436351024,0.,-0.819152044289007));
#32603=DIRECTION('',(0.497542812164509,0.497542812164509,-0.71056477546165));
#32604=DIRECTION('',(0.,1.,0.));
#32605=DIRECTION('',(-0.497542812164509,0.497542812164509,0.71056477546165));
#32606=DIRECTION('',(-0.497542812164497,-0.497542812164545,0.710564775461633));
#32607=DIRECTION('',(0.,-1.,0.));
#32608=DIRECTION('',(0.497542812164509,-0.497542812164509,-0.71056477546165));
#32609=DIRECTION('center_axis',(0.241844762647986,0.707106781186536,0.664463024388684));
#32610=DIRECTION('ref_axis',(0.939692620785905,0.,-0.342020143325678));
#32611=DIRECTION('',(-0.63368727422465,0.63368727422465,-0.443712606279636));
#32612=DIRECTION('',(-0.633687274224657,0.633687274224651,-0.443712606279624));
#32613=DIRECTION('',(0.939692620785905,0.,-0.342020143325678));
#32614=DIRECTION('center_axis',(0.707106781186548,0.707106781186548,0.));
#32615=DIRECTION('ref_axis',(0.,0.,-1.));
#32616=DIRECTION('',(0.,0.,-1.));
#32617=DIRECTION('',(0.497542812164536,-0.497542812164536,0.710564775461612));
#32618=DIRECTION('',(0.63368727422465,-0.63368727422465,-0.443712606279635));
#32619=DIRECTION('center_axis',(1.,0.,0.));
#32620=DIRECTION('ref_axis',(0.,1.,0.));
#32621=DIRECTION('',(0.,0.,1.));
#32622=DIRECTION('',(0.,-1.,0.));
#32623=DIRECTION('center_axis',(0.819152044288978,0.,-0.573576436351066));
#32624=DIRECTION('ref_axis',(-0.573576436351066,0.,-0.819152044288978));
#32625=DIRECTION('',(-0.497542812164536,-0.497542812164536,-0.710564775461612));
#32626=DIRECTION('',(-0.497542812164528,0.49754281216456,-0.7105647754616));
#32627=DIRECTION('',(0.,1.,0.));
#32628=DIRECTION('',(0.497542812164539,0.497542812164525,0.710564775461617));
#32629=DIRECTION('center_axis',(0.24184476264798,0.707106781186533,-0.664463024388688));
#32630=DIRECTION('ref_axis',(-0.939692620785908,0.,-0.342020143325669));
#32631=DIRECTION('',(-0.939692620785908,0.,-0.342020143325669));
#32632=DIRECTION('',(-0.633687274224651,0.633687274224655,0.443712606279627));
#32633=DIRECTION('center_axis',(0.81915204428898,0.,0.573576436351063));
#32634=DIRECTION('ref_axis',(0.573576436351063,0.,-0.81915204428898));
#32635=DIRECTION('',(0.497542812164534,0.497542812164534,-0.710564775461614));
#32636=DIRECTION('',(0.,1.,0.));
#32637=DIRECTION('',(-0.497542812164534,0.497542812164534,0.710564775461614));
#32638=DIRECTION('',(-0.497542812164527,-0.497542812164557,0.710564775461603));
#32639=DIRECTION('',(0.,-1.,0.));
#32640=DIRECTION('',(0.497542812164539,-0.497542812164519,-0.710564775461621));
#32641=DIRECTION('center_axis',(0.241844762647998,0.7071067811865,0.664463024388717));
#32642=DIRECTION('ref_axis',(0.939692620785905,0.,-0.342020143325678));
#32643=DIRECTION('',(-0.633687274224669,0.633687274224669,-0.443712606279581));
#32644=DIRECTION('',(-0.633687274224674,0.633687274224668,-0.443712606279576));
#32645=DIRECTION('',(0.939692620785905,0.,-0.342020143325678));
#32646=DIRECTION('center_axis',(0.707106781186548,0.707106781186548,0.));
#32647=DIRECTION('ref_axis',(0.,0.,-1.));
#32648=DIRECTION('',(0.,0.,-1.));
#32649=DIRECTION('',(0.497542812164512,-0.497542812164512,0.710564775461646));
#32650=DIRECTION('',(0.633687274224649,-0.633687274224649,-0.443712606279638));
#32651=DIRECTION('center_axis',(1.,0.,0.));
#32652=DIRECTION('ref_axis',(0.,1.,0.));
#32653=DIRECTION('',(0.,0.,1.));
#32654=DIRECTION('',(0.,-1.,0.));
#32655=DIRECTION('center_axis',(0.819152044289004,0.,-0.573576436351029));
#32656=DIRECTION('ref_axis',(-0.573576436351029,0.,-0.819152044289004));
#32657=DIRECTION('',(-0.497542812164512,-0.497542812164512,-0.710564775461646));
#32658=DIRECTION('',(-0.497542812164502,0.497542812164542,-0.710564775461631));
#32659=DIRECTION('',(0.,1.,0.));
#32660=DIRECTION('',(0.497542812164502,0.497542812164541,0.710564775461632));
#32661=DIRECTION('center_axis',(0.241844762647985,0.707106781186537,-0.664463024388683));
#32662=DIRECTION('ref_axis',(-0.939692620785905,0.,-0.342020143325678));
#32663=DIRECTION('',(-0.939692620785905,0.,-0.342020143325678));
#32664=DIRECTION('',(-0.633687274224651,0.633687274224655,0.443712606279627));
#32665=DIRECTION('center_axis',(0.819152044289007,0.,0.573576436351024));
#32666=DIRECTION('ref_axis',(0.573576436351024,0.,-0.819152044289007));
#32667=DIRECTION('',(0.497542812164509,0.497542812164509,-0.71056477546165));
#32668=DIRECTION('',(0.,1.,0.));
#32669=DIRECTION('',(-0.497542812164509,0.497542812164509,0.71056477546165));
#32670=DIRECTION('',(-0.497542812164497,-0.497542812164545,0.710564775461633));
#32671=DIRECTION('',(0.,-1.,0.));
#32672=DIRECTION('',(0.497542812164497,-0.497542812164545,-0.710564775461633));
#32673=DIRECTION('center_axis',(0.241844762647986,0.707106781186536,0.664463024388684));
#32674=DIRECTION('ref_axis',(0.939692620785905,0.,-0.342020143325678));
#32675=DIRECTION('',(-0.63368727422465,0.63368727422465,-0.443712606279636));
#32676=DIRECTION('',(-0.633687274224652,0.633687274224654,-0.443712606279627));
#32677=DIRECTION('',(0.939692620785905,0.,-0.342020143325678));
#32678=DIRECTION('center_axis',(0.707106781186548,0.707106781186548,0.));
#32679=DIRECTION('ref_axis',(0.,0.,-1.));
#32680=DIRECTION('',(0.,0.,-1.));
#32681=DIRECTION('',(0.497542812164483,-0.497542812164483,0.710564775461686));
#32682=DIRECTION('',(0.63368727422463,-0.63368727422463,-0.443712606279692));
#32683=DIRECTION('center_axis',(1.,0.,0.));
#32684=DIRECTION('ref_axis',(0.,1.,0.));
#32685=DIRECTION('',(0.,0.,1.));
#32686=DIRECTION('',(0.,-1.,0.));
#32687=DIRECTION('center_axis',(0.819152044289035,0.,-0.573576436350985));
#32688=DIRECTION('ref_axis',(-0.573576436350985,0.,-0.819152044289035));
#32689=DIRECTION('',(-0.497542812164483,-0.497542812164483,-0.710564775461686));
#32690=DIRECTION('',(-0.497542812164467,0.497542812164533,-0.710564775461663));
#32691=DIRECTION('',(0.,1.,0.));
#32692=DIRECTION('',(0.497542812164467,0.497542812164532,0.710564775461663));
#32693=DIRECTION('center_axis',(0.241844762647973,0.707106781186572,-0.664463024388649));
#32694=DIRECTION('ref_axis',(-0.939692620785905,0.,-0.342020143325678));
#32695=DIRECTION('',(-0.939692620785905,0.,-0.342020143325678));
#32696=DIRECTION('',(-0.633687274224617,0.633687274224621,0.443712606279724));
#32697=DIRECTION('center_axis',(0.819152044289007,0.,0.573576436351024));
#32698=DIRECTION('ref_axis',(0.573576436351024,0.,-0.819152044289007));
#32699=DIRECTION('',(0.497542812164509,0.497542812164509,-0.71056477546165));
#32700=DIRECTION('',(0.,1.,0.));
#32701=DIRECTION('',(-0.497542812164509,0.497542812164509,0.71056477546165));
#32702=DIRECTION('',(-0.497542812164497,-0.497542812164543,0.710564775461634));
#32703=DIRECTION('',(0.,-1.,0.));
#32704=DIRECTION('',(0.497542812164497,-0.497542812164545,-0.710564775461633));
#32705=DIRECTION('center_axis',(0.241844762647985,0.707106781186537,0.664463024388682));
#32706=DIRECTION('ref_axis',(0.939692620785905,0.,-0.342020143325678));
#32707=DIRECTION('',(-0.633687274224649,0.633687274224649,-0.443712606279638));
#32708=DIRECTION('',(-0.633687274224657,0.633687274224651,-0.443712606279624));
#32709=DIRECTION('',(0.939692620785905,0.,-0.342020143325678));
#32710=DIRECTION('center_axis',(0.707106781186548,0.707106781186548,0.));
#32711=DIRECTION('ref_axis',(0.,0.,-1.));
#32712=DIRECTION('',(0.,0.,-1.));
#32713=DIRECTION('',(0.497542812164512,-0.497542812164512,0.710564775461646));
#32714=DIRECTION('',(0.633687274224649,-0.633687274224649,-0.443712606279637));
#32715=DIRECTION('center_axis',(1.,0.,0.));
#32716=DIRECTION('ref_axis',(0.,1.,0.));
#32717=DIRECTION('',(0.,0.,1.));
#32718=DIRECTION('',(0.,-1.,0.));
#32719=DIRECTION('center_axis',(0.819152044289004,0.,-0.573576436351029));
#32720=DIRECTION('ref_axis',(-0.573576436351029,0.,-0.819152044289004));
#32721=DIRECTION('',(-0.497542812164512,-0.497542812164512,-0.710564775461646));
#32722=DIRECTION('',(-0.497542812164502,0.497542812164542,-0.710564775461631));
#32723=DIRECTION('',(0.,1.,0.));
#32724=DIRECTION('',(0.497542812164502,0.497542812164541,0.710564775461632));
#32725=DIRECTION('center_axis',(0.241844762647985,0.707106781186537,-0.664463024388683));
#32726=DIRECTION('ref_axis',(-0.939692620785905,0.,-0.342020143325678));
#32727=DIRECTION('',(-0.939692620785905,0.,-0.342020143325678));
#32728=DIRECTION('',(-0.633687274224651,0.633687274224655,0.443712606279627));
#32729=DIRECTION('center_axis',(0.819152044289002,0.,0.573576436351031));
#32730=DIRECTION('ref_axis',(0.573576436351031,0.,-0.819152044289002));
#32731=DIRECTION('',(0.497542812164513,0.497542812164513,-0.710564775461643));
#32732=DIRECTION('',(0.,1.,0.));
#32733=DIRECTION('',(-0.497542812164513,0.497542812164513,0.710564775461643));
#32734=DIRECTION('',(-0.497542812164502,-0.497542812164546,0.710564775461628));
#32735=DIRECTION('',(0.,-1.,0.));
#32736=DIRECTION('',(0.497542812164503,-0.497542812164544,-0.710564775461629));
#32737=DIRECTION('center_axis',(0.24184476264798,0.707106781186534,0.664463024388687));
#32738=DIRECTION('ref_axis',(0.939692620785908,0.,-0.342020143325669));
#32739=DIRECTION('',(-0.633687274224649,0.633687274224649,-0.443712606279638));
#32740=DIRECTION('',(-0.633687274224652,0.633687274224654,-0.443712606279627));
#32741=DIRECTION('',(0.939692620785908,0.,-0.342020143325669));
#32742=DIRECTION('center_axis',(0.707106781186548,0.707106781186548,0.));
#32743=DIRECTION('ref_axis',(0.,0.,-1.));
#32744=DIRECTION('',(0.,0.,-1.));
#32745=DIRECTION('',(0.497542812164513,-0.497542812164513,0.710564775461643));
#32746=DIRECTION('',(0.633687274224649,-0.633687274224649,-0.443712606279638));
#32747=DIRECTION('center_axis',(1.,0.,0.));
#32748=DIRECTION('ref_axis',(0.,1.,0.));
#32749=DIRECTION('',(0.,0.,1.));
#32750=DIRECTION('',(0.,-1.,0.));
#32751=DIRECTION('center_axis',(0.819152044289002,0.,-0.573576436351031));
#32752=DIRECTION('ref_axis',(-0.573576436351031,0.,-0.819152044289002));
#32753=DIRECTION('',(-0.497542812164513,-0.497542812164513,-0.710564775461643));
#32754=DIRECTION('',(-0.497542812164502,0.497542812164548,-0.710564775461627));
#32755=DIRECTION('',(0.,1.,0.));
#32756=DIRECTION('',(0.497542812164503,0.497542812164546,0.710564775461628));
#32757=DIRECTION('center_axis',(0.24184476264798,0.707106781186535,-0.664463024388686));
#32758=DIRECTION('ref_axis',(-0.939692620785908,0.,-0.342020143325669));
#32759=DIRECTION('',(-0.939692620785908,0.,-0.342020143325669));
#32760=DIRECTION('',(-0.633687274224651,0.633687274224655,0.443712606279627));
#32761=DIRECTION('center_axis',(0.819152044288976,0.,0.573576436351068));
#32762=DIRECTION('ref_axis',(0.573576436351068,0.,-0.819152044288976));
#32763=DIRECTION('',(0.497542812164537,0.497542812164537,-0.71056477546161));
#32764=DIRECTION('',(-0.497542812164518,-0.497542812164595,0.710564775461582));
#32765=DIRECTION('',(0.,-1.,0.));
#32766=DIRECTION('',(0.49754281216453,-0.49754281216456,-0.710564775461599));
#32767=DIRECTION('center_axis',(0.241844762647992,-0.707106781186499,0.66446302438872));
#32768=DIRECTION('ref_axis',(0.939692620785908,0.,-0.342020143325669));
#32769=DIRECTION('',(-0.939692620785908,0.,0.342020143325669));
#32770=DIRECTION('',(0.633687274224669,0.633687274224671,0.443712606279578));
#32771=DIRECTION('',(0.939692620785908,0.,-0.342020143325669));
#32772=DIRECTION('',(0.633687274224668,0.633687274224668,0.443712606279584));
#32773=DIRECTION('center_axis',(-0.342020143325669,0.,-0.939692620785908));
#32774=DIRECTION('ref_axis',(-0.939692620785908,0.,0.342020143325669));
#32775=DIRECTION('',(0.939692620785908,0.,-0.342020143325669));
#32776=DIRECTION('',(0.,1.,0.));
#32777=DIRECTION('center_axis',(0.241844762648004,0.707106781186466,0.664463024388752));
#32778=DIRECTION('ref_axis',(0.939692620785908,0.,-0.342020143325669));
#32779=DIRECTION('',(-0.633687274224695,0.633687274224682,-0.443712606279526));
#32780=DIRECTION('center_axis',(0.70710678118655,0.707106781186545,0.));
#32781=DIRECTION('ref_axis',(0.,0.,-1.));
#32782=DIRECTION('',(0.,0.,-1.));
#32783=DIRECTION('center_axis',(-1.,0.,0.));
#32784=DIRECTION('ref_axis',(0.,0.,1.));
#32785=DIRECTION('',(0.,1.,0.));
#32786=DIRECTION('',(0.,0.,1.));
#32787=DIRECTION('center_axis',(-0.342020143325669,0.,0.939692620785908));
#32788=DIRECTION('ref_axis',(0.939692620785908,0.,0.342020143325669));
#32789=DIRECTION('',(0.939692620785908,0.,0.342020143325669));
#32790=DIRECTION('center_axis',(0.70710678118655,0.707106781186545,0.));
#32791=DIRECTION('ref_axis',(0.,0.,-1.));
#32792=DIRECTION('',(0.,0.,-1.));
#32793=DIRECTION('center_axis',(-0.342020143325669,0.,-0.939692620785908));
#32794=DIRECTION('ref_axis',(-0.939692620785908,0.,0.342020143325669));
#32795=DIRECTION('',(0.,1.,0.));
#32796=DIRECTION('',(-0.939692620785908,0.,0.342020143325669));
#32797=DIRECTION('center_axis',(-1.,0.,0.));
#32798=DIRECTION('ref_axis',(0.,0.,1.));
#32799=DIRECTION('',(0.,1.,0.));
#32800=DIRECTION('',(0.,0.,1.));
#32801=DIRECTION('center_axis',(-0.342020143325678,0.,0.939692620785905));
#32802=DIRECTION('ref_axis',(0.939692620785905,0.,0.342020143325678));
#32803=DIRECTION('',(0.939692620785905,0.,0.342020143325678));
#32804=DIRECTION('center_axis',(0.70710678118655,0.707106781186545,0.));
#32805=DIRECTION('ref_axis',(0.,0.,-1.));
#32806=DIRECTION('',(0.,0.,-1.));
#32807=DIRECTION('center_axis',(-0.342020143325678,0.,-0.939692620785905));
#32808=DIRECTION('ref_axis',(-0.939692620785905,0.,0.342020143325678));
#32809=DIRECTION('',(0.,1.,0.));
#32810=DIRECTION('',(-0.939692620785905,0.,0.342020143325678));
#32811=DIRECTION('center_axis',(-1.,0.,0.));
#32812=DIRECTION('ref_axis',(0.,0.,1.));
#32813=DIRECTION('',(0.,1.,0.));
#32814=DIRECTION('',(0.,0.,1.));
#32815=DIRECTION('center_axis',(-0.342020143325678,0.,0.939692620785905));
#32816=DIRECTION('ref_axis',(0.939692620785905,0.,0.342020143325678));
#32817=DIRECTION('',(0.939692620785905,0.,0.342020143325678));
#32818=DIRECTION('center_axis',(0.70710678118655,0.707106781186545,0.));
#32819=DIRECTION('ref_axis',(0.,0.,-1.));
#32820=DIRECTION('',(0.,0.,-1.));
#32821=DIRECTION('center_axis',(-0.342020143325678,0.,-0.939692620785905));
#32822=DIRECTION('ref_axis',(-0.939692620785905,0.,0.342020143325678));
#32823=DIRECTION('',(0.,1.,0.));
#32824=DIRECTION('',(-0.939692620785905,0.,0.342020143325678));
#32825=DIRECTION('center_axis',(-1.,0.,0.));
#32826=DIRECTION('ref_axis',(0.,0.,1.));
#32827=DIRECTION('',(0.,1.,0.));
#32828=DIRECTION('',(0.,0.,1.));
#32829=DIRECTION('center_axis',(-0.342020143325678,0.,0.939692620785905));
#32830=DIRECTION('ref_axis',(0.939692620785905,0.,0.342020143325678));
#32831=DIRECTION('',(0.939692620785905,0.,0.342020143325678));
#32832=DIRECTION('center_axis',(0.70710678118655,0.707106781186545,0.));
#32833=DIRECTION('ref_axis',(0.,0.,-1.));
#32834=DIRECTION('',(0.,0.,-1.));
#32835=DIRECTION('center_axis',(-0.342020143325678,0.,-0.939692620785905));
#32836=DIRECTION('ref_axis',(-0.939692620785905,0.,0.342020143325678));
#32837=DIRECTION('',(0.,1.,0.));
#32838=DIRECTION('',(-0.939692620785905,0.,0.342020143325678));
#32839=DIRECTION('center_axis',(-1.,0.,0.));
#32840=DIRECTION('ref_axis',(0.,0.,1.));
#32841=DIRECTION('',(0.,1.,0.));
#32842=DIRECTION('',(0.,0.,1.));
#32843=DIRECTION('center_axis',(-0.342020143325669,0.,0.939692620785908));
#32844=DIRECTION('ref_axis',(0.939692620785908,0.,0.342020143325669));
#32845=DIRECTION('',(0.939692620785908,0.,0.342020143325669));
#32846=DIRECTION('center_axis',(0.70710678118655,0.707106781186545,0.));
#32847=DIRECTION('ref_axis',(0.,0.,-1.));
#32848=DIRECTION('',(0.,0.,-1.));
#32849=DIRECTION('center_axis',(-0.342020143325678,0.,-0.939692620785905));
#32850=DIRECTION('ref_axis',(-0.939692620785905,0.,0.342020143325678));
#32851=DIRECTION('',(0.,1.,0.));
#32852=DIRECTION('',(-0.939692620785905,0.,0.342020143325678));
#32853=DIRECTION('center_axis',(-1.,0.,0.));
#32854=DIRECTION('ref_axis',(0.,0.,1.));
#32855=DIRECTION('',(0.,1.,0.));
#32856=DIRECTION('',(0.,0.,1.));
#32857=DIRECTION('center_axis',(-0.342020143325678,0.,0.939692620785905));
#32858=DIRECTION('ref_axis',(0.939692620785905,0.,0.342020143325678));
#32859=DIRECTION('',(0.939692620785905,0.,0.342020143325678));
#32860=DIRECTION('center_axis',(0.70710678118655,0.707106781186545,0.));
#32861=DIRECTION('ref_axis',(0.,0.,-1.));
#32862=DIRECTION('',(-0.633687274224646,0.63368727422465,0.443712606279641));
#32863=DIRECTION('',(0.,0.,-1.));
#32864=DIRECTION('center_axis',(-0.342020143325678,0.,-0.939692620785905));
#32865=DIRECTION('ref_axis',(-0.939692620785905,0.,0.342020143325678));
#32866=DIRECTION('',(0.,1.,0.));
#32867=DIRECTION('',(-0.939692620785905,0.,0.342020143325678));
#32868=DIRECTION('center_axis',(-1.,0.,0.));
#32869=DIRECTION('ref_axis',(0.,0.,1.));
#32870=DIRECTION('',(0.,0.,1.));
#32871=DIRECTION('center_axis',(0.241844762647985,0.707106781186537,-0.664463024388682));
#32872=DIRECTION('ref_axis',(-0.939692620785905,0.,-0.342020143325678));
#32873=DIRECTION('',(0.633687274224649,-0.633687274224649,-0.443712606279638));
#32874=DIRECTION('center_axis',(0.24184476264798,-0.707106781186534,-0.664463024388687));
#32875=DIRECTION('ref_axis',(-0.939692620785908,0.,-0.342020143325669));
#32876=DIRECTION('',(-0.633687274224649,-0.633687274224649,0.443712606279638));
#32877=DIRECTION('',(-0.939692620785908,0.,-0.342020143325669));
#32878=DIRECTION('',(0.633687274224652,0.633687274224654,-0.443712606279627));
#32879=DIRECTION('center_axis',(0.707106781186549,-0.707106781186546,0.));
#32880=DIRECTION('ref_axis',(0.,0.,-1.));
#32881=DIRECTION('',(0.,0.,-1.));
#32882=DIRECTION('',(0.633687274224661,0.633687274224648,0.443712606279622));
#32883=DIRECTION('center_axis',(0.241844762647997,-0.707106781186503,0.664463024388715));
#32884=DIRECTION('ref_axis',(0.939692620785905,0.,-0.342020143325678));
#32885=DIRECTION('',(0.939692620785905,0.,-0.342020143325678));
#32886=DIRECTION('',(0.633687274224667,0.633687274224667,0.443712606279586));
#32887=DIRECTION('center_axis',(0.,-1.,0.));
#32888=DIRECTION('ref_axis',(1.,0.,0.));
#32889=DIRECTION('',(0.,0.,-1.));
#32890=DIRECTION('',(0.939692620785905,0.,-0.342020143325678));
#32891=DIRECTION('',(0.,0.,-1.));
#32892=DIRECTION('',(-0.939692620785905,0.,-0.342020143325678));
#32893=DIRECTION('',(0.,0.,-1.));
#32894=DIRECTION('',(0.939692620785908,0.,-0.342020143325669));
#32895=DIRECTION('',(0.,0.,-1.));
#32896=DIRECTION('',(-0.939692620785908,0.,-0.342020143325669));
#32897=DIRECTION('',(0.,0.,-1.));
#32898=DIRECTION('',(-1.,0.,0.));
#32899=DIRECTION('',(0.,0.,-1.));
#32900=DIRECTION('',(0.,0.,-1.));
#32901=DIRECTION('',(-0.939692620785908,0.,-0.342020143325669));
#32902=DIRECTION('',(0.,0.,-1.));
#32903=DIRECTION('',(0.939692620785908,0.,-0.342020143325669));
#32904=DIRECTION('',(0.,0.,-1.));
#32905=DIRECTION('',(-0.939692620785908,0.,-0.342020143325669));
#32906=DIRECTION('',(0.,0.,-1.));
#32907=DIRECTION('',(0.939692620785908,0.,-0.342020143325669));
#32908=DIRECTION('',(0.,0.,-1.));
#32909=DIRECTION('',(0.939692620785908,0.,-0.342020143325669));
#32910=DIRECTION('',(0.,0.,-1.));
#32911=DIRECTION('',(-0.939692620785908,0.,-0.342020143325669));
#32912=DIRECTION('',(0.,0.,-1.));
#32913=DIRECTION('',(0.939692620785908,0.,-0.342020143325669));
#32914=DIRECTION('',(0.,0.,-1.));
#32915=DIRECTION('',(0.,0.,-1.));
#32916=DIRECTION('',(0.939692620785908,0.,-0.342020143325669));
#32917=DIRECTION('',(0.,0.,-1.));
#32918=DIRECTION('',(-0.939692620785908,0.,-0.342020143325669));
#32919=DIRECTION('',(0.,0.,-1.));
#32920=DIRECTION('',(0.939692620785908,0.,-0.342020143325669));
#32921=DIRECTION('',(0.,0.,-1.));
#32922=DIRECTION('',(-0.939692620785908,0.,-0.342020143325669));
#32923=DIRECTION('',(0.,0.,-1.));
#32924=DIRECTION('',(0.,0.,-1.));
#32925=DIRECTION('',(-0.939692620785908,0.,-0.342020143325669));
#32926=DIRECTION('',(0.,0.,-1.));
#32927=DIRECTION('',(0.939692620785908,0.,-0.342020143325669));
#32928=DIRECTION('',(0.,0.,-1.));
#32929=DIRECTION('',(-0.939692620785908,0.,-0.342020143325669));
#32930=DIRECTION('',(0.,0.,-1.));
#32931=DIRECTION('',(0.939692620785908,0.,-0.342020143325669));
#32932=DIRECTION('',(0.,0.,-1.));
#32933=DIRECTION('',(0.939692620785908,0.,-0.342020143325669));
#32934=DIRECTION('',(0.,0.,-1.));
#32935=DIRECTION('',(-0.939692620785908,0.,-0.342020143325669));
#32936=DIRECTION('',(0.,0.,-1.));
#32937=DIRECTION('',(0.939692620785908,0.,-0.342020143325669));
#32938=DIRECTION('',(0.,0.,-1.));
#32939=DIRECTION('',(-0.939692620785908,0.,-0.342020143325669));
#32940=DIRECTION('',(0.,0.,-1.));
#32941=DIRECTION('',(0.939692620785908,0.,-0.342020143325669));
#32942=DIRECTION('',(0.,0.,-1.));
#32943=DIRECTION('',(-0.939692620785908,0.,-0.342020143325669));
#32944=DIRECTION('',(0.,0.,-1.));
#32945=DIRECTION('',(0.939692620785908,0.,-0.342020143325669));
#32946=DIRECTION('',(0.,0.,-1.));
#32947=DIRECTION('',(0.,0.,-1.));
#32948=DIRECTION('',(0.939692620785908,0.,-0.342020143325669));
#32949=DIRECTION('',(0.,0.,-1.));
#32950=DIRECTION('',(-0.939692620785908,0.,-0.342020143325669));
#32951=DIRECTION('',(0.,0.,-1.));
#32952=DIRECTION('',(0.939692620785908,0.,-0.342020143325669));
#32953=DIRECTION('',(0.,0.,-1.));
#32954=DIRECTION('',(-0.939692620785908,0.,-0.342020143325669));
#32955=DIRECTION('',(0.,0.,-1.));
#32956=DIRECTION('',(0.,0.,-1.));
#32957=DIRECTION('',(-0.939692620785908,0.,-0.342020143325669));
#32958=DIRECTION('',(0.,0.,-1.));
#32959=DIRECTION('',(0.939692620785908,0.,-0.342020143325669));
#32960=DIRECTION('',(0.,0.,-1.));
#32961=DIRECTION('',(-0.939692620785905,0.,-0.342020143325678));
#32962=DIRECTION('',(0.,0.,-1.));
#32963=DIRECTION('',(0.939692620785905,0.,-0.342020143325678));
#32964=DIRECTION('',(0.,0.,-1.));
#32965=DIRECTION('',(-0.939692620785905,0.,-0.342020143325678));
#32966=DIRECTION('',(0.,0.,-1.));
#32967=DIRECTION('',(0.939692620785905,0.,-0.342020143325678));
#32968=DIRECTION('',(0.,0.,-1.));
#32969=DIRECTION('',(-0.939692620785905,0.,-0.342020143325678));
#32970=DIRECTION('',(0.,0.,-1.));
#32971=DIRECTION('',(0.939692620785905,0.,-0.342020143325678));
#32972=DIRECTION('',(0.,0.,-1.));
#32973=DIRECTION('',(-0.939692620785908,0.,-0.342020143325669));
#32974=DIRECTION('',(0.,0.,-1.));
#32975=DIRECTION('',(0.939692620785905,0.,-0.342020143325678));
#32976=DIRECTION('',(0.,0.,-1.));
#32977=DIRECTION('',(-0.939692620785905,0.,-0.342020143325678));
#32978=DIRECTION('',(0.,0.,-1.));
#32979=DIRECTION('',(0.939692620785905,0.,-0.342020143325678));
#32980=DIRECTION('',(0.,0.,-1.));
#32981=DIRECTION('',(0.,0.,-1.));
#32982=DIRECTION('',(-0.939692620785908,0.,-0.342020143325669));
#32983=DIRECTION('',(0.,0.,-1.));
#32984=DIRECTION('',(0.939692620785905,0.,-0.342020143325678));
#32985=DIRECTION('',(0.,0.,-1.));
#32986=DIRECTION('',(-0.939692620785905,0.,-0.342020143325678));
#32987=DIRECTION('',(0.,0.,-1.));
#32988=DIRECTION('',(0.939692620785905,0.,-0.342020143325678));
#32989=DIRECTION('',(0.,0.,-1.));
#32990=DIRECTION('',(0.,0.,-1.));
#32991=DIRECTION('',(0.939692620785905,0.,-0.342020143325678));
#32992=DIRECTION('',(0.,0.,-1.));
#32993=DIRECTION('',(-0.939692620785908,0.,-0.342020143325669));
#32994=DIRECTION('',(0.,0.,-1.));
#32995=DIRECTION('',(0.939692620785905,0.,-0.342020143325678));
#32996=DIRECTION('',(0.,0.,-1.));
#32997=DIRECTION('',(-0.939692620785905,0.,-0.342020143325678));
#32998=DIRECTION('',(0.,0.,-1.));
#32999=DIRECTION('',(0.939692620785905,0.,-0.342020143325678));
#33000=DIRECTION('',(0.,0.,-1.));
#33001=DIRECTION('',(-0.939692620785905,0.,-0.342020143325678));
#33002=DIRECTION('',(0.,0.,-1.));
#33003=DIRECTION('center_axis',(0.,-1.,0.));
#33004=DIRECTION('ref_axis',(0.,0.,1.));
#33005=DIRECTION('center_axis',(0.707106781186548,-0.707106781186548,0.));
#33006=DIRECTION('ref_axis',(0.,0.,-1.));
#33007=DIRECTION('',(0.63368727422465,0.63368727422465,0.443712606279634));
#33008=DIRECTION('center_axis',(0.241844762647985,-0.707106781186537,-0.664463024388682));
#33009=DIRECTION('ref_axis',(-0.939692620785905,0.,-0.342020143325678));
#33010=DIRECTION('',(-0.633687274224649,-0.633687274224649,0.443712606279638));
#33011=DIRECTION('',(0.633687274224635,0.633687274224637,-0.443712606279675));
#33012=DIRECTION('center_axis',(0.707106781186549,-0.707106781186546,0.));
#33013=DIRECTION('ref_axis',(0.,0.,-1.));
#33014=DIRECTION('',(0.633687274224642,0.633687274224633,0.443712606279672));
#33015=DIRECTION('center_axis',(0.241844762647985,-0.707106781186539,0.664463024388681));
#33016=DIRECTION('ref_axis',(0.939692620785905,0.,-0.342020143325678));
#33017=DIRECTION('',(0.633687274224648,0.633687274224648,0.443712606279641));
#33018=DIRECTION('center_axis',(0.707106781186548,-0.707106781186548,0.));
#33019=DIRECTION('ref_axis',(0.,0.,-1.));
#33020=DIRECTION('center_axis',(0.241844762647973,-0.707106781186573,-0.664463024388649));
#33021=DIRECTION('ref_axis',(-0.939692620785905,0.,-0.342020143325678));
#33022=DIRECTION('',(-0.63368727422463,-0.63368727422463,0.443712606279693));
#33023=DIRECTION('',(0.633687274224618,0.63368727422462,-0.443712606279723));
#33024=DIRECTION('center_axis',(0.707106781186549,-0.707106781186546,0.));
#33025=DIRECTION('ref_axis',(0.,0.,-1.));
#33026=DIRECTION('',(0.633687274224635,0.633687274224637,0.443712606279675));
#33027=DIRECTION('center_axis',(0.241844762647974,-0.70710678118657,0.664463024388651));
#33028=DIRECTION('ref_axis',(0.939692620785905,0.,-0.342020143325678));
#33029=DIRECTION('',(0.633687274224631,0.633687274224631,0.443712606279689));
#33030=DIRECTION('center_axis',(0.707106781186548,-0.707106781186548,0.));
#33031=DIRECTION('ref_axis',(0.,0.,-1.));
#33032=DIRECTION('center_axis',(0.24184476264798,-0.707106781186534,-0.664463024388687));
#33033=DIRECTION('ref_axis',(-0.939692620785908,0.,-0.342020143325669));
#33034=DIRECTION('',(-0.633687274224649,-0.633687274224649,0.443712606279638));
#33035=DIRECTION('',(0.633687274224652,0.633687274224654,-0.443712606279627));
#33036=DIRECTION('center_axis',(0.707106781186549,-0.707106781186546,0.));
#33037=DIRECTION('ref_axis',(0.,0.,-1.));
#33038=DIRECTION('',(0.63368727422465,0.633687274224655,0.443712606279628));
#33039=DIRECTION('center_axis',(0.241844762647986,-0.707106781186534,0.664463024388685));
#33040=DIRECTION('ref_axis',(0.939692620785905,0.,-0.342020143325678));
#33041=DIRECTION('',(0.63368727422465,0.63368727422465,0.443712606279634));
#33042=DIRECTION('center_axis',(0.707106781186548,-0.707106781186548,0.));
#33043=DIRECTION('ref_axis',(0.,0.,-1.));
#33044=DIRECTION('center_axis',(0.707106781186549,-0.707106781186546,0.));
#33045=DIRECTION('ref_axis',(0.,0.,-1.));
#33046=DIRECTION('',(0.633687274224652,0.633687274224654,0.443712606279627));
#33047=DIRECTION('center_axis',(0.241844762647986,-0.707106781186534,0.664463024388685));
#33048=DIRECTION('ref_axis',(0.939692620785905,0.,-0.342020143325678));
#33049=DIRECTION('',(0.63368727422465,0.63368727422465,0.443712606279634));
#33050=DIRECTION('center_axis',(0.707106781186548,-0.707106781186548,0.));
#33051=DIRECTION('ref_axis',(0.,0.,-1.));
#33052=DIRECTION('',(0.,0.,1.));
#33053=DIRECTION('center_axis',(0.241844762647973,-0.707106781186573,-0.664463024388649));
#33054=DIRECTION('ref_axis',(-0.939692620785905,0.,-0.342020143325678));
#33055=DIRECTION('',(-0.63368727422463,-0.63368727422463,0.443712606279693));
#33056=DIRECTION('',(0.633687274224635,0.633687274224637,-0.443712606279675));
#33057=DIRECTION('center_axis',(0.707106781186549,-0.707106781186546,0.));
#33058=DIRECTION('ref_axis',(0.,0.,-1.));
#33059=DIRECTION('',(0.633687274224635,0.633687274224637,0.443712606279675));
#33060=DIRECTION('center_axis',(0.241844762647974,-0.70710678118657,0.664463024388651));
#33061=DIRECTION('ref_axis',(0.939692620785905,0.,-0.342020143325678));
#33062=DIRECTION('',(0.633687274224631,0.633687274224631,0.443712606279689));
#33063=DIRECTION('center_axis',(0.707106781186548,-0.707106781186548,0.));
#33064=DIRECTION('ref_axis',(0.,0.,-1.));
#33065=DIRECTION('center_axis',(0.24184476264798,-0.707106781186536,-0.664463024388686));
#33066=DIRECTION('ref_axis',(-0.939692620785908,0.,-0.342020143325669));
#33067=DIRECTION('',(-0.633687274224648,-0.633687274224648,0.44371260627964));
#33068=DIRECTION('',(-0.633687274224647,-0.633687274224649,0.443712606279641));
#33069=DIRECTION('center_axis',(0.707106781186549,-0.707106781186546,0.));
#33070=DIRECTION('ref_axis',(0.,0.,-1.));
#33071=DIRECTION('center_axis',(0.707106781186549,-0.707106781186546,0.));
#33072=DIRECTION('ref_axis',(0.,0.,-1.));
#33073=DIRECTION('',(0.633687274224652,0.633687274224654,0.443712606279627));
#33074=DIRECTION('center_axis',(0.241844762647986,-0.707106781186536,0.664463024388684));
#33075=DIRECTION('ref_axis',(0.939692620785905,0.,-0.342020143325678));
#33076=DIRECTION('',(0.63368727422465,0.63368727422465,0.443712606279636));
#33077=DIRECTION('center_axis',(0.241844762647973,-0.707106781186572,-0.66446302438865));
#33078=DIRECTION('ref_axis',(-0.939692620785905,0.,-0.342020143325678));
#33079=DIRECTION('',(-0.63368727422463,-0.63368727422463,0.443712606279691));
#33080=DIRECTION('',(0.633687274224635,0.633687274224637,-0.443712606279675));
#33081=DIRECTION('center_axis',(0.707106781186549,-0.707106781186546,0.));
#33082=DIRECTION('ref_axis',(0.,0.,-1.));
#33083=DIRECTION('',(0.633687274224637,0.633687274224636,0.443712606279674));
#33084=DIRECTION('center_axis',(0.241844762647974,-0.70710678118657,0.664463024388651));
#33085=DIRECTION('ref_axis',(0.939692620785905,0.,-0.342020143325678));
#33086=DIRECTION('',(0.633687274224631,0.633687274224631,0.443712606279689));
#33087=DIRECTION('center_axis',(0.707106781186548,-0.707106781186548,0.));
#33088=DIRECTION('ref_axis',(0.,0.,-1.));
#33089=DIRECTION('center_axis',(0.241844762647992,-0.7071067811865,-0.664463024388719));
#33090=DIRECTION('ref_axis',(-0.939692620785908,0.,-0.342020143325669));
#33091=DIRECTION('',(-0.633687274224668,-0.633687274224668,0.443712606279585));
#33092=DIRECTION('',(0.633687274224669,0.633687274224671,-0.443712606279578));
#33093=DIRECTION('center_axis',(0.707106781186549,-0.707106781186546,0.));
#33094=DIRECTION('ref_axis',(0.,0.,-1.));
#33095=DIRECTION('',(0.633687274224652,0.633687274224654,0.443712606279627));
#33096=DIRECTION('center_axis',(0.241844762647986,-0.707106781186536,0.664463024388684));
#33097=DIRECTION('ref_axis',(0.939692620785905,0.,-0.342020143325678));
#33098=DIRECTION('',(0.63368727422465,0.63368727422465,0.443712606279636));
#33099=DIRECTION('center_axis',(0.707106781186548,-0.707106781186548,0.));
#33100=DIRECTION('ref_axis',(0.,0.,-1.));
#33101=DIRECTION('center_axis',(0.241844762647986,-0.707106781186536,-0.664463024388684));
#33102=DIRECTION('ref_axis',(-0.939692620785905,0.,-0.342020143325678));
#33103=DIRECTION('',(-0.63368727422465,-0.63368727422465,0.443712606279636));
#33104=DIRECTION('',(0.633687274224652,0.633687274224654,-0.443712606279627));
#33105=DIRECTION('center_axis',(0.707106781186549,-0.707106781186546,0.));
#33106=DIRECTION('ref_axis',(0.,0.,-1.));
#33107=DIRECTION('',(0.633687274224654,0.633687274224652,0.443712606279625));
#33108=DIRECTION('center_axis',(0.241844762647986,-0.707106781186536,0.664463024388684));
#33109=DIRECTION('ref_axis',(0.939692620785905,0.,-0.342020143325678));
#33110=DIRECTION('',(0.63368727422465,0.63368727422465,0.443712606279636));
#33111=DIRECTION('center_axis',(0.707106781186548,-0.707106781186548,0.));
#33112=DIRECTION('ref_axis',(0.,0.,-1.));
#33113=DIRECTION('center_axis',(0.241844762647973,-0.707106781186572,-0.66446302438865));
#33114=DIRECTION('ref_axis',(-0.939692620785905,0.,-0.342020143325678));
#33115=DIRECTION('',(-0.63368727422463,-0.63368727422463,0.443712606279691));
#33116=DIRECTION('',(0.633687274224635,0.633687274224637,-0.443712606279675));
#33117=DIRECTION('center_axis',(0.707106781186549,-0.707106781186546,0.));
#33118=DIRECTION('ref_axis',(0.,0.,-1.));
#33119=DIRECTION('',(0.633687274224643,0.63368727422466,0.443712606279631));
#33120=DIRECTION('center_axis',(0.241844762647986,-0.707106781186536,0.664463024388684));
#33121=DIRECTION('ref_axis',(0.939692620785905,0.,-0.342020143325678));
#33122=DIRECTION('',(0.63368727422465,0.63368727422465,0.443712606279636));
#33123=DIRECTION('center_axis',(0.707106781186548,-0.707106781186548,0.));
#33124=DIRECTION('ref_axis',(0.,0.,-1.));
#33125=DIRECTION('center_axis',(0.241844762647986,-0.707106781186536,-0.664463024388684));
#33126=DIRECTION('ref_axis',(-0.939692620785905,0.,-0.342020143325678));
#33127=DIRECTION('',(-0.63368727422465,-0.63368727422465,0.443712606279636));
#33128=DIRECTION('',(0.633687274224652,0.633687274224654,-0.443712606279627));
#33129=DIRECTION('center_axis',(0.707106781186549,-0.707106781186546,0.));
#33130=DIRECTION('ref_axis',(0.,0.,-1.));
#33131=DIRECTION('',(0.633687274224642,0.633687274224633,0.443712606279672));
#33132=DIRECTION('center_axis',(0.241844762647979,-0.707106781186536,0.664463024388685));
#33133=DIRECTION('ref_axis',(0.939692620785908,0.,-0.342020143325669));
#33134=DIRECTION('',(0.633687274224648,0.633687274224648,0.443712606279641));
#33135=DIRECTION('center_axis',(0.707106781186548,-0.707106781186548,0.));
#33136=DIRECTION('ref_axis',(0.,0.,-1.));
#33137=DIRECTION('center_axis',(0.24184476264798,-0.707106781186533,-0.664463024388688));
#33138=DIRECTION('ref_axis',(-0.939692620785908,0.,-0.342020143325669));
#33139=DIRECTION('',(-0.63368727422465,-0.63368727422465,0.443712606279635));
#33140=DIRECTION('',(0.633687274224652,0.633687274224654,-0.443712606279627));
#33141=DIRECTION('center_axis',(0.707106781186549,-0.707106781186546,0.));
#33142=DIRECTION('ref_axis',(0.,0.,-1.));
#33143=DIRECTION('center_axis',(0.707106781186548,-0.707106781186548,0.));
#33144=DIRECTION('ref_axis',(0.,0.,-1.));
#33145=DIRECTION('center_axis',(0.24184476264798,-0.707106781186535,-0.664463024388686));
#33146=DIRECTION('ref_axis',(-0.939692620785908,0.,-0.342020143325669));
#33147=DIRECTION('',(-0.633687274224649,-0.633687274224649,0.443712606279638));
#33148=DIRECTION('',(0.633687274224652,0.633687274224654,-0.443712606279627));
#33149=DIRECTION('center_axis',(0.707106781186549,-0.707106781186546,0.));
#33150=DIRECTION('ref_axis',(0.,0.,-1.));
#33151=DIRECTION('',(0.633687274224654,0.633687274224652,0.443712606279625));
#33152=DIRECTION('center_axis',(0.24184476264798,-0.707106781186534,0.664463024388688));
#33153=DIRECTION('ref_axis',(0.939692620785908,0.,-0.342020143325669));
#33154=DIRECTION('',(0.63368727422465,0.63368727422465,0.443712606279636));
#33155=DIRECTION('center_axis',(0.707106781186548,-0.707106781186548,0.));
#33156=DIRECTION('ref_axis',(0.,0.,-1.));
#33157=DIRECTION('center_axis',(0.241844762647979,-0.707106781186536,-0.664463024388685));
#33158=DIRECTION('ref_axis',(-0.939692620785908,0.,-0.342020143325669));
#33159=DIRECTION('',(-0.633687274224648,-0.633687274224648,0.443712606279641));
#33160=DIRECTION('',(0.633687274224635,0.633687274224637,-0.443712606279675));
#33161=DIRECTION('center_axis',(0.707106781186549,-0.707106781186546,0.));
#33162=DIRECTION('ref_axis',(0.,0.,-1.));
#33163=DIRECTION('',(0.633687274224676,0.633687274224666,0.443712606279575));
#33164=DIRECTION('center_axis',(0.241844762647992,-0.707106781186501,0.664463024388719));
#33165=DIRECTION('ref_axis',(0.939692620785908,0.,-0.342020143325669));
#33166=DIRECTION('',(0.633687274224667,0.633687274224667,0.443712606279586));
#33167=DIRECTION('center_axis',(0.707106781186548,-0.707106781186548,0.));
#33168=DIRECTION('ref_axis',(0.,0.,-1.));
#33169=DIRECTION('center_axis',(0.707106781186549,-0.707106781186546,0.));
#33170=DIRECTION('ref_axis',(0.,0.,-1.));
#33171=DIRECTION('',(0.63368727422467,0.63368727422467,0.443712606279578));
#33172=DIRECTION('center_axis',(0.241844762647992,-0.707106781186499,0.66446302438872));
#33173=DIRECTION('ref_axis',(0.939692620785908,0.,-0.342020143325669));
#33174=DIRECTION('',(0.633687274224668,0.633687274224668,0.443712606279584));
#33175=DIRECTION('center_axis',(0.707106781186548,-0.707106781186548,0.));
#33176=DIRECTION('ref_axis',(0.,0.,-1.));
#33177=DIRECTION('',(0.,0.,1.));
#33178=DIRECTION('center_axis',(0.24184476264798,-0.707106781186535,-0.664463024388686));
#33179=DIRECTION('ref_axis',(-0.939692620785908,0.,-0.342020143325669));
#33180=DIRECTION('',(-0.633687274224649,-0.633687274224649,0.443712606279638));
#33181=DIRECTION('',(0.633687274224652,0.633687274224654,-0.443712606279627));
#33182=DIRECTION('center_axis',(0.707106781186549,-0.707106781186546,0.));
#33183=DIRECTION('ref_axis',(0.,0.,-1.));
#33184=DIRECTION('',(0.633687274224666,0.633687274224673,0.44371260627958));
#33185=DIRECTION('center_axis',(0.241844762647993,-0.707106781186497,0.664463024388722));
#33186=DIRECTION('ref_axis',(0.939692620785908,0.,-0.342020143325669));
#33187=DIRECTION('',(0.633687274224669,0.633687274224669,0.44371260627958));
#33188=DIRECTION('center_axis',(0.707106781186548,-0.707106781186548,0.));
#33189=DIRECTION('ref_axis',(0.,0.,-1.));
#33190=DIRECTION('center_axis',(0.241844762647979,-0.707106781186536,-0.664463024388685));
#33191=DIRECTION('ref_axis',(-0.939692620785908,0.,-0.342020143325669));
#33192=DIRECTION('',(-0.633687274224648,-0.633687274224648,0.443712606279641));
#33193=DIRECTION('',(0.633687274224635,0.633687274224637,-0.443712606279675));
#33194=DIRECTION('center_axis',(0.707106781186549,-0.707106781186546,0.));
#33195=DIRECTION('ref_axis',(0.,0.,-1.));
#33196=DIRECTION('',(0.63368727422466,0.633687274224649,0.443712606279623));
#33197=DIRECTION('center_axis',(0.24184476264798,-0.707106781186536,0.664463024388686));
#33198=DIRECTION('ref_axis',(0.939692620785908,0.,-0.342020143325669));
#33199=DIRECTION('',(0.633687274224648,0.633687274224648,0.44371260627964));
#33200=DIRECTION('center_axis',(0.707106781186548,-0.707106781186548,0.));
#33201=DIRECTION('ref_axis',(0.,0.,-1.));
#33202=DIRECTION('center_axis',(0.24184476264798,-0.707106781186534,-0.664463024388688));
#33203=DIRECTION('ref_axis',(-0.939692620785908,0.,-0.342020143325669));
#33204=DIRECTION('',(-0.63368727422465,-0.63368727422465,0.443712606279636));
#33205=DIRECTION('',(0.633687274224652,0.633687274224654,-0.443712606279627));
#33206=DIRECTION('center_axis',(0.707106781186549,-0.707106781186546,0.));
#33207=DIRECTION('ref_axis',(0.,0.,-1.));
#33208=DIRECTION('',(-0.633687274224648,-0.63368727422465,-0.443712606279639));
#33209=DIRECTION('center_axis',(0.24184476264798,-0.707106781186534,0.664463024388687));
#33210=DIRECTION('ref_axis',(0.939692620785908,0.,-0.342020143325669));
#33211=DIRECTION('center_axis',(0.707106781186549,-0.707106781186546,0.));
#33212=DIRECTION('ref_axis',(0.,0.,-1.));
#33213=DIRECTION('',(0.633687274224664,0.633687274224674,0.44371260627958));
#33214=DIRECTION('center_axis',(0.241844762647993,-0.707106781186497,0.664463024388722));
#33215=DIRECTION('ref_axis',(0.939692620785908,0.,-0.342020143325669));
#33216=DIRECTION('',(0.633687274224669,0.633687274224669,0.44371260627958));
#33217=DIRECTION('center_axis',(0.241844762647979,-0.707106781186536,-0.664463024388685));
#33218=DIRECTION('ref_axis',(-0.939692620785908,0.,-0.342020143325669));
#33219=DIRECTION('',(-0.633687274224648,-0.633687274224648,0.443712606279641));
#33220=DIRECTION('',(0.633687274224635,0.633687274224637,-0.443712606279675));
#33221=DIRECTION('center_axis',(0.707106781186549,-0.707106781186546,0.));
#33222=DIRECTION('ref_axis',(0.,0.,-1.));
#33223=DIRECTION('',(0.633687274224658,0.63368727422465,0.443712606279624));
#33224=DIRECTION('center_axis',(0.24184476264798,-0.707106781186536,0.664463024388686));
#33225=DIRECTION('ref_axis',(0.939692620785908,0.,-0.342020143325669));
#33226=DIRECTION('',(0.633687274224648,0.633687274224648,0.44371260627964));
#33227=DIRECTION('center_axis',(0.707106781186548,-0.707106781186548,0.));
#33228=DIRECTION('ref_axis',(0.,0.,-1.));
#33229=DIRECTION('center_axis',(0.241844762647993,-0.707106781186498,-0.664463024388721));
#33230=DIRECTION('ref_axis',(-0.939692620785908,0.,-0.342020143325669));
#33231=DIRECTION('',(-0.633687274224669,-0.633687274224669,0.443712606279582));
#33232=DIRECTION('',(0.633687274224669,0.633687274224671,-0.443712606279578));
#33233=DIRECTION('center_axis',(0.707106781186549,-0.707106781186546,0.));
#33234=DIRECTION('ref_axis',(0.,0.,-1.));
#33235=DIRECTION('center_axis',(0.707106781186548,-0.707106781186548,0.));
#33236=DIRECTION('ref_axis',(0.,0.,-1.));
#33237=DIRECTION('center_axis',(0.24184476264798,-0.707106781186535,-0.664463024388686));
#33238=DIRECTION('ref_axis',(-0.939692620785908,0.,-0.342020143325669));
#33239=DIRECTION('',(-0.633687274224649,-0.633687274224649,0.443712606279638));
#33240=DIRECTION('',(0.633687274224652,0.633687274224654,-0.443712606279627));
#33241=DIRECTION('center_axis',(0.707106781186549,-0.707106781186546,0.));
#33242=DIRECTION('ref_axis',(0.,0.,-1.));
#33243=DIRECTION('',(0.633687274224664,0.633687274224674,0.44371260627958));
#33244=DIRECTION('center_axis',(0.241844762647993,-0.707106781186497,0.664463024388722));
#33245=DIRECTION('ref_axis',(0.939692620785908,0.,-0.342020143325669));
#33246=DIRECTION('',(0.633687274224669,0.633687274224669,0.44371260627958));
#33247=DIRECTION('center_axis',(0.707106781186548,-0.707106781186548,0.));
#33248=DIRECTION('ref_axis',(0.,0.,-1.));
#33249=DIRECTION('center_axis',(0.241844762647979,-0.707106781186536,-0.664463024388685));
#33250=DIRECTION('ref_axis',(-0.939692620785908,0.,-0.342020143325669));
#33251=DIRECTION('',(-0.633687274224648,-0.633687274224648,0.443712606279641));
#33252=DIRECTION('',(0.633687274224635,0.633687274224637,-0.443712606279675));
#33253=DIRECTION('center_axis',(0.707106781186549,-0.707106781186546,0.));
#33254=DIRECTION('ref_axis',(0.,0.,-1.));
#33255=DIRECTION('',(0.633687274224658,0.63368727422465,0.443712606279624));
#33256=DIRECTION('center_axis',(0.24184476264798,-0.707106781186536,0.664463024388686));
#33257=DIRECTION('ref_axis',(0.939692620785908,0.,-0.342020143325669));
#33258=DIRECTION('',(0.633687274224648,0.633687274224648,0.44371260627964));
#33259=DIRECTION('center_axis',(0.707106781186548,-0.707106781186548,0.));
#33260=DIRECTION('ref_axis',(0.,0.,-1.));
#33261=DIRECTION('center_axis',(0.707106781186549,-0.707106781186546,0.));
#33262=DIRECTION('ref_axis',(0.,0.,-1.));
#33263=DIRECTION('',(0.633687274224653,0.633687274224653,0.443712606279626));
#33264=DIRECTION('center_axis',(0.24184476264798,-0.707106781186534,0.664463024388687));
#33265=DIRECTION('ref_axis',(0.939692620785908,0.,-0.342020143325669));
#33266=DIRECTION('',(0.633687274224649,0.633687274224649,0.443712606279638));
#33267=DIRECTION('center_axis',(0.707106781186548,-0.707106781186548,0.));
#33268=DIRECTION('ref_axis',(0.,0.,-1.));
#33269=DIRECTION('',(0.,0.,1.));
#33270=DIRECTION('center_axis',(0.241844762647992,-0.7071067811865,-0.66446302438872));
#33271=DIRECTION('ref_axis',(-0.939692620785908,0.,-0.342020143325669));
#33272=DIRECTION('',(-0.633687274224668,-0.633687274224668,0.443712606279584));
#33273=DIRECTION('',(-0.633687274224667,-0.633687274224668,0.443712606279585));
#33274=DIRECTION('center_axis',(0.707106781186549,-0.707106781186546,0.));
#33275=DIRECTION('ref_axis',(0.,0.,-1.));
#33276=DIRECTION('',(0.633687274224648,0.633687274224657,0.443712606279629));
#33277=DIRECTION('center_axis',(0.241844762647991,-0.707106781186501,0.664463024388718));
#33278=DIRECTION('ref_axis',(0.939692620785908,0.,-0.342020143325669));
#33279=DIRECTION('center_axis',(0.707106781186549,-0.707106781186546,0.));
#33280=DIRECTION('ref_axis',(0.,0.,-1.));
#33281=DIRECTION('',(0.633687274224658,0.63368727422465,0.443712606279624));
#33282=DIRECTION('center_axis',(0.24184476264798,-0.707106781186536,0.664463024388686));
#33283=DIRECTION('ref_axis',(0.939692620785908,0.,-0.342020143325669));
#33284=DIRECTION('',(0.633687274224648,0.633687274224648,0.44371260627964));
#33285=DIRECTION('center_axis',(0.241844762647968,-0.70710678118657,-0.664463024388653));
#33286=DIRECTION('ref_axis',(-0.939692620785908,0.,-0.342020143325669));
#33287=DIRECTION('',(-0.63368727422463,-0.63368727422463,0.443712606279692));
#33288=DIRECTION('',(0.633687274224635,0.633687274224637,-0.443712606279675));
#33289=DIRECTION('center_axis',(0.707106781186549,-0.707106781186546,0.));
#33290=DIRECTION('ref_axis',(0.,0.,-1.));
#33291=DIRECTION('',(0.633687274224652,0.633687274224654,0.443712606279627));
#33292=DIRECTION('center_axis',(0.24184476264798,-0.707106781186534,0.664463024388687));
#33293=DIRECTION('ref_axis',(0.939692620785908,0.,-0.342020143325669));
#33294=DIRECTION('',(0.633687274224649,0.633687274224649,0.443712606279637));
#33295=DIRECTION('center_axis',(0.707106781186548,-0.707106781186548,0.));
#33296=DIRECTION('ref_axis',(0.,0.,-1.));
#33297=DIRECTION('center_axis',(0.241844762647992,-0.7071067811865,-0.664463024388719));
#33298=DIRECTION('ref_axis',(-0.939692620785908,0.,-0.342020143325669));
#33299=DIRECTION('',(-0.633687274224668,-0.633687274224668,0.443712606279585));
#33300=DIRECTION('',(0.633687274224669,0.633687274224671,-0.443712606279578));
#33301=DIRECTION('center_axis',(0.707106781186549,-0.707106781186546,0.));
#33302=DIRECTION('ref_axis',(0.,0.,-1.));
#33303=DIRECTION('center_axis',(0.707106781186548,-0.707106781186548,0.));
#33304=DIRECTION('ref_axis',(0.,0.,-1.));
#33305=DIRECTION('center_axis',(0.,-0.923879532511285,-0.382683432365094));
#33306=DIRECTION('ref_axis',(0.,0.382683432365094,-0.923879532511285));
#33307=DIRECTION('',(0.67859834454585,-0.281084637714822,0.678598344545844));
#33308=DIRECTION('',(-0.357406744336596,-0.357406744336596,0.862856209461014));
#33309=DIRECTION('center_axis',(0.241844762647955,-0.707106781186607,-0.664463024388618));
#33310=DIRECTION('ref_axis',(-0.939692620785908,0.,-0.342020143325669));
#33311=DIRECTION('',(-0.63368727422461,-0.63368727422461,0.443712606279749));
#33312=DIRECTION('',(0.633687274224618,0.63368727422462,-0.443712606279723));
#33313=DIRECTION('center_axis',(0.707106781186549,-0.707106781186546,0.));
#33314=DIRECTION('ref_axis',(0.,0.,-1.));
#33315=DIRECTION('',(0.63368727422467,0.633687274224642,0.443712606279618));
#33316=DIRECTION('center_axis',(0.241844762647992,-0.7071067811865,0.664463024388719));
#33317=DIRECTION('ref_axis',(0.939692620785908,0.,-0.342020143325669));
#33318=DIRECTION('',(0.633687274224668,0.633687274224668,0.443712606279585));
#33319=DIRECTION('center_axis',(0.707106781186548,-0.707106781186548,0.));
#33320=DIRECTION('ref_axis',(0.,0.,-1.));
#33321=DIRECTION('center_axis',(0.241844762647973,-0.707106781186573,-0.664463024388649));
#33322=DIRECTION('ref_axis',(-0.939692620785905,0.,-0.342020143325678));
#33323=DIRECTION('',(-0.63368727422463,-0.63368727422463,0.443712606279693));
#33324=DIRECTION('',(0.633687274224618,0.63368727422462,-0.443712606279723));
#33325=DIRECTION('center_axis',(0.707106781186549,-0.707106781186546,0.));
#33326=DIRECTION('ref_axis',(0.,0.,-1.));
#33327=DIRECTION('',(0.633687274224648,0.633687274224657,0.443712606279629));
#33328=DIRECTION('center_axis',(0.241844762647986,-0.707106781186534,0.664463024388685));
#33329=DIRECTION('ref_axis',(0.939692620785905,0.,-0.342020143325678));
#33330=DIRECTION('center_axis',(0.707106781186548,-0.707106781186548,0.));
#33331=DIRECTION('ref_axis',(0.,0.,-1.));
#33332=DIRECTION('',(0.501874170540788,-0.864940643595846,-2.73831019897557E-14));
#33333=DIRECTION('center_axis',(0.,1.,0.));
#33334=DIRECTION('ref_axis',(0.,0.,1.));
#33335=DIRECTION('center_axis',(0.,1.,0.));
#33336=DIRECTION('ref_axis',(0.,0.,1.));
#33337=DIRECTION('',(0.,1.,0.));
#33338=DIRECTION('center_axis',(0.,0.,1.));
#33339=DIRECTION('ref_axis',(1.,0.,0.));
#33340=DIRECTION('center_axis',(0.,0.,1.));
#33341=DIRECTION('ref_axis',(1.,0.,0.));
#33342=DIRECTION('',(0.,0.,1.));
#33343=DIRECTION('center_axis',(0.,0.,1.));
#33344=DIRECTION('ref_axis',(1.,0.,0.));
#33345=DIRECTION('center_axis',(0.,-1.,0.));
#33346=DIRECTION('ref_axis',(0.,0.,1.));
#33347=DIRECTION('',(-8.65956056235501E-17,0.707106781186541,0.707106781186554));
#33348=DIRECTION('center_axis',(0.,0.,-1.));
#33349=DIRECTION('ref_axis',(1.,0.,0.));
#33350=DIRECTION('',(0.707106781186551,-8.65956056235498E-17,0.707106781186544));
#33351=DIRECTION('center_axis',(0.,0.,-1.));
#33352=DIRECTION('ref_axis',(1.,0.,0.));
#33353=DIRECTION('',(0.857167300702111,1.04972719113862E-16,0.515038074910056));
#33354=DIRECTION('center_axis',(0.707106781186548,0.707106781186548,0.));
#33355=DIRECTION('ref_axis',(0.,0.,-1.));
#33356=DIRECTION('',(0.,0.,-1.));
#33357=DIRECTION('',(-0.577350269189628,0.577350269189628,-0.577350269189622));
#33358=DIRECTION('center_axis',(0.707106781186548,0.707106781186548,0.));
#33359=DIRECTION('ref_axis',(0.,0.,-1.));
#33360=DIRECTION('',(0.,0.,-1.));
#33361=DIRECTION('center_axis',(1.,0.,0.));
#33362=DIRECTION('ref_axis',(0.,1.,0.));
#33363=DIRECTION('',(0.,0.,1.));
#33364=DIRECTION('',(0.,-1.,0.));
#33365=DIRECTION('center_axis',(1.,0.,0.));
#33366=DIRECTION('ref_axis',(0.,1.,0.));
#33367=DIRECTION('center_axis',(1.,0.,0.));
#33368=DIRECTION('ref_axis',(0.,1.,0.));
#33369=DIRECTION('center_axis',(1.,0.,0.));
#33370=DIRECTION('ref_axis',(0.,1.,0.));
#33371=DIRECTION('center_axis',(1.,0.,0.));
#33372=DIRECTION('ref_axis',(0.,1.,0.));
#33373=DIRECTION('center_axis',(1.,0.,0.));
#33374=DIRECTION('ref_axis',(0.,1.,0.));
#33375=DIRECTION('center_axis',(1.,0.,0.));
#33376=DIRECTION('ref_axis',(0.,1.,0.));
#33377=DIRECTION('center_axis',(0.707106781186548,-0.707106781186548,0.));
#33378=DIRECTION('ref_axis',(0.,0.,-1.));
#33379=DIRECTION('',(0.577350269189628,0.577350269189628,0.577350269189622));
#33380=DIRECTION('center_axis',(0.707106781186548,-0.707106781186548,0.));
#33381=DIRECTION('ref_axis',(0.,0.,-1.));
#33382=DIRECTION('center_axis',(0.707106781186548,-0.707106781186548,0.));
#33383=DIRECTION('ref_axis',(0.,0.,-1.));
#33384=DIRECTION('center_axis',(0.707106781186548,-0.707106781186548,0.));
#33385=DIRECTION('ref_axis',(0.,0.,-1.));
#33386=DIRECTION('center_axis',(0.,0.707106781186561,0.707106781186534));
#33387=DIRECTION('ref_axis',(1.,0.,0.));
#33388=DIRECTION('',(1.,0.,0.));
#33389=DIRECTION('',(0.577350269189618,0.577350269189618,-0.577350269189641));
#33390=DIRECTION('center_axis',(0.707106781186544,0.,-0.707106781186551));
#33391=DIRECTION('ref_axis',(-0.707106781186551,0.,-0.707106781186544));
#33392=DIRECTION('',(0.577350269189628,0.577350269189628,0.577350269189622));
#33393=DIRECTION('center_axis',(0.707106781186561,0.,0.707106781186534));
#33394=DIRECTION('ref_axis',(0.707106781186534,0.,-0.707106781186561));
#33395=DIRECTION('',(0.,-1.,0.));
#33396=DIRECTION('center_axis',(0.,0.707106781186544,-0.707106781186551));
#33397=DIRECTION('ref_axis',(-1.,0.,0.));
#33398=DIRECTION('center_axis',(0.,0.,1.));
#33399=DIRECTION('ref_axis',(1.,0.,0.));
#33400=DIRECTION('center_axis',(-1.,0.,0.));
#33401=DIRECTION('ref_axis',(0.,-1.,0.));
#60846=CARTESIAN_POINT('',(0.,0.,0.));
#60847=CARTESIAN_POINT('Origin',(4.42952305344106,-2.25,78.7389695278488));
#60848=CARTESIAN_POINT('',(4.42952305344106,4.42047694655894,78.7389695278488));
#60849=CARTESIAN_POINT('',(4.5,4.35,78.8396210385982));
#60850=CARTESIAN_POINT('',(1.84616051607008,7.00383948392992,75.04954546941));
#60851=CARTESIAN_POINT('',(4.5,-4.35,78.8396210385982));
#60852=CARTESIAN_POINT('',(4.5,-2.25,78.8396210385982));
#60853=CARTESIAN_POINT('',(4.42952305344105,-4.42047694655895,78.7389695278488));
#60854=CARTESIAN_POINT('',(1.2891756037128,-7.56082439628721,74.2540885770415));
#60855=CARTESIAN_POINT('',(4.35904610688211,-4.35,78.6383180170993));
#60856=CARTESIAN_POINT('',(2.71496575386869,-2.70591964698626,76.2903279380192));
#60857=CARTESIAN_POINT('',(4.35904610688211,4.35,78.6383180170993));
#60858=CARTESIAN_POINT('',(4.35904610688211,-2.25,78.6383180170993));
#60859=CARTESIAN_POINT('',(2.90546581342326,2.89641970654102,76.5623902183564));
#60860=CARTESIAN_POINT('Origin',(0.709236498419204,4.425,77.3897092918157));
#60861=CARTESIAN_POINT('',(3.15,4.35,78.1982612223388));
#60862=CARTESIAN_POINT('',(0.734888009168629,4.35,77.3192323452568));
#60863=CARTESIAN_POINT('',(3.,4.5,78.3032923530703));
#60864=CARTESIAN_POINT('',(4.07348426223018,3.42651573776982,77.5516305805072));
#60865=CARTESIAN_POINT('',(4.35,4.5,78.7946521693296));
#60866=CARTESIAN_POINT('',(0.683584987669779,4.5,77.4601862383747));
#60867=CARTESIAN_POINT('',(6.57988693089012,2.27011306910988,77.2332685309651));
#60868=CARTESIAN_POINT('Origin',(3.15,0.,78.1982612223388));
#60869=CARTESIAN_POINT('',(3.15,-4.35,78.1982612223388));
#60870=CARTESIAN_POINT('',(-3.23871198784907,-4.35,75.8729602234621));
#60871=CARTESIAN_POINT('',(3.15,0.,78.1982612223388));
#60872=CARTESIAN_POINT('Origin',(-3.26436349859849,-4.425,75.943437170021));
#60873=CARTESIAN_POINT('',(4.35,-4.5,78.7946521693296));
#60874=CARTESIAN_POINT('',(5.98539619974414,-2.86460380025586,77.6495354223095));
#60875=CARTESIAN_POINT('',(3.,-4.5,78.3032923530702));
#60876=CARTESIAN_POINT('',(-3.29001500934791,-4.5,76.01391411658));
#60877=CARTESIAN_POINT('',(3.,-4.5,78.3032923530702));
#60878=CARTESIAN_POINT('Origin',(4.42952305344106,-2.25,95.7035698572336));
#60879=CARTESIAN_POINT('',(4.42952305344105,4.42047694655895,95.7035698572336));
#60880=CARTESIAN_POINT('',(4.5,4.35,95.8042213679831));
#60881=CARTESIAN_POINT('',(-1.1526413191047,10.0026413191047,87.7314129352752));
#60882=CARTESIAN_POINT('',(4.5,-4.35,95.8042213679831));
#60883=CARTESIAN_POINT('',(4.5,-2.25,95.8042213679831));
#60884=CARTESIAN_POINT('',(4.42952305344106,-4.42047694655894,95.7035698572336));
#60885=CARTESIAN_POINT('',(-1.70962623146198,-10.559626231462,86.9359560429067));
#60886=CARTESIAN_POINT('',(4.35904610688212,-4.35,95.6029183464842));
#60887=CARTESIAN_POINT('',(2.2021404371328,-2.19309433025049,92.5225378135008));
#60888=CARTESIAN_POINT('',(4.35904610688211,4.35,95.6029183464842));
#60889=CARTESIAN_POINT('',(4.35904610688211,-2.25,95.6029183464842));
#60890=CARTESIAN_POINT('',(2.39264049668742,2.38359438980513,92.794600093838));
#60891=CARTESIAN_POINT('Origin',(-2.01692222533399,4.425,93.3620689918693));
#60892=CARTESIAN_POINT('',(3.15,4.35,95.1628615517237));
#60893=CARTESIAN_POINT('',(-1.99127071458457,4.35,93.2915920453104));
#60894=CARTESIAN_POINT('',(3.,4.5,95.2678926824551));
#60895=CARTESIAN_POINT('',(4.85812886689736,2.64187113310263,93.9668168428886));
#60896=CARTESIAN_POINT('',(4.35,4.5,95.7592524987145));
#60897=CARTESIAN_POINT('',(-2.04257373608342,4.5,93.4325459384283));
#60898=CARTESIAN_POINT('',(8.55703704573063,0.292962954269369,92.8134534457666));
#60899=CARTESIAN_POINT('Origin',(3.15,0.,95.1628615517237));
#60900=CARTESIAN_POINT('',(3.15,-4.35,95.1628615517237));
#60901=CARTESIAN_POINT('',(-5.96487071160227,-4.35,91.8453199235157));
#60902=CARTESIAN_POINT('',(3.15,0.,95.1628615517237));
#60903=CARTESIAN_POINT('Origin',(-5.99052222235169,-4.425,91.9157968700746));
#60904=CARTESIAN_POINT('',(4.35,-4.5,95.7592524987145));
#60905=CARTESIAN_POINT('',(7.96254631458501,-0.887453685414986,93.2297203371105));
#60906=CARTESIAN_POINT('',(3.,-4.5,95.2678926824551));
#60907=CARTESIAN_POINT('',(-6.01617373310111,-4.5,91.9862738166335));
#60908=CARTESIAN_POINT('',(3.,-4.5,95.2678926824551));
#60909=CARTESIAN_POINT('Origin',(4.42952305344106,-2.25,112.668170186619));
#60910=CARTESIAN_POINT('',(4.42952305344106,4.42047694655894,112.668170186619));
#60911=CARTESIAN_POINT('',(4.5,4.35,112.768821697368));
#60912=CARTESIAN_POINT('',(-4.15144315427948,13.0014431542795,100.41328040114));
#60913=CARTESIAN_POINT('',(4.5,-4.35,112.768821697368));
#60914=CARTESIAN_POINT('',(4.5,-2.25,112.768821697368));
#60915=CARTESIAN_POINT('',(4.42952305344106,-4.42047694655895,112.668170186619));
#60916=CARTESIAN_POINT('',(-4.70842806663676,-13.5584280666368,99.6178235087719));
#60917=CARTESIAN_POINT('',(4.35904610688211,-4.35,112.567518675869));
#60918=CARTESIAN_POINT('',(1.68931512039689,-1.68026901351456,108.754747688982));
#60919=CARTESIAN_POINT('',(4.35904610688211,4.35,112.567518675869));
#60920=CARTESIAN_POINT('',(4.35904610688211,-2.25,112.567518675869));
#60921=CARTESIAN_POINT('',(1.87981517995153,1.87076907306921,109.02680996932));
#60922=CARTESIAN_POINT('Origin',(3.15,0.,112.127461881109));
#60923=CARTESIAN_POINT('',(3.15,-4.35,112.127461881109));
#60924=CARTESIAN_POINT('',(-8.69102943535563,-4.35,107.817679623569));
#60925=CARTESIAN_POINT('',(3.15,4.35,112.127461881109));
#60926=CARTESIAN_POINT('',(3.15,0.,112.127461881109));
#60927=CARTESIAN_POINT('',(-4.71742943833795,4.35,109.263951745364));
#60928=CARTESIAN_POINT('Origin',(-8.71668094610505,-4.425,107.888156570128));
#60929=CARTESIAN_POINT('',(4.35,-4.5,112.723852828099));
#60930=CARTESIAN_POINT('',(9.93969642942553,1.08969642942552,108.809905251912));
#60931=CARTESIAN_POINT('',(3.,-4.5,112.23249301184));
#60932=CARTESIAN_POINT('',(-8.74233245685448,-4.5,107.958633516687));
#60933=CARTESIAN_POINT('',(3.,-4.5,112.23249301184));
#60934=CARTESIAN_POINT('Origin',(4.425,-4.425,59.4601776313845));
#60935=CARTESIAN_POINT('',(4.5,-4.35,112.974535212325));
#60936=CARTESIAN_POINT('',(4.5,-4.35,59.4601776313845));
#60937=CARTESIAN_POINT('',(4.42952305344105,-4.42047694655896,113.075186723075));
#60938=CARTESIAN_POINT('',(14.1744814719277,5.32448147192768,99.1579437819278));
#60939=CARTESIAN_POINT('',(4.35,-4.5,113.019504081594));
#60940=CARTESIAN_POINT('',(-2.40533103406217,-11.2553310340622,108.289370368442));
#60941=CARTESIAN_POINT('',(4.35,-4.5,59.4601776313845));
#60942=CARTESIAN_POINT('Origin',(4.42952305344106,-2.25,118.32303696308));
#60943=CARTESIAN_POINT('',(4.42952305344106,4.42047694655894,118.32303696308));
#60944=CARTESIAN_POINT('',(4.5,4.35,118.42368847383));
#60945=CARTESIAN_POINT('',(-5.1510437660044,14.0010437660044,104.640569556429));
#60946=CARTESIAN_POINT('',(4.5,-4.35,118.42368847383));
#60947=CARTESIAN_POINT('',(4.5,-2.25,118.42368847383));
#60948=CARTESIAN_POINT('',(4.42952305344105,-4.42047694655895,118.32303696308));
#60949=CARTESIAN_POINT('',(-5.70802867836169,-14.5580286783617,103.845112664061));
#60950=CARTESIAN_POINT('',(4.35904610688211,-4.35,118.222385452331));
#60951=CARTESIAN_POINT('',(1.51837334815156,-1.50932724126927,114.165484314143));
#60952=CARTESIAN_POINT('',(4.35904610688211,4.35,118.222385452331));
#60953=CARTESIAN_POINT('',(4.35904610688211,-2.25,118.222385452331));
#60954=CARTESIAN_POINT('',(1.70887340770616,1.69982730082414,114.43754659448));
#60955=CARTESIAN_POINT('Origin',(-5.6518005236718,4.425,114.658548591941));
#60956=CARTESIAN_POINT('',(3.15,4.35,117.78232865757));
#60957=CARTESIAN_POINT('',(-5.62614901292237,4.35,114.588071645382));
#60958=CARTESIAN_POINT('',(3.,4.5,117.887359788302));
#60959=CARTESIAN_POINT('',(5.90432167312078,1.5956783268792,115.853731859396));
#60960=CARTESIAN_POINT('',(4.35,4.5,118.378719604561));
#60961=CARTESIAN_POINT('',(-5.67745203442123,4.5,114.7290255385));
#60962=CARTESIAN_POINT('',(11.1932371988523,-2.34323719885225,113.587033332167));
#60963=CARTESIAN_POINT('Origin',(3.15,0.,117.78232865757));
#60964=CARTESIAN_POINT('',(3.15,-4.35,117.78232865757));
#60965=CARTESIAN_POINT('',(-9.59974900994005,-4.35,113.141799523587));
#60966=CARTESIAN_POINT('',(3.15,0.,117.78232865757));
#60967=CARTESIAN_POINT('Origin',(-9.62540052068947,-4.425,113.212276470146));
#60968=CARTESIAN_POINT('',(4.35,-4.5,118.378719604561));
#60969=CARTESIAN_POINT('',(10.5987464677057,1.74874646770573,114.003300223512));
#60970=CARTESIAN_POINT('',(3.,-4.5,117.887359788302));
#60971=CARTESIAN_POINT('',(-9.6510520314389,-4.5,113.282753416705));
#60972=CARTESIAN_POINT('',(3.,-4.5,117.887359788302));
#60973=CARTESIAN_POINT('Origin',(4.42952305344106,-2.25,99.4734810415414));
#60974=CARTESIAN_POINT('',(4.42952305344106,4.42047694655894,99.4734810415414));
#60975=CARTESIAN_POINT('',(4.5,4.35,99.5741325522908));
#60976=CARTESIAN_POINT('',(-1.81904172692132,10.6690417269213,90.5496057054675));
#60977=CARTESIAN_POINT('',(4.5,-4.35,99.5741325522908));
#60978=CARTESIAN_POINT('',(4.5,-2.25,99.5741325522908));
#60979=CARTESIAN_POINT('',(4.42952305344106,-4.42047694655894,99.4734810415414));
#60980=CARTESIAN_POINT('',(-2.3760266392786,-11.2260266392786,89.754148813099));
#60981=CARTESIAN_POINT('',(4.35904610688212,-4.35,99.372829530792));
#60982=CARTESIAN_POINT('',(2.08817925563595,-2.07913314875362,96.1296955636079));
#60983=CARTESIAN_POINT('',(4.35904610688211,4.35,99.372829530792));
#60984=CARTESIAN_POINT('',(4.35904610688211,-2.25,99.372829530792));
#60985=CARTESIAN_POINT('',(2.27867931519057,2.26963320830827,96.4017578439451));
#60986=CARTESIAN_POINT('Origin',(4.5,-4.5,59.4601776313845));
#60987=CARTESIAN_POINT('',(4.5,4.35,99.7798460672483));
#60988=CARTESIAN_POINT('',(4.5,4.35,59.4601776313845));
#60989=CARTESIAN_POINT('',(4.5,-4.35,99.7798460672483));
#60990=CARTESIAN_POINT('',(4.5,-2.25,99.7798460672483));
#60991=CARTESIAN_POINT('',(4.5,-4.35,59.4601776313845));
#60992=CARTESIAN_POINT('Origin',(4.425,4.425,59.4601776313845));
#60993=CARTESIAN_POINT('',(4.35,4.5,99.5291636830223));
#60994=CARTESIAN_POINT('',(8.99640373791744,-0.146403737917441,96.2757167601669));
#60995=CARTESIAN_POINT('',(4.35,4.5,99.8248149365169));
#60996=CARTESIAN_POINT('',(4.35,4.5,59.4601776313845));
#60997=CARTESIAN_POINT('',(4.42952305344105,4.42047694655895,99.8804975779977));
#60998=CARTESIAN_POINT('',(-0.273056880261707,9.12305688026171,96.5877156593865));
#60999=CARTESIAN_POINT('',(12.3990649569269,-3.54906495692689,88.4988121938873));
#61000=CARTESIAN_POINT('Origin',(-2.62273527505693,4.425,96.9114822585479));
#61001=CARTESIAN_POINT('',(3.15,4.35,98.9327727360315));
#61002=CARTESIAN_POINT('',(-2.5970837643075,4.35,96.841005311989));
#61003=CARTESIAN_POINT('',(3.,4.5,99.0378038667629));
#61004=CARTESIAN_POINT('',(3.15,4.35,98.9327727360315));
#61005=CARTESIAN_POINT('',(-2.64838678580635,4.5,96.9819592051068));
#61006=CARTESIAN_POINT('Origin',(4.42952305344106,-2.25,97.9955419858439));
#61007=CARTESIAN_POINT('',(4.42952305344105,-4.42047694655895,97.9955419858439));
#61008=CARTESIAN_POINT('',(4.5,-4.35,97.8948904750944));
#61009=CARTESIAN_POINT('',(11.5088798406612,2.65887984066121,87.8851727011587));
#61010=CARTESIAN_POINT('',(4.5,4.35,97.8948904750944));
#61011=CARTESIAN_POINT('',(4.5,-2.25,97.8948904750944));
#61012=CARTESIAN_POINT('',(4.42952305344105,4.42047694655894,97.9955419858439));
#61013=CARTESIAN_POINT('',(12.0658647530185,-3.2158647530185,87.0897158087902));
#61014=CARTESIAN_POINT('',(4.35904610688211,4.35,98.0961934965933));
#61015=CARTESIAN_POINT('',(4.78481711861775,4.77577101173567,97.4881294748544));
#61016=CARTESIAN_POINT('',(4.35904610688211,-4.35,98.0961934965933));
#61017=CARTESIAN_POINT('',(4.35904610688211,-2.25,98.0961934965933));
#61018=CARTESIAN_POINT('',(4.59431705906312,-4.58527095218102,97.7601917551917));
#61019=CARTESIAN_POINT('Origin',(10.699792324063,4.425,95.7085372775677));
#61020=CARTESIAN_POINT('',(4.35,4.5,97.939859344363));
#61021=CARTESIAN_POINT('',(-0.0533735341695696,8.90337353416957,94.8565840021845));
#61022=CARTESIAN_POINT('',(3.,4.5,98.4312191606224));
#61023=CARTESIAN_POINT('',(10.6741408133136,4.5,95.6380603310088));
#61024=CARTESIAN_POINT('',(3.15,4.35,98.5362502913538));
#61025=CARTESIAN_POINT('',(3.15,4.35,98.5362502913538));
#61026=CARTESIAN_POINT('',(10.7254438348125,4.35,95.7790142241267));
#61027=CARTESIAN_POINT('Origin',(4.425,4.425,59.4601776313845));
#61028=CARTESIAN_POINT('',(4.5,4.35,97.689176960137));
#61029=CARTESIAN_POINT('',(4.5,4.35,59.4601776313845));
#61030=CARTESIAN_POINT('',(4.42952305344105,4.42047694655894,97.5885254493875));
#61031=CARTESIAN_POINT('',(-1.48584152301308,10.3358415230131,89.1405093203705));
#61032=CARTESIAN_POINT('',(4.35,4.5,97.6442080908684));
#61033=CARTESIAN_POINT('',(8.77672039182401,0.0732796081759872,94.5445851029668));
#61034=CARTESIAN_POINT('',(4.35,4.5,59.4601776313845));
#61035=CARTESIAN_POINT('Origin',(4.5,-4.5,59.4601776313845));
#61036=CARTESIAN_POINT('',(4.5,-4.35,97.689176960137));
#61037=CARTESIAN_POINT('',(4.5,-4.35,59.4601776313845));
#61038=CARTESIAN_POINT('',(4.5,-2.25,97.689176960137));
#61039=CARTESIAN_POINT('Origin',(4.42952305344106,-2.25,97.5885254493875));
#61040=CARTESIAN_POINT('',(4.42952305344106,-4.42047694655894,97.5885254493875));
#61041=CARTESIAN_POINT('',(-2.04282643537031,-10.8928264353703,88.3450524280019));
#61042=CARTESIAN_POINT('',(4.35904610688211,-4.35,97.4878739386381));
#61043=CARTESIAN_POINT('',(2.14515984638464,-2.13611373950202,94.3261166885544));
#61044=CARTESIAN_POINT('',(4.35904610688212,4.35,97.4878739386381));
#61045=CARTESIAN_POINT('',(4.35904610688212,-2.25,97.4878739386381));
#61046=CARTESIAN_POINT('',(2.33565990593919,2.3266137990566,94.5981789688915));
#61047=CARTESIAN_POINT('Origin',(-2.31982875019547,4.425,95.1367756252086));
#61048=CARTESIAN_POINT('',(3.15,4.35,97.0478171438776));
#61049=CARTESIAN_POINT('',(-2.29417723944604,4.35,95.0662986786497));
#61050=CARTESIAN_POINT('',(3.,4.5,97.152848274609));
#61051=CARTESIAN_POINT('',(3.15,4.35,97.0478171438776));
#61052=CARTESIAN_POINT('',(-2.34548026094489,4.5,95.2072525717676));
#61053=CARTESIAN_POINT('Origin',(4.42952305344106,-2.25,96.11058639369));
#61054=CARTESIAN_POINT('',(4.42952305344106,-4.42047694655894,96.11058639369));
#61055=CARTESIAN_POINT('',(4.5,-4.35,96.0099348829406));
#61056=CARTESIAN_POINT('',(11.1756796367529,2.3256796367529,86.4760763160626));
#61057=CARTESIAN_POINT('',(4.5,4.35,96.0099348829406));
#61058=CARTESIAN_POINT('',(4.5,-2.25,96.0099348829406));
#61059=CARTESIAN_POINT('',(4.42952305344105,4.42047694655895,96.11058639369));
#61060=CARTESIAN_POINT('',(11.7326645491102,-2.88266454911019,85.680619423694));
#61061=CARTESIAN_POINT('',(4.35904610688211,4.35,96.2112379044394));
#61062=CARTESIAN_POINT('',(4.72783652786931,4.71879042098724,95.6845505998009));
#61063=CARTESIAN_POINT('',(4.35904610688211,-4.35,96.2112379044394));
#61064=CARTESIAN_POINT('',(4.35904610688211,-2.25,96.2112379044394));
#61065=CARTESIAN_POINT('',(4.53733646831466,-4.52829036143257,95.9566128801382));
#61066=CARTESIAN_POINT('Origin',(4.55,0.,96.1417363712273));
#61067=CARTESIAN_POINT('',(3.15,4.35,96.6512946992));
#61068=CARTESIAN_POINT('',(10.422537309951,4.35,94.0043075907874));
#61069=CARTESIAN_POINT('',(3.15,-4.35,96.6512946992));
#61070=CARTESIAN_POINT('',(3.15,0.,96.6512946992));
#61071=CARTESIAN_POINT('',(6.44893731293329,-4.35,95.4505797125821));
#61072=CARTESIAN_POINT('Origin',(10.3968857992016,4.425,93.9338306442285));
#61073=CARTESIAN_POINT('',(4.35,4.5,96.0549037522091));
#61074=CARTESIAN_POINT('',(0.16630981192384,8.68369018807616,93.1254523449844));
#61075=CARTESIAN_POINT('',(3.,4.5,96.5462635684685));
#61076=CARTESIAN_POINT('',(10.3712342884521,4.5,93.8633536976695));
#61077=CARTESIAN_POINT('',(3.15,4.35,96.6512946992));
#61078=CARTESIAN_POINT('Origin',(4.425,4.425,59.4601776313845));
#61079=CARTESIAN_POINT('',(4.35,4.5,59.4601776313845));
#61080=CARTESIAN_POINT('',(4.5,4.35,59.4601776313845));
#61081=CARTESIAN_POINT('Origin',(4.42952305344105,-2.25,82.5088807121565));
#61082=CARTESIAN_POINT('',(4.42952305344105,4.42047694655895,82.5088807121565));
#61083=CARTESIAN_POINT('',(4.5,4.35,82.6095322229059));
#61084=CARTESIAN_POINT('',(1.17976010825354,7.67023989174646,77.8677382396028));
#61085=CARTESIAN_POINT('',(4.5,-4.35,82.6095322229059));
#61086=CARTESIAN_POINT('',(4.5,-2.25,82.6095322229059));
#61087=CARTESIAN_POINT('',(4.42952305344105,-4.42047694655895,82.5088807121565));
#61088=CARTESIAN_POINT('',(0.622775195896197,-8.2272248041038,77.0722813472343));
#61089=CARTESIAN_POINT('',(4.35904610688211,-4.35,82.4082292014071));
#61090=CARTESIAN_POINT('',(2.60100457237156,-2.59195846548954,79.8974856881262));
#61091=CARTESIAN_POINT('',(4.35904610688211,4.35,82.4082292014071));
#61092=CARTESIAN_POINT('',(4.35904610688211,-2.25,82.4082292014071));
#61093=CARTESIAN_POINT('',(2.79150463192627,2.78245852504406,80.1695479684634));
#61094=CARTESIAN_POINT('Origin',(4.5,-4.5,59.4601776313845));
#61095=CARTESIAN_POINT('',(4.5,4.35,82.8152457378634));
#61096=CARTESIAN_POINT('',(4.5,4.35,59.4601776313845));
#61097=CARTESIAN_POINT('',(4.5,-4.35,82.8152457378634));
#61098=CARTESIAN_POINT('',(4.5,-2.25,82.8152457378634));
#61099=CARTESIAN_POINT('',(4.5,-4.35,59.4601776313845));
#61100=CARTESIAN_POINT('Origin',(4.425,4.425,59.4601776313845));
#61101=CARTESIAN_POINT('',(4.35,4.5,82.5645633536374));
#61102=CARTESIAN_POINT('',(7.0192536230765,1.8307463769235,80.695531845366));
#61103=CARTESIAN_POINT('',(4.35,4.5,82.860214607132));
#61104=CARTESIAN_POINT('',(4.35,4.5,59.4601776313845));
#61105=CARTESIAN_POINT('',(4.42952305344106,4.42047694655894,82.9158972486129));
#61106=CARTESIAN_POINT('',(1.70409323457756,7.14590676542244,81.0075307445832));
#61107=CARTESIAN_POINT('',(9.40026312175203,-0.550263121752025,75.8169447280211));
#61108=CARTESIAN_POINT('Origin',(0.103423448696272,4.425,80.9391225584943));
#61109=CARTESIAN_POINT('',(3.15,4.35,81.9681724066466));
#61110=CARTESIAN_POINT('',(0.129074959445692,4.35,80.8686456119354));
#61111=CARTESIAN_POINT('',(3.,4.5,82.073203537378));
#61112=CARTESIAN_POINT('',(3.15,4.35,81.9681724066466));
#61113=CARTESIAN_POINT('',(0.0777719379468511,4.5,81.0095995050532));
#61114=CARTESIAN_POINT('Origin',(4.42952305344106,-2.25,81.030941656459));
#61115=CARTESIAN_POINT('',(4.42952305344105,-4.42047694655895,81.030941656459));
#61116=CARTESIAN_POINT('',(4.5,-4.35,80.9302901457095));
#61117=CARTESIAN_POINT('',(8.51007800548643,-0.339921994513569,75.2033052352935));
#61118=CARTESIAN_POINT('',(4.5,4.35,80.9302901457095));
#61119=CARTESIAN_POINT('',(4.5,-2.25,80.9302901457095));
#61120=CARTESIAN_POINT('',(4.42952305344106,4.42047694655894,81.030941656459));
#61121=CARTESIAN_POINT('',(9.06706291784371,-0.217062917843715,74.4078483429249));
#61122=CARTESIAN_POINT('',(4.35904610688211,4.35,81.1315931672084));
#61123=CARTESIAN_POINT('',(4.2719918018819,4.26294569499977,81.2559195993728));
#61124=CARTESIAN_POINT('',(4.35904610688212,-4.35,81.1315931672084));
#61125=CARTESIAN_POINT('',(4.35904610688211,-2.25,81.1315931672084));
#61126=CARTESIAN_POINT('',(4.08149174232726,-4.07244563544511,81.52798187971));
#61127=CARTESIAN_POINT('Origin',(7.97363360030984,4.425,79.7361775775141));
#61128=CARTESIAN_POINT('',(4.35,4.5,80.9752590149781));
#61129=CARTESIAN_POINT('',(1.92377658067096,6.92622341932904,79.2763990873831));
#61130=CARTESIAN_POINT('',(3.,4.5,81.4666188312375));
#61131=CARTESIAN_POINT('',(7.94798208956041,4.5,79.6657006309552));
#61132=CARTESIAN_POINT('',(3.15,4.35,81.5716499619689));
#61133=CARTESIAN_POINT('',(3.15,4.35,81.5716499619689));
#61134=CARTESIAN_POINT('',(7.99928511105926,4.35,79.8066545240731));
#61135=CARTESIAN_POINT('Origin',(4.425,4.425,59.4601776313845));
#61136=CARTESIAN_POINT('',(4.5,4.35,80.7245766307521));
#61137=CARTESIAN_POINT('',(4.5,4.35,59.4601776313845));
#61138=CARTESIAN_POINT('',(4.42952305344105,4.42047694655894,80.6239251200027));
#61139=CARTESIAN_POINT('',(1.51296031216177,7.33703968783823,76.4586418545061));
#61140=CARTESIAN_POINT('',(4.35,4.5,80.6796077614835));
#61141=CARTESIAN_POINT('',(6.7995702769835,2.0504297230165,78.9644001881653));
#61142=CARTESIAN_POINT('',(4.35,4.5,59.4601776313845));
#61143=CARTESIAN_POINT('Origin',(4.5,-4.5,59.4601776313845));
#61144=CARTESIAN_POINT('',(4.5,-4.35,80.7245766307521));
#61145=CARTESIAN_POINT('',(4.5,-4.35,59.4601776313845));
#61146=CARTESIAN_POINT('',(4.5,-2.25,80.7245766307521));
#61147=CARTESIAN_POINT('Origin',(4.42952305344106,-2.25,80.6239251200027));
#61148=CARTESIAN_POINT('',(4.42952305344105,-4.42047694655895,80.6239251200026));
#61149=CARTESIAN_POINT('',(0.955975399804484,-7.89402460019551,75.6631849621376));
#61150=CARTESIAN_POINT('',(4.35904610688211,-4.35,80.5232736092532));
#61151=CARTESIAN_POINT('',(2.65798516312021,-2.64893905623794,78.0939068130727));
#61152=CARTESIAN_POINT('',(4.35904610688211,4.35,80.5232736092532));
#61153=CARTESIAN_POINT('',(4.35904610688211,-2.25,80.5232736092532));
#61154=CARTESIAN_POINT('',(2.84848522267484,2.83943911579257,78.3659690934099));
#61155=CARTESIAN_POINT('Origin',(0.406329973557735,4.425,79.164415925155));
#61156=CARTESIAN_POINT('',(3.15,4.35,80.0832168144927));
#61157=CARTESIAN_POINT('',(0.431981484307159,4.35,79.0939389785961));
#61158=CARTESIAN_POINT('',(3.,4.5,80.1882479452241));
#61159=CARTESIAN_POINT('',(3.15,4.35,80.0832168144927));
#61160=CARTESIAN_POINT('',(0.380678462808311,4.5,79.234892871714));
#61161=CARTESIAN_POINT('Origin',(4.42952305344106,-2.25,79.1459860643051));
#61162=CARTESIAN_POINT('',(4.42952305344106,-4.42047694655894,79.1459860643051));
#61163=CARTESIAN_POINT('',(4.5,-4.35,79.0453345535557));
#61164=CARTESIAN_POINT('',(8.17687780157812,-0.673122198421876,73.7942088501973));
#61165=CARTESIAN_POINT('',(4.5,4.35,79.0453345535557));
#61166=CARTESIAN_POINT('',(4.5,-2.25,79.0453345535557));
#61167=CARTESIAN_POINT('',(4.42952305344106,4.42047694655894,79.1459860643051));
#61168=CARTESIAN_POINT('',(8.73386271393541,0.116137286064592,72.9987519578288));
#61169=CARTESIAN_POINT('',(4.35904610688211,4.35,79.2466375750545));
#61170=CARTESIAN_POINT('',(4.21501121113347,4.20596510425134,79.4523407243193));
#61171=CARTESIAN_POINT('',(4.35904610688211,-4.35,79.2466375750545));
#61172=CARTESIAN_POINT('',(4.35904610688211,-2.25,79.2466375750545));
#61173=CARTESIAN_POINT('',(4.02451115157885,-4.0154650446967,79.7244030046565));
#61174=CARTESIAN_POINT('Origin',(4.55,0.,79.1771360418424));
#61175=CARTESIAN_POINT('',(3.15,4.35,79.6866943698151));
#61176=CARTESIAN_POINT('',(7.69637858619779,4.35,78.0319478907338));
#61177=CARTESIAN_POINT('',(3.15,-4.35,79.6866943698151));
#61178=CARTESIAN_POINT('',(3.15,0.,79.6866943698151));
#61179=CARTESIAN_POINT('',(3.7227785891801,-4.35,79.4782200125285));
#61180=CARTESIAN_POINT('Origin',(7.67072707544837,4.425,77.9614709441749));
#61181=CARTESIAN_POINT('',(4.35,4.5,79.0903034228242));
#61182=CARTESIAN_POINT('',(2.14345992676436,6.70654007323564,77.5452674301829));
#61183=CARTESIAN_POINT('',(3.,4.5,79.5816632390836));
#61184=CARTESIAN_POINT('',(7.64507556469895,4.5,77.8909939976159));
#61185=CARTESIAN_POINT('',(3.15,4.35,79.6866943698151));
#61186=CARTESIAN_POINT('Origin',(4.425,4.425,59.4601776313845));
#61187=CARTESIAN_POINT('',(4.35,4.5,59.4601776313845));
#61188=CARTESIAN_POINT('',(4.5,4.35,59.4601776313845));
#61189=CARTESIAN_POINT('Origin',(4.42952305344106,-2.25,77.2610304721512));
#61190=CARTESIAN_POINT('',(4.42952305344106,-4.42047694655894,77.2610304721512));
#61191=CARTESIAN_POINT('',(4.5,-4.35,77.1603789614018));
#61192=CARTESIAN_POINT('',(7.84367759766981,-1.00632240233019,72.3851124651012));
#61193=CARTESIAN_POINT('',(4.5,4.35,77.1603789614018));
#61194=CARTESIAN_POINT('',(4.5,-2.25,77.1603789614018));
#61195=CARTESIAN_POINT('',(4.42952305344106,4.42047694655894,77.2610304721512));
#61196=CARTESIAN_POINT('',(8.4006625100271,0.449337489972902,71.5896555727327));
#61197=CARTESIAN_POINT('',(4.35904610688211,4.35,77.3616819829007));
#61198=CARTESIAN_POINT('',(4.15803062038505,4.14898451350291,77.6487618492658));
#61199=CARTESIAN_POINT('',(4.35904610688211,-4.35,77.3616819829007));
#61200=CARTESIAN_POINT('',(4.35904610688211,-2.25,77.3616819829007));
#61201=CARTESIAN_POINT('',(3.96753056083043,-3.95848445394826,77.920824129603));
#61202=CARTESIAN_POINT('Origin',(7.36782055058691,4.425,76.1867643108356));
#61203=CARTESIAN_POINT('',(4.35,4.5,77.2053478306703));
#61204=CARTESIAN_POINT('',(2.36314327285774,6.48685672714226,75.8141357729827));
#61205=CARTESIAN_POINT('',(3.,4.5,77.6967076469297));
#61206=CARTESIAN_POINT('',(7.34216903983748,4.5,76.1162873642766));
#61207=CARTESIAN_POINT('',(3.15,4.35,77.8017387776612));
#61208=CARTESIAN_POINT('',(3.15,4.35,77.8017387776612));
#61209=CARTESIAN_POINT('',(7.39347206133633,4.35,76.2572412573945));
#61210=CARTESIAN_POINT('Origin',(4.425,4.425,59.4601776313845));
#61211=CARTESIAN_POINT('',(4.5,4.35,76.9546654464443));
#61212=CARTESIAN_POINT('',(4.5,4.35,59.4601776313845));
#61213=CARTESIAN_POINT('',(4.42952305344105,4.42047694655895,76.8540139356949));
#61214=CARTESIAN_POINT('',(2.17936071997847,6.67063928002153,73.6404490843143));
#61215=CARTESIAN_POINT('',(4.35,4.5,76.9096965771758));
#61216=CARTESIAN_POINT('',(6.36020358479645,2.48979641520355,75.5021368737654));
#61217=CARTESIAN_POINT('',(4.35,4.5,59.4601776313845));
#61218=CARTESIAN_POINT('Origin',(4.5,-4.5,59.4601776313845));
#61219=CARTESIAN_POINT('',(4.5,-4.35,76.9546654464443));
#61220=CARTESIAN_POINT('',(4.5,-4.35,59.4601776313845));
#61221=CARTESIAN_POINT('',(4.5,-2.25,76.9546654464443));
#61222=CARTESIAN_POINT('Origin',(4.42952305344105,-2.25,76.8540139356949));
#61223=CARTESIAN_POINT('',(4.42952305344106,-4.42047694655894,76.8540139356949));
#61224=CARTESIAN_POINT('',(1.62237580762112,-7.22762419237888,72.8449921919458));
#61225=CARTESIAN_POINT('',(4.35904610688211,-4.35,76.7533624249455));
#61226=CARTESIAN_POINT('',(2.77194634461692,-2.76290023773472,74.4867490629657));
#61227=CARTESIAN_POINT('',(4.35904610688211,4.35,76.7533624249455));
#61228=CARTESIAN_POINT('',(4.35904610688211,-2.25,76.7533624249455));
#61229=CARTESIAN_POINT('',(2.96244640417157,2.95340029728938,74.7588113433029));
#61230=CARTESIAN_POINT('Origin',(1.01214302328067,4.425,75.6150026584765));
#61231=CARTESIAN_POINT('',(3.15,4.35,76.3133056301849));
#61232=CARTESIAN_POINT('',(1.0377945340301,4.35,75.5445257119175));
#61233=CARTESIAN_POINT('',(3.,4.5,76.4183367609164));
#61234=CARTESIAN_POINT('',(3.15,4.35,76.3133056301849));
#61235=CARTESIAN_POINT('',(0.986491512531251,4.5,75.6854796050354));
#61236=CARTESIAN_POINT('Origin',(4.42952305344106,-2.25,75.3760748799974));
#61237=CARTESIAN_POINT('',(4.42952305344106,-4.42047694655894,75.3760748799974));
#61238=CARTESIAN_POINT('',(4.5,-4.35,75.2754233692479));
#61239=CARTESIAN_POINT('',(7.51047739376151,-1.33952260623849,70.9760160800051));
#61240=CARTESIAN_POINT('',(4.5,4.35,75.2754233692479));
#61241=CARTESIAN_POINT('',(4.5,-2.25,75.2754233692479));
#61242=CARTESIAN_POINT('',(4.42952305344105,4.42047694655895,75.3760748799974));
#61243=CARTESIAN_POINT('',(8.06746230611879,0.782537693881209,70.1805591876365));
#61244=CARTESIAN_POINT('',(4.35904610688211,4.35,75.4767263907468));
#61245=CARTESIAN_POINT('',(4.10105002963662,4.09200392275448,75.8451829742122));
#61246=CARTESIAN_POINT('',(4.35904610688211,-4.35,75.4767263907468));
#61247=CARTESIAN_POINT('',(4.35904610688211,-2.25,75.4767263907468));
#61248=CARTESIAN_POINT('',(3.910549970082,-3.90150386319978,76.1172452545494));
#61249=CARTESIAN_POINT('Origin',(4.55,0.,75.4072248575346));
#61250=CARTESIAN_POINT('',(3.15,4.35,75.9167831855073));
#61251=CARTESIAN_POINT('',(7.09056553647487,4.35,74.4825346240552));
#61252=CARTESIAN_POINT('',(3.15,-4.35,75.9167831855073));
#61253=CARTESIAN_POINT('',(3.15,0.,75.9167831855073));
#61254=CARTESIAN_POINT('',(3.11696553945717,-4.35,75.9288067458499));
#61255=CARTESIAN_POINT('Origin',(7.06491402572544,4.425,74.4120576774963));
#61256=CARTESIAN_POINT('',(4.35,4.5,75.3203922385165));
#61257=CARTESIAN_POINT('',(2.58282661895114,6.26717338104886,74.0830041157826));
#61258=CARTESIAN_POINT('',(3.,4.5,75.8117520547759));
#61259=CARTESIAN_POINT('',(7.03926251497602,4.5,74.3415807309374));
#61260=CARTESIAN_POINT('',(3.15,4.35,75.9167831855073));
#61261=CARTESIAN_POINT('Origin',(4.425,4.425,59.4601776313845));
#61262=CARTESIAN_POINT('',(4.5,4.35,75.0697098542905));
#61263=CARTESIAN_POINT('',(4.5,4.35,59.4601776313845));
#61264=CARTESIAN_POINT('',(4.42952305344105,4.42047694655895,74.969058343541));
#61265=CARTESIAN_POINT('',(2.51256092388669,6.33743907611331,72.2313526992177));
#61266=CARTESIAN_POINT('',(4.35,4.5,75.0247409850219));
#61267=CARTESIAN_POINT('',(6.14052023870333,2.70947976129667,73.7710052165648));
#61268=CARTESIAN_POINT('',(4.35,4.5,59.4601776313845));
#61269=CARTESIAN_POINT('Origin',(4.42952305344106,-2.25,74.969058343541));
#61270=CARTESIAN_POINT('',(4.5,-4.35,75.0697098542905));
#61271=CARTESIAN_POINT('',(4.5,-2.25,75.0697098542905));
#61272=CARTESIAN_POINT('',(4.42952305344106,-4.42047694655895,74.969058343541));
#61273=CARTESIAN_POINT('',(1.95557601152941,-6.89442398847059,71.4358958068492));
#61274=CARTESIAN_POINT('',(4.35904610688211,-4.35,74.8684068327916));
#61275=CARTESIAN_POINT('',(2.8289269353655,-2.81988082848323,72.6831701879121));
#61276=CARTESIAN_POINT('',(4.35904610688211,4.35,74.8684068327916));
#61277=CARTESIAN_POINT('',(4.35904610688211,-2.25,74.8684068327916));
#61278=CARTESIAN_POINT('',(3.01942699492011,3.01038088803788,72.9552324682493));
#61279=CARTESIAN_POINT('Origin',(3.15,0.,74.4283500380311));
#61280=CARTESIAN_POINT('',(3.15,-4.35,74.4283500380311));
#61281=CARTESIAN_POINT('',(-2.63289893812614,-4.35,72.3235469567835));
#61282=CARTESIAN_POINT('',(3.15,4.35,74.4283500380311));
#61283=CARTESIAN_POINT('',(3.15,0.,74.4283500380311));
#61284=CARTESIAN_POINT('',(1.34070105889156,4.35,73.7698190785782));
#61285=CARTESIAN_POINT('Origin',(-2.65855044887556,-4.425,72.3940239033425));
#61286=CARTESIAN_POINT('',(4.35,-4.5,75.0247409850219));
#61287=CARTESIAN_POINT('',(5.54602950755777,-3.30397049244223,74.1872721079087));
#61288=CARTESIAN_POINT('',(3.,-4.5,74.5333811687625));
#61289=CARTESIAN_POINT('',(-2.68420195962499,-4.5,72.4645008499014));
#61290=CARTESIAN_POINT('',(3.,-4.5,74.5333811687625));
#61291=CARTESIAN_POINT('Origin',(4.425,-4.425,59.4601776313845));
#61292=CARTESIAN_POINT('',(4.35,-4.5,75.3203922385165));
#61293=CARTESIAN_POINT('',(1.98833588780573,-6.86166411219427,73.666737224439));
#61294=CARTESIAN_POINT('',(4.35,-4.5,59.4601776313845));
#61295=CARTESIAN_POINT('',(4.5,-4.35,59.4601776313845));
#61296=CARTESIAN_POINT('Origin',(4.42952305344106,-2.25,73.4911192878435));
#61297=CARTESIAN_POINT('',(4.42952305344106,-4.42047694655894,73.4911192878435));
#61298=CARTESIAN_POINT('',(4.5,-4.35,73.390467777094));
#61299=CARTESIAN_POINT('',(7.1772771898532,-1.6727228101468,69.5669196949089));
#61300=CARTESIAN_POINT('',(4.5,4.35,73.390467777094));
#61301=CARTESIAN_POINT('',(4.5,-2.25,73.390467777094));
#61302=CARTESIAN_POINT('',(4.42952305344105,4.42047694655895,73.4911192878435));
#61303=CARTESIAN_POINT('',(7.73426210221048,1.11573789778952,68.7714628025404));
#61304=CARTESIAN_POINT('',(4.35904610688211,4.35,73.5917707985929));
#61305=CARTESIAN_POINT('',(4.04406943888819,4.03502333200606,74.0416040991587));
#61306=CARTESIAN_POINT('',(4.35904610688211,-4.35,73.5917707985929));
#61307=CARTESIAN_POINT('',(4.35904610688211,-2.25,73.5917707985929));
#61308=CARTESIAN_POINT('',(3.85356937933357,-3.84452327245141,74.3136663794959));
#61309=CARTESIAN_POINT('Origin',(6.76200750086397,4.425,72.637351044157));
#61310=CARTESIAN_POINT('',(4.35,4.5,73.4354366463626));
#61311=CARTESIAN_POINT('',(2.80250996504453,6.04749003495547,72.3518724585824));
#61312=CARTESIAN_POINT('',(3.,4.5,73.926796462622));
#61313=CARTESIAN_POINT('',(6.73635599011455,4.5,72.5668740975981));
#61314=CARTESIAN_POINT('',(3.15,4.35,74.0318275933534));
#61315=CARTESIAN_POINT('',(3.15,4.35,74.0318275933534));
#61316=CARTESIAN_POINT('',(6.78765901161339,4.35,72.7078279907159));
#61317=CARTESIAN_POINT('Origin',(4.425,4.425,59.4601776313845));
#61318=CARTESIAN_POINT('',(4.5,4.35,73.1847542621366));
#61319=CARTESIAN_POINT('',(4.5,4.35,59.4601776313845));
#61320=CARTESIAN_POINT('',(4.42952305344106,4.42047694655894,73.0841027513871));
#61321=CARTESIAN_POINT('',(2.845761127795,6.004238872205,70.8222563141216));
#61322=CARTESIAN_POINT('',(4.35,4.5,73.139785392868));
#61323=CARTESIAN_POINT('',(5.92083689260995,2.92916310739005,72.0398735593647));
#61324=CARTESIAN_POINT('',(4.35,4.5,59.4601776313845));
#61325=CARTESIAN_POINT('Origin',(4.5,-4.5,59.4601776313845));
#61326=CARTESIAN_POINT('',(4.5,-4.35,73.1847542621366));
#61327=CARTESIAN_POINT('',(4.5,-4.35,59.4601776313845));
#61328=CARTESIAN_POINT('',(4.5,-2.25,73.1847542621366));
#61329=CARTESIAN_POINT('Origin',(4.42952305344106,-2.25,73.0841027513871));
#61330=CARTESIAN_POINT('',(4.42952305344106,-4.42047694655894,73.0841027513872));
#61331=CARTESIAN_POINT('',(2.28877621543772,-6.56122378456228,70.0267994217531));
#61332=CARTESIAN_POINT('',(4.35904610688211,-4.35,72.9834512406377));
#61333=CARTESIAN_POINT('',(2.88590752611388,-2.87686141923176,70.8795913128586));
#61334=CARTESIAN_POINT('',(4.35904610688211,4.35,72.9834512406377));
#61335=CARTESIAN_POINT('',(4.35904610688211,-2.25,72.9834512406377));
#61336=CARTESIAN_POINT('',(3.07640758566854,3.06736147878631,71.1516535931958));
#61337=CARTESIAN_POINT('Origin',(1.6179560730036,4.425,72.0655893917979));
#61338=CARTESIAN_POINT('',(3.15,4.35,72.5433944458772));
#61339=CARTESIAN_POINT('',(1.64360758375303,4.35,71.995112445239));
#61340=CARTESIAN_POINT('',(3.,4.5,72.6484255766087));
#61341=CARTESIAN_POINT('',(3.15,4.35,72.5433944458772));
#61342=CARTESIAN_POINT('',(1.59230456225418,4.5,72.1360663383568));
#61343=CARTESIAN_POINT('Origin',(4.42952305344106,-2.25,71.6061636956896));
#61344=CARTESIAN_POINT('',(4.42952305344105,-4.42047694655895,71.6061636956896));
#61345=CARTESIAN_POINT('',(4.5,-4.35,71.5055121849402));
#61346=CARTESIAN_POINT('',(6.84407698594489,-2.00592301405511,68.1578233098128));
#61347=CARTESIAN_POINT('',(4.5,4.35,71.5055121849402));
#61348=CARTESIAN_POINT('',(4.5,-2.25,71.5055121849402));
#61349=CARTESIAN_POINT('',(4.42952305344105,4.42047694655895,71.6061636956896));
#61350=CARTESIAN_POINT('',(7.40106189830217,1.44893810169782,67.3623664174442));
#61351=CARTESIAN_POINT('',(4.35904610688211,4.35,71.706815206439));
#61352=CARTESIAN_POINT('',(3.98708884813977,3.97804274125761,72.2380252241052));
#61353=CARTESIAN_POINT('',(4.35904610688211,-4.35,71.706815206439));
#61354=CARTESIAN_POINT('',(4.35904610688211,-2.25,71.706815206439));
#61355=CARTESIAN_POINT('',(3.79658878858514,-3.78754268170298,72.5100875044424));
#61356=CARTESIAN_POINT('Origin',(6.45910097600251,4.425,70.8626444108177));
#61357=CARTESIAN_POINT('',(4.35,4.5,71.5504810542087));
#61358=CARTESIAN_POINT('',(3.02219331113791,5.82780668886209,70.6207408013823));
#61359=CARTESIAN_POINT('',(3.,4.5,72.0418408704681));
#61360=CARTESIAN_POINT('',(6.43344946525308,4.5,70.7921674642588));
#61361=CARTESIAN_POINT('',(3.15,4.35,72.1468720011996));
#61362=CARTESIAN_POINT('',(3.15,4.35,72.1468720011996));
#61363=CARTESIAN_POINT('',(6.48475248675193,4.35,70.9331213573767));
#61364=CARTESIAN_POINT('Origin',(4.425,4.425,59.4601776313845));
#61365=CARTESIAN_POINT('',(4.5,4.35,71.2997986699827));
#61366=CARTESIAN_POINT('',(4.5,4.35,59.4601776313845));
#61367=CARTESIAN_POINT('',(4.42952305344104,4.42047694655896,71.1991471592332));
#61368=CARTESIAN_POINT('',(3.17896133170339,5.67103866829661,69.4131599290257));
#61369=CARTESIAN_POINT('',(4.35,4.5,71.2548298007141));
#61370=CARTESIAN_POINT('',(5.70115354651634,3.14884645348366,70.3087419021648));
#61371=CARTESIAN_POINT('',(4.35,4.5,59.4601776313845));
#61372=CARTESIAN_POINT('Origin',(4.5,-4.5,59.4601776313845));
#61373=CARTESIAN_POINT('',(4.5,-4.35,71.2997986699827));
#61374=CARTESIAN_POINT('',(4.5,-4.35,59.4601776313845));
#61375=CARTESIAN_POINT('',(4.5,-2.25,71.2997986699827));
#61376=CARTESIAN_POINT('Origin',(4.42952305344105,-2.25,71.1991471592333));
#61377=CARTESIAN_POINT('',(4.42952305344104,-4.42047694655895,71.1991471592332));
#61378=CARTESIAN_POINT('',(2.62197641934605,-6.22802358065395,68.6177030366572));
#61379=CARTESIAN_POINT('',(4.35904610688211,-4.35,71.0984956484838));
#61380=CARTESIAN_POINT('',(2.94288811686221,-2.93384200998003,69.0760124378051));
#61381=CARTESIAN_POINT('',(4.35904610688211,4.35,71.0984956484838));
#61382=CARTESIAN_POINT('',(4.35904610688211,-2.25,71.0984956484838));
#61383=CARTESIAN_POINT('',(3.13338817641685,3.12434206953468,69.3480747181423));
#61384=CARTESIAN_POINT('Origin',(1.92086259786507,4.425,70.2908827584586));
#61385=CARTESIAN_POINT('',(3.15,4.35,70.6584388537233));
#61386=CARTESIAN_POINT('',(1.94651410861449,4.35,70.2204058118997));
#61387=CARTESIAN_POINT('',(3.,4.5,70.7634699844547));
#61388=CARTESIAN_POINT('',(3.15,4.35,70.6584388537233));
#61389=CARTESIAN_POINT('',(1.89521108711565,4.5,70.3613597050175));
#61390=CARTESIAN_POINT('Origin',(4.42952305344106,-2.25,69.7212081035357));
#61391=CARTESIAN_POINT('',(4.42952305344105,-4.42047694655895,69.7212081035357));
#61392=CARTESIAN_POINT('',(4.5,-4.35,69.6205565927863));
#61393=CARTESIAN_POINT('',(6.51087678203658,-2.33912321796342,66.7487269247166));
#61394=CARTESIAN_POINT('',(4.5,4.35,69.6205565927863));
#61395=CARTESIAN_POINT('',(4.5,-2.25,69.6205565927863));
#61396=CARTESIAN_POINT('',(4.42952305344105,4.42047694655895,69.7212081035357));
#61397=CARTESIAN_POINT('',(7.06786169439386,1.78213830560614,65.9532700323481));
#61398=CARTESIAN_POINT('',(4.35904610688211,4.35,69.8218596142852));
#61399=CARTESIAN_POINT('',(3.93010825739134,3.92106215050918,70.4344463490517));
#61400=CARTESIAN_POINT('',(4.35904610688211,-4.35,69.8218596142852));
#61401=CARTESIAN_POINT('',(4.35904610688211,-2.25,69.8218596142852));
#61402=CARTESIAN_POINT('',(3.73960819783673,-3.73056209095443,70.7065086293889));
#61403=CARTESIAN_POINT('Origin',(2.18259445412334,-4.425,70.5342098992732));
#61404=CARTESIAN_POINT('',(3.15,-4.35,70.2619164090457));
#61405=CARTESIAN_POINT('',(2.20824596487276,-4.35,70.6046868458321));
#61406=CARTESIAN_POINT('',(3.,-4.5,70.1568852783142));
#61407=CARTESIAN_POINT('',(3.,-4.5,70.1568852783142));
#61408=CARTESIAN_POINT('',(4.35,-4.5,69.6655254620549));
#61409=CARTESIAN_POINT('',(2.15694294337392,-4.5,70.4637329527142));
#61410=CARTESIAN_POINT('',(2.64738592608591,-6.20261407391409,68.4733422528387));
#61411=CARTESIAN_POINT('Origin',(4.55,0.,69.752358081073));
#61412=CARTESIAN_POINT('',(3.15,4.35,70.2619164090457));
#61413=CARTESIAN_POINT('',(6.18184596189047,4.35,69.1584147240374));
#61414=CARTESIAN_POINT('',(3.15,0.,70.2619164090457));
#61415=CARTESIAN_POINT('Origin',(6.15619445114104,4.425,69.0879377774784));
#61416=CARTESIAN_POINT('',(4.35,4.5,69.6655254620549));
#61417=CARTESIAN_POINT('',(3.24187665723131,5.60812334276869,68.8896091441821));
#61418=CARTESIAN_POINT('',(3.,4.5,70.1568852783142));
#61419=CARTESIAN_POINT('',(6.13054294039162,4.5,69.0174608309195));
#61420=CARTESIAN_POINT('',(3.15,4.35,70.2619164090457));
#61421=CARTESIAN_POINT('Origin',(4.42952305344106,-2.25,116.845097907383));
#61422=CARTESIAN_POINT('',(4.42952305344105,-4.42047694655895,116.845097907383));
#61423=CARTESIAN_POINT('',(4.5,-4.35,116.744446396633));
#61424=CARTESIAN_POINT('',(14.8408818797443,5.9908818797443,101.97613655212));
#61425=CARTESIAN_POINT('',(4.5,4.35,116.744446396633));
#61426=CARTESIAN_POINT('',(4.5,-2.25,116.744446396633));
#61427=CARTESIAN_POINT('',(4.42952305344106,4.42047694655894,116.845097907383));
#61428=CARTESIAN_POINT('',(15.3978667921016,-6.54786679210158,101.180679659752));
#61429=CARTESIAN_POINT('',(4.35904610688211,4.35,116.945749418132));
#61430=CARTESIAN_POINT('',(5.35462302610208,5.34557691922005,115.52391822539));
#61431=CARTESIAN_POINT('',(4.35904610688212,-4.35,116.945749418132));
#61432=CARTESIAN_POINT('',(4.35904610688211,-2.25,116.945749418132));
#61433=CARTESIAN_POINT('',(5.16412296654744,-5.15507685966539,115.795980505727));
#61434=CARTESIAN_POINT('Origin',(13.7288575726779,4.425,113.45560361096));
#61435=CARTESIAN_POINT('',(4.35,4.5,116.789415265902));
#61436=CARTESIAN_POINT('',(-2.25020699510341,11.1002069951034,112.167900574186));
#61437=CARTESIAN_POINT('',(3.,4.5,117.280775082161));
#61438=CARTESIAN_POINT('',(13.7032060619285,4.5,113.385126664401));
#61439=CARTESIAN_POINT('',(3.15,4.35,117.385806212893));
#61440=CARTESIAN_POINT('',(3.15,4.35,117.385806212893));
#61441=CARTESIAN_POINT('',(13.7545090834273,4.35,113.526080557519));
#61442=CARTESIAN_POINT('Origin',(4.425,4.425,59.4601776313845));
#61443=CARTESIAN_POINT('',(4.5,4.35,116.538732881676));
#61444=CARTESIAN_POINT('',(4.5,4.35,59.4601776313845));
#61445=CARTESIAN_POINT('',(4.42952305344106,4.42047694655894,116.438081370926));
#61446=CARTESIAN_POINT('',(-4.8178435620961,13.6678435620961,103.231473171333));
#61447=CARTESIAN_POINT('',(4.35,4.5,116.493764012407));
#61448=CARTESIAN_POINT('',(10.9735538527579,-2.12355385275793,111.855901674968));
#61449=CARTESIAN_POINT('',(4.35,4.5,59.4601776313845));
#61450=CARTESIAN_POINT('Origin',(4.5,-4.5,59.4601776313845));
#61451=CARTESIAN_POINT('',(4.5,-4.35,116.538732881676));
#61452=CARTESIAN_POINT('',(4.5,-4.35,59.4601776313845));
#61453=CARTESIAN_POINT('',(4.5,-2.25,116.538732881676));
#61454=CARTESIAN_POINT('Origin',(4.42952305344106,-2.25,116.438081370926));
#61455=CARTESIAN_POINT('',(4.42952305344106,-4.42047694655894,116.438081370926));
#61456=CARTESIAN_POINT('',(-5.37482847445338,-14.2248284744534,102.436016278964));
#61457=CARTESIAN_POINT('',(4.35904610688211,-4.35,116.337429860177));
#61458=CARTESIAN_POINT('',(1.57535393889992,-1.56630783201787,112.361905439089));
#61459=CARTESIAN_POINT('',(4.35904610688211,4.35,116.337429860177));
#61460=CARTESIAN_POINT('',(4.35904610688211,-2.25,116.337429860177));
#61461=CARTESIAN_POINT('',(1.76585399845467,1.75680789157236,112.633967719427));
#61462=CARTESIAN_POINT('Origin',(-5.34889399881033,4.425,112.883841958601));
#61463=CARTESIAN_POINT('',(3.15,4.35,115.897373065416));
#61464=CARTESIAN_POINT('',(-5.3232424880609,4.35,112.813365012042));
#61465=CARTESIAN_POINT('',(3.,4.5,116.002404196148));
#61466=CARTESIAN_POINT('',(3.15,4.35,115.897373065416));
#61467=CARTESIAN_POINT('',(-5.37454550955975,4.5,112.95431890516));
#61468=CARTESIAN_POINT('Origin',(4.42952305344106,-2.25,114.960142315229));
#61469=CARTESIAN_POINT('',(4.42952305344107,-4.42047694655893,114.960142315229));
#61470=CARTESIAN_POINT('',(4.5,-4.35,114.859490804479));
#61471=CARTESIAN_POINT('',(14.507681675836,5.65768167583598,100.567040167024));
#61472=CARTESIAN_POINT('',(4.5,4.35,114.859490804479));
#61473=CARTESIAN_POINT('',(4.5,-2.25,114.859490804479));
#61474=CARTESIAN_POINT('',(4.42952305344106,4.42047694655894,114.960142315229));
#61475=CARTESIAN_POINT('',(15.0646665881933,-6.21466658819326,99.7715832746552));
#61476=CARTESIAN_POINT('',(4.35904610688211,4.35,115.060793825978));
#61477=CARTESIAN_POINT('',(5.29764243535362,5.28859632847161,113.720339350336));
#61478=CARTESIAN_POINT('',(4.35904610688212,-4.35,115.060793825978));
#61479=CARTESIAN_POINT('',(4.35904610688212,-2.25,115.060793825978));
#61480=CARTESIAN_POINT('',(5.10714237579906,-5.09809626891695,113.992401630673));
#61481=CARTESIAN_POINT('Origin',(13.4259510478164,4.425,111.680896977621));
#61482=CARTESIAN_POINT('',(4.35,4.5,114.904459673748));
#61483=CARTESIAN_POINT('',(-2.03052364901003,10.88052364901,110.436768916986));
#61484=CARTESIAN_POINT('',(3.,4.5,115.395819490007));
#61485=CARTESIAN_POINT('',(13.400299537067,4.5,111.610420031062));
#61486=CARTESIAN_POINT('',(3.15,4.35,115.500850620739));
#61487=CARTESIAN_POINT('',(3.15,4.35,115.500850620739));
#61488=CARTESIAN_POINT('',(13.4516025585659,4.35,111.75137392418));
#61489=CARTESIAN_POINT('Origin',(4.425,4.425,59.4601776313845));
#61490=CARTESIAN_POINT('',(4.5,4.35,114.653777289522));
#61491=CARTESIAN_POINT('',(4.5,4.35,59.4601776313845));
#61492=CARTESIAN_POINT('',(4.42952305344105,4.42047694655895,114.553125778772));
#61493=CARTESIAN_POINT('',(-4.48464335818771,13.3346433581877,101.822376786238));
#61494=CARTESIAN_POINT('',(4.35,4.5,114.608808420253));
#61495=CARTESIAN_POINT('',(10.7538705066645,-1.90387050666449,110.124770017768));
#61496=CARTESIAN_POINT('',(4.35,4.5,59.4601776313845));
#61497=CARTESIAN_POINT('Origin',(4.5,-4.5,59.4601776313845));
#61498=CARTESIAN_POINT('',(4.5,-4.35,114.653777289522));
#61499=CARTESIAN_POINT('',(4.5,-4.35,59.4601776313845));
#61500=CARTESIAN_POINT('',(4.5,-2.25,114.653777289522));
#61501=CARTESIAN_POINT('Origin',(4.42952305344105,-2.25,114.553125778772));
#61502=CARTESIAN_POINT('',(4.42952305344105,-4.42047694655895,114.553125778772));
#61503=CARTESIAN_POINT('',(-5.04162827054505,-13.8916282705451,101.02691989387));
#61504=CARTESIAN_POINT('',(4.35904610688211,-4.35,114.452474268023));
#61505=CARTESIAN_POINT('',(1.63233452964815,-1.62328842276621,110.558326564036));
#61506=CARTESIAN_POINT('',(4.35904610688211,4.35,114.452474268023));
#61507=CARTESIAN_POINT('',(4.35904610688211,-2.25,114.452474268023));
#61508=CARTESIAN_POINT('',(1.82283458920287,1.81378848232088,110.830388844373));
#61509=CARTESIAN_POINT('Origin',(-5.04598747394865,4.425,111.109135325262));
#61510=CARTESIAN_POINT('',(3.15,4.35,114.012417473262));
#61511=CARTESIAN_POINT('',(-5.02033596319923,4.35,111.038658378703));
#61512=CARTESIAN_POINT('',(3.,4.5,114.117448603994));
#61513=CARTESIAN_POINT('',(3.15,4.35,114.012417473262));
#61514=CARTESIAN_POINT('',(-5.07163898469808,4.5,111.179612271821));
#61515=CARTESIAN_POINT('Origin',(4.42952305344106,-2.25,113.075186723075));
#61516=CARTESIAN_POINT('',(4.5,4.35,112.974535212325));
#61517=CARTESIAN_POINT('',(4.5,-2.25,112.974535212325));
#61518=CARTESIAN_POINT('',(4.42952305344106,4.42047694655894,113.075186723075));
#61519=CARTESIAN_POINT('',(14.731466384285,-5.88146638428496,98.3624868895593));
#61520=CARTESIAN_POINT('',(4.35904610688211,4.35,113.175838233824));
#61521=CARTESIAN_POINT('',(5.24066184460522,5.23161573772318,111.916760475283));
#61522=CARTESIAN_POINT('',(4.35904610688212,-4.35,113.175838233824));
#61523=CARTESIAN_POINT('',(4.35904610688211,-2.25,113.175838233824));
#61524=CARTESIAN_POINT('',(5.05016178505058,-5.04111567816854,112.18882275562));
#61525=CARTESIAN_POINT('Origin',(9.14944452593728,-4.425,111.352462466077));
#61526=CARTESIAN_POINT('',(3.15,-4.35,113.615895028585));
#61527=CARTESIAN_POINT('',(9.17509603668671,-4.35,111.422939412636));
#61528=CARTESIAN_POINT('',(3.,-4.5,113.510863897853));
#61529=CARTESIAN_POINT('',(3.,-4.5,113.510863897853));
#61530=CARTESIAN_POINT('',(9.12379301518786,-4.5,111.281985519518));
#61531=CARTESIAN_POINT('Origin',(4.55,0.,113.106336700612));
#61532=CARTESIAN_POINT('',(3.15,4.35,113.615895028585));
#61533=CARTESIAN_POINT('',(13.1486960337044,4.35,109.976667290841));
#61534=CARTESIAN_POINT('',(3.15,0.,113.615895028585));
#61535=CARTESIAN_POINT('Origin',(13.123044522955,4.425,109.906190344282));
#61536=CARTESIAN_POINT('',(4.35,4.5,113.019504081594));
#61537=CARTESIAN_POINT('',(-1.81084030291663,10.6608403029166,108.705637259786));
#61538=CARTESIAN_POINT('',(3.,4.5,113.510863897853));
#61539=CARTESIAN_POINT('',(13.0973930122055,4.5,109.835713397723));
#61540=CARTESIAN_POINT('',(3.15,4.35,113.615895028585));
#61541=CARTESIAN_POINT('Origin',(4.178033008589,-1.125,59.5132106399735));
#61542=CARTESIAN_POINT('',(4.05000000000001,4.2,59.4601776313845));
#61543=CARTESIAN_POINT('',(4.30606601717799,4.30606601717799,59.5662436485625));
#61544=CARTESIAN_POINT('',(2.66093885398715,3.62463203435592,58.8848096657404));
#61545=CARTESIAN_POINT('',(4.30606601717799,-4.30606601717799,59.5662436485625));
#61546=CARTESIAN_POINT('',(4.30606601717798,-1.125,59.5662436485625));
#61547=CARTESIAN_POINT('',(4.05000000000001,-4.2,59.4601776313845));
#61548=CARTESIAN_POINT('',(1.33270642526082,-3.07446014839369,58.3346377797782));
#61549=CARTESIAN_POINT('',(4.05000000000001,-1.125,59.4601776313845));
#61550=CARTESIAN_POINT('Origin',(0.,0.,59.4601776313845));
#61551=CARTESIAN_POINT('',(-4.05000000000001,-4.2,59.4601776313845));
#61552=CARTESIAN_POINT('',(-2.25,-4.2,59.4601776313845));
#61553=CARTESIAN_POINT('',(-4.05000000000001,4.2,59.4601776313845));
#61554=CARTESIAN_POINT('',(-4.05000000000001,1.125,59.4601776313845));
#61555=CARTESIAN_POINT('',(2.25,4.2,59.4601776313845));
#61556=CARTESIAN_POINT('',(-1.905,2.33295215237571E-16,59.4601776313845));
#61557=CARTESIAN_POINT('Origin',(0.,0.,59.4601776313845));
#61558=CARTESIAN_POINT('Origin',(-2.25,-4.35,59.6101776313845));
#61559=CARTESIAN_POINT('',(4.39393398282202,-4.39393398282202,59.6541116142065));
#61560=CARTESIAN_POINT('',(4.2,-4.2,59.4601776313845));
#61561=CARTESIAN_POINT('',(-4.39393398282202,-4.39393398282202,59.6541116142065));
#61562=CARTESIAN_POINT('',(-3.375,-4.39393398282202,59.6541116142065));
#61563=CARTESIAN_POINT('',(-4.30606601717799,-4.30606601717799,59.5662436485625));
#61564=CARTESIAN_POINT('',(-4.2,-4.2,59.4601776313845));
#61565=CARTESIAN_POINT('',(-2.66093885398715,-3.62463203435592,58.8848096657404));
#61566=CARTESIAN_POINT('Origin',(-4.44696699141101,3.375,59.7821446227955));
#61567=CARTESIAN_POINT('',(-4.425,4.425,59.7291116142065));
#61568=CARTESIAN_POINT('',(-4.39393398282202,4.39393398282202,59.6541116142065));
#61569=CARTESIAN_POINT('',(-3.87891329166411,3.87891329166411,58.4107416767103));
#61570=CARTESIAN_POINT('',(-4.39393398282202,3.375,59.6541116142065));
#61571=CARTESIAN_POINT('',(-4.425,-4.425,59.7291116142065));
#61572=CARTESIAN_POINT('',(-3.87891329166411,-3.87891329166411,58.4107416767103));
#61573=CARTESIAN_POINT('',(-4.5,-4.35,59.9101776313845));
#61574=CARTESIAN_POINT('',(-4.89129647405225,-3.95870352594775,60.8548508859502));
#61575=CARTESIAN_POINT('',(-4.5,4.35,59.9101776313845));
#61576=CARTESIAN_POINT('',(-4.5,3.375,59.9101776313845));
#61577=CARTESIAN_POINT('',(-4.46017538852391,4.38982461147609,59.8140325142427));
#61578=CARTESIAN_POINT('Origin',(-4.35,2.25,59.6101776313845));
#61579=CARTESIAN_POINT('',(-4.30606601717799,4.30606601717799,59.5662436485625));
#61580=CARTESIAN_POINT('',(-4.5,4.5,59.7601776313845));
#61581=CARTESIAN_POINT('',(-4.30606601717798,1.125,59.5662436485625));
#61582=CARTESIAN_POINT('Origin',(3.375,4.44696699141101,59.7821446227955));
#61583=CARTESIAN_POINT('',(-4.35,4.5,59.9101776313845));
#61584=CARTESIAN_POINT('',(-3.95870352594775,4.89129647405225,60.8548508859502));
#61585=CARTESIAN_POINT('',(4.35,4.5,59.9101776313845));
#61586=CARTESIAN_POINT('',(3.375,4.5,59.9101776313845));
#61587=CARTESIAN_POINT('',(4.43786796564403,4.41213203435597,59.6980455970285));
#61588=CARTESIAN_POINT('',(4.38982461147609,4.46017538852391,59.8140325142427));
#61589=CARTESIAN_POINT('',(4.39393398282202,4.39393398282202,59.6541116142065));
#61590=CARTESIAN_POINT('',(3.53998854218627,4.04021819978403,58.8001661735708));
#61591=CARTESIAN_POINT('',(3.375,4.39393398282202,59.6541116142065));
#61592=CARTESIAN_POINT('Origin',(-4.425,4.425,59.4601776313845));
#61593=CARTESIAN_POINT('',(-4.5,4.35,144.510177631384));
#61594=CARTESIAN_POINT('',(-4.5,4.35,59.4601776313845));
#61595=CARTESIAN_POINT('',(-4.425,4.425,144.691243648562));
#61596=CARTESIAN_POINT('',(-17.6438747634856,-8.7938747634856,112.778056915244));
#61597=CARTESIAN_POINT('',(-4.35,4.5,144.510177631384));
#61598=CARTESIAN_POINT('',(9.22499584901393,18.0749958490139,111.737238543536));
#61599=CARTESIAN_POINT('',(-4.35,4.5,59.4601776313845));
#61600=CARTESIAN_POINT('Origin',(-4.178033008589,1.125,59.5132106399735));
#61601=CARTESIAN_POINT('',(-1.33270642526082,3.07446014839369,58.3346377797782));
#61602=CARTESIAN_POINT('Origin',(4.44696699141101,-3.375,144.638210639973));
#61603=CARTESIAN_POINT('',(4.425,4.425,144.691243648562));
#61604=CARTESIAN_POINT('',(4.39393398282201,4.39393398282201,144.766243648562));
#61605=CARTESIAN_POINT('',(3.87891329166412,3.87891329166412,146.009613586059));
#61606=CARTESIAN_POINT('',(4.39393398282201,-4.39393398282201,144.766243648562));
#61607=CARTESIAN_POINT('',(4.39393398282201,-3.375,144.766243648562));
#61608=CARTESIAN_POINT('',(4.425,-4.425,144.691243648562));
#61609=CARTESIAN_POINT('',(3.87891329166412,-3.87891329166411,146.009613586059));
#61610=CARTESIAN_POINT('',(4.5,-4.35,144.510177631384));
#61611=CARTESIAN_POINT('',(17.6438747634856,8.7938747634856,112.778056915244));
#61612=CARTESIAN_POINT('',(4.5,4.35,144.510177631384));
#61613=CARTESIAN_POINT('',(4.5,-3.375,144.510177631384));
#61614=CARTESIAN_POINT('',(18.0749958490139,-9.22499584901393,111.737238543536));
#61615=CARTESIAN_POINT('Origin',(3.375,4.44696699141101,144.638210639973));
#61616=CARTESIAN_POINT('',(4.35,4.5,144.510177631384));
#61617=CARTESIAN_POINT('',(-8.7938747634856,17.6438747634856,112.778056915244));
#61618=CARTESIAN_POINT('',(3.375,4.5,144.510177631384));
#61619=CARTESIAN_POINT('',(-4.39393398282201,4.39393398282201,144.766243648562));
#61620=CARTESIAN_POINT('',(-3.87891329166412,3.87891329166411,146.009613586059));
#61621=CARTESIAN_POINT('',(3.375,4.39393398282201,144.766243648562));
#61622=CARTESIAN_POINT('Origin',(4.425,4.425,59.4601776313845));
#61623=CARTESIAN_POINT('',(4.5,4.35,129.733422026753));
#61624=CARTESIAN_POINT('',(4.5,4.35,59.4601776313845));
#61625=CARTESIAN_POINT('',(4.42952305344106,4.42047694655894,129.632770516003));
#61626=CARTESIAN_POINT('',(-7.15024498945427,16.0002449894543,113.095147867005));
#61627=CARTESIAN_POINT('',(4.35,4.5,129.688453157484));
#61628=CARTESIAN_POINT('',(12.5113372754116,-3.66133727541164,123.973823275369));
#61629=CARTESIAN_POINT('',(4.35,4.5,59.4601776313845));
#61630=CARTESIAN_POINT('Origin',(4.5,-4.5,59.4601776313845));
#61631=CARTESIAN_POINT('',(4.5,-4.35,129.733422026753));
#61632=CARTESIAN_POINT('',(4.5,-4.35,59.4601776313845));
#61633=CARTESIAN_POINT('',(4.5,-2.25,129.733422026753));
#61634=CARTESIAN_POINT('Origin',(4.42952305344106,-2.25,126.269875868152));
#61635=CARTESIAN_POINT('',(4.42952305344105,-4.42047694655895,126.269875868152));
#61636=CARTESIAN_POINT('',(4.5,-4.35,126.169224357403));
#61637=CARTESIAN_POINT('',(16.5068828992858,7.65688289928583,109.0216184776));
#61638=CARTESIAN_POINT('',(4.5,4.35,126.169224357403));
#61639=CARTESIAN_POINT('',(4.5,-2.25,126.169224357403));
#61640=CARTESIAN_POINT('',(4.42952305344107,4.42047694655893,126.269875868152));
#61641=CARTESIAN_POINT('',(17.0638678116431,-8.21386781164311,108.226161585232));
#61642=CARTESIAN_POINT('',(4.35904610688212,4.35,126.370527378901));
#61643=CARTESIAN_POINT('',(5.63952597984432,5.63047987296221,124.541812600657));
#61644=CARTESIAN_POINT('',(4.35904610688212,-4.35,126.370527378901));
#61645=CARTESIAN_POINT('',(4.35904610688212,-2.25,126.370527378901));
#61646=CARTESIAN_POINT('',(5.44902592028955,-5.43997981340756,124.813874880994));
#61647=CARTESIAN_POINT('Origin',(15.2433901969853,4.425,122.329136777657));
#61648=CARTESIAN_POINT('',(4.35,4.5,126.214193226671));
#61649=CARTESIAN_POINT('',(-3.34862372557137,12.1986237255714,120.823558860185));
#61650=CARTESIAN_POINT('',(3.,4.5,126.705553042931));
#61651=CARTESIAN_POINT('',(15.2177386862358,4.5,122.258659831098));
#61652=CARTESIAN_POINT('',(3.15,4.35,126.810584173662));
#61653=CARTESIAN_POINT('',(3.15,4.35,126.810584173662));
#61654=CARTESIAN_POINT('',(15.2690417077347,4.35,122.399613724216));
#61655=CARTESIAN_POINT('Origin',(4.425,4.425,59.4601776313845));
#61656=CARTESIAN_POINT('',(4.5,4.35,125.963510842445));
#61657=CARTESIAN_POINT('',(4.5,4.35,59.4601776313845));
#61658=CARTESIAN_POINT('',(4.42952305344105,4.42047694655895,125.862859331696));
#61659=CARTESIAN_POINT('',(-6.48384458163758,15.3338445816376,110.276955096815));
#61660=CARTESIAN_POINT('',(4.35,4.5,125.918541973177));
#61661=CARTESIAN_POINT('',(12.0719705832239,-3.22197058322388,120.511559960971));
#61662=CARTESIAN_POINT('',(4.35,4.5,59.4601776313845));
#61663=CARTESIAN_POINT('Origin',(4.5,-4.5,59.4601776313845));
#61664=CARTESIAN_POINT('',(4.5,-4.35,125.963510842445));
#61665=CARTESIAN_POINT('',(4.5,-4.35,59.4601776313845));
#61666=CARTESIAN_POINT('',(4.5,-2.25,125.963510842445));
#61667=CARTESIAN_POINT('Origin',(4.42952305344106,-2.25,125.862859331696));
#61668=CARTESIAN_POINT('',(4.42952305344105,-4.42047694655895,125.862859331696));
#61669=CARTESIAN_POINT('',(-7.04082949399491,-15.8908294939949,109.481498204446));
#61670=CARTESIAN_POINT('',(4.35904610688211,-4.35,125.762207820946));
#61671=CARTESIAN_POINT('',(1.29045098515763,-1.28140487827559,121.379799814357));
#61672=CARTESIAN_POINT('',(4.35904610688211,4.35,125.762207820946));
#61673=CARTESIAN_POINT('',(4.35904610688211,-2.25,125.762207820946));
#61674=CARTESIAN_POINT('',(1.48095104471238,1.47190493783007,121.651862094694));
#61675=CARTESIAN_POINT('Origin',(-6.86342662311746,4.425,121.757375125298));
#61676=CARTESIAN_POINT('',(3.15,4.35,125.322151026186));
#61677=CARTESIAN_POINT('',(-6.83777511236803,4.35,121.686898178739));
#61678=CARTESIAN_POINT('',(3.,4.5,125.427182156917));
#61679=CARTESIAN_POINT('',(3.15,4.35,125.322151026186));
#61680=CARTESIAN_POINT('',(-6.88907813386688,4.5,121.827852071857));
#61681=CARTESIAN_POINT('Origin',(4.42952305344106,-2.25,124.384920275998));
#61682=CARTESIAN_POINT('',(4.42952305344105,-4.42047694655895,124.384920275998));
#61683=CARTESIAN_POINT('',(4.5,-4.35,124.284268765249));
#61684=CARTESIAN_POINT('',(16.1736826953775,7.32368269537753,107.612522092505));
#61685=CARTESIAN_POINT('',(4.5,4.35,124.284268765249));
#61686=CARTESIAN_POINT('',(4.5,-2.25,124.284268765249));
#61687=CARTESIAN_POINT('',(4.42952305344105,4.42047694655895,124.384920275998));
#61688=CARTESIAN_POINT('',(16.7306676077348,-7.88066760773481,106.817065200136));
#61689=CARTESIAN_POINT('',(4.35904610688212,4.35,124.485571786748));
#61690=CARTESIAN_POINT('',(5.58254538909579,5.57349928221377,122.738233725604));
#61691=CARTESIAN_POINT('',(4.35904610688211,-4.35,124.485571786748));
#61692=CARTESIAN_POINT('',(4.35904610688211,-2.25,124.485571786748));
#61693=CARTESIAN_POINT('',(5.39204532954109,-5.38299922265914,123.010296005941));
#61694=CARTESIAN_POINT('Origin',(14.9404836721238,4.425,120.554430144318));
#61695=CARTESIAN_POINT('',(4.35,4.5,124.329237634517));
#61696=CARTESIAN_POINT('',(-3.12894037947692,11.9789403794769,119.092427202987));
#61697=CARTESIAN_POINT('',(3.,4.5,124.820597450777));
#61698=CARTESIAN_POINT('',(14.9148321613744,4.5,120.483953197759));
#61699=CARTESIAN_POINT('',(3.15,4.35,124.925628581508));
#61700=CARTESIAN_POINT('',(3.15,4.35,124.925628581508));
#61701=CARTESIAN_POINT('',(14.9661351828732,4.35,120.624907090876));
#61702=CARTESIAN_POINT('Origin',(4.425,4.425,59.4601776313845));
#61703=CARTESIAN_POINT('',(4.5,4.35,124.078555250291));
#61704=CARTESIAN_POINT('',(4.5,4.35,59.4601776313845));
#61705=CARTESIAN_POINT('',(4.42952305344105,4.42047694655896,123.977903739542));
#61706=CARTESIAN_POINT('',(-6.15064437772934,15.0006443777293,108.867858711717));
#61707=CARTESIAN_POINT('',(4.35,4.5,124.033586381023));
#61708=CARTESIAN_POINT('',(11.8522872371324,-3.00228723713242,118.780428303768));
#61709=CARTESIAN_POINT('',(4.35,4.5,59.4601776313845));
#61710=CARTESIAN_POINT('Origin',(4.5,-4.5,59.4601776313845));
#61711=CARTESIAN_POINT('',(4.5,-4.35,124.078555250291));
#61712=CARTESIAN_POINT('',(4.5,-4.35,59.4601776313845));
#61713=CARTESIAN_POINT('',(4.5,-2.25,124.078555250291));
#61714=CARTESIAN_POINT('Origin',(4.42952305344106,-2.25,123.977903739542));
#61715=CARTESIAN_POINT('',(4.42952305344106,-4.42047694655894,123.977903739542));
#61716=CARTESIAN_POINT('',(-6.70762929008662,-15.5576292900866,108.072401819349));
#61717=CARTESIAN_POINT('',(4.35904610688212,-4.35,123.877252228792));
#61718=CARTESIAN_POINT('',(1.34743157590636,-1.33838546902397,119.576220939304));
#61719=CARTESIAN_POINT('',(4.35904610688212,4.35,123.877252228792));
#61720=CARTESIAN_POINT('',(4.35904610688212,-2.25,123.877252228792));
#61721=CARTESIAN_POINT('',(1.53793163546093,1.52888552857883,119.848283219641));
#61722=CARTESIAN_POINT('Origin',(-6.56052009825622,4.425,119.982668491958));
#61723=CARTESIAN_POINT('',(3.15,4.35,123.437195434032));
#61724=CARTESIAN_POINT('',(-6.53486858750679,4.35,119.912191545399));
#61725=CARTESIAN_POINT('',(3.,4.5,123.542226564763));
#61726=CARTESIAN_POINT('',(3.15,4.35,123.437195434032));
#61727=CARTESIAN_POINT('',(-6.58617160900565,4.5,120.053145438517));
#61728=CARTESIAN_POINT('Origin',(4.42952305344106,-2.25,122.499964683844));
#61729=CARTESIAN_POINT('',(4.42952305344106,-4.42047694655893,122.499964683844));
#61730=CARTESIAN_POINT('',(4.5,-4.35,122.399313173095));
#61731=CARTESIAN_POINT('',(15.8404824914692,6.99048249146922,106.203425707408));
#61732=CARTESIAN_POINT('',(4.5,4.35,122.399313173095));
#61733=CARTESIAN_POINT('',(4.5,-2.25,122.399313173095));
#61734=CARTESIAN_POINT('',(4.42952305344106,4.42047694655894,122.499964683844));
#61735=CARTESIAN_POINT('',(16.3974674038265,-7.54746740382649,105.40796881504));
#61736=CARTESIAN_POINT('',(4.35904610688212,4.35,122.600616194594));
#61737=CARTESIAN_POINT('',(5.52556479834734,5.51651869146533,120.93465485055));
#61738=CARTESIAN_POINT('',(4.35904610688211,-4.35,122.600616194594));
#61739=CARTESIAN_POINT('',(4.35904610688212,-2.25,122.600616194594));
#61740=CARTESIAN_POINT('',(5.33506473879272,-5.32601863191069,121.206717130887));
#61741=CARTESIAN_POINT('Origin',(14.6375771472623,4.425,118.779723510978));
#61742=CARTESIAN_POINT('',(4.35,4.5,122.444282042363));
#61743=CARTESIAN_POINT('',(-2.90925703338358,11.7592570333836,117.361295545787));
#61744=CARTESIAN_POINT('',(3.,4.5,122.935641858623));
#61745=CARTESIAN_POINT('',(14.6119256365129,4.5,118.709246564419));
#61746=CARTESIAN_POINT('',(3.15,4.35,123.040672989354));
#61747=CARTESIAN_POINT('',(3.15,4.35,123.040672989354));
#61748=CARTESIAN_POINT('',(14.6632286580117,4.35,118.850200457537));
#61749=CARTESIAN_POINT('Origin',(4.425,4.425,59.4601776313845));
#61750=CARTESIAN_POINT('',(4.5,4.35,122.193599658137));
#61751=CARTESIAN_POINT('',(4.5,4.35,59.4601776313845));
#61752=CARTESIAN_POINT('',(4.42952305344106,4.42047694655895,122.092948147388));
#61753=CARTESIAN_POINT('',(-5.81744417382102,14.667444173821,107.458762326621));
#61754=CARTESIAN_POINT('',(4.35,4.5,122.148630788869));
#61755=CARTESIAN_POINT('',(11.6326038910391,-2.78260389103911,117.049296646567));
#61756=CARTESIAN_POINT('',(4.35,4.5,59.4601776313845));
#61757=CARTESIAN_POINT('Origin',(4.5,-4.5,59.4601776313845));
#61758=CARTESIAN_POINT('',(4.5,-4.35,122.193599658137));
#61759=CARTESIAN_POINT('',(4.5,-4.35,59.4601776313845));
#61760=CARTESIAN_POINT('',(4.5,-2.25,122.193599658137));
#61761=CARTESIAN_POINT('Origin',(4.42952305344106,-2.25,122.092948147388));
#61762=CARTESIAN_POINT('',(4.42952305344105,-4.42047694655894,122.092948147388));
#61763=CARTESIAN_POINT('',(-6.37442908617831,-15.2244290861783,106.663305434253));
#61764=CARTESIAN_POINT('',(4.35904610688211,-4.35,121.992296636638));
#61765=CARTESIAN_POINT('',(1.40441216665457,-1.39536605977259,117.77264206425));
#61766=CARTESIAN_POINT('',(4.35904610688211,4.35,121.992296636638));
#61767=CARTESIAN_POINT('',(4.35904610688211,-2.25,121.992296636638));
#61768=CARTESIAN_POINT('',(1.59491222620929,1.58586611932729,118.044704344587));
#61769=CARTESIAN_POINT('Origin',(-6.25761357339475,4.425,118.207961858619));
#61770=CARTESIAN_POINT('',(3.15,4.35,121.552239841878));
#61771=CARTESIAN_POINT('',(-6.23196206264532,4.35,118.13748491206));
#61772=CARTESIAN_POINT('',(3.,4.5,121.657270972609));
#61773=CARTESIAN_POINT('',(3.15,4.35,121.552239841878));
#61774=CARTESIAN_POINT('',(-6.28326508414417,4.5,118.278438805178));
#61775=CARTESIAN_POINT('Origin',(4.42952305344106,-2.25,120.61500909169));
#61776=CARTESIAN_POINT('',(4.42952305344107,-4.42047694655894,120.61500909169));
#61777=CARTESIAN_POINT('',(4.5,-4.35,120.514357580941));
#61778=CARTESIAN_POINT('',(15.5072822875609,6.65728228756088,104.794329322311));
#61779=CARTESIAN_POINT('',(4.5,4.35,120.514357580941));
#61780=CARTESIAN_POINT('',(4.5,-2.25,120.514357580941));
#61781=CARTESIAN_POINT('',(4.42952305344106,4.42047694655894,120.61500909169));
#61782=CARTESIAN_POINT('',(16.0642671999181,-7.2142671999181,103.998872429942));
#61783=CARTESIAN_POINT('',(4.35904610688212,4.35,120.71566060244));
#61784=CARTESIAN_POINT('',(5.46858420759883,5.45953810071684,119.131075975497));
#61785=CARTESIAN_POINT('',(4.35904610688212,-4.35,120.71566060244));
#61786=CARTESIAN_POINT('',(4.35904610688212,-2.25,120.71566060244));
#61787=CARTESIAN_POINT('',(5.27808414804422,-5.26903804116222,119.403138255834));
#61788=CARTESIAN_POINT('Origin',(14.3346706224008,4.425,117.005016877639));
#61789=CARTESIAN_POINT('',(4.35,4.5,120.55932645021));
#61790=CARTESIAN_POINT('',(-2.68957368729112,11.5395736872911,115.630163888585));
#61791=CARTESIAN_POINT('',(3.,4.5,121.050686266469));
#61792=CARTESIAN_POINT('',(14.3090191116514,4.5,116.93453993108));
#61793=CARTESIAN_POINT('',(3.15,4.35,121.1557173972));
#61794=CARTESIAN_POINT('',(3.15,4.35,121.1557173972));
#61795=CARTESIAN_POINT('',(14.3603221331503,4.35,117.075493824198));
#61796=CARTESIAN_POINT('Origin',(4.425,4.425,59.4601776313845));
#61797=CARTESIAN_POINT('',(4.5,4.35,120.308644065983));
#61798=CARTESIAN_POINT('',(4.5,4.35,59.4601776313845));
#61799=CARTESIAN_POINT('',(4.42952305344105,4.42047694655895,120.207992555234));
#61800=CARTESIAN_POINT('',(-5.48424396991263,14.3342439699126,106.049665941527));
#61801=CARTESIAN_POINT('',(4.35,4.5,120.263675196715));
#61802=CARTESIAN_POINT('',(11.4129205449447,-2.56292054494465,115.318164989369));
#61803=CARTESIAN_POINT('',(4.35,4.5,59.4601776313845));
#61804=CARTESIAN_POINT('Origin',(4.5,-4.5,59.4601776313845));
#61805=CARTESIAN_POINT('',(4.5,-4.35,120.308644065983));
#61806=CARTESIAN_POINT('',(4.5,-4.35,59.4601776313845));
#61807=CARTESIAN_POINT('',(4.5,-2.25,120.308644065983));
#61808=CARTESIAN_POINT('Origin',(4.42952305344105,-2.25,120.207992555234));
#61809=CARTESIAN_POINT('',(4.42952305344106,-4.42047694655894,120.207992555234));
#61810=CARTESIAN_POINT('',(-6.04122888226998,-14.89122888227,105.254209049158));
#61811=CARTESIAN_POINT('',(4.35904610688211,-4.35,120.107341044485));
#61812=CARTESIAN_POINT('',(1.46139275740286,-1.45234665052089,115.969063189196));
#61813=CARTESIAN_POINT('',(4.35904610688211,4.35,120.107341044485));
#61814=CARTESIAN_POINT('',(4.35904610688211,-2.25,120.107341044485));
#61815=CARTESIAN_POINT('',(1.65189281695757,1.64284671007559,116.241125469534));
#61816=CARTESIAN_POINT('Origin',(-5.95470704853306,4.425,116.43325522528));
#61817=CARTESIAN_POINT('',(3.15,4.35,119.667284249724));
#61818=CARTESIAN_POINT('',(-5.92905553778363,4.35,116.362778278721));
#61819=CARTESIAN_POINT('',(3.,4.5,119.772315380456));
#61820=CARTESIAN_POINT('',(3.15,4.35,119.667284249724));
#61821=CARTESIAN_POINT('',(-5.98035855928248,4.5,116.503732171839));
#61822=CARTESIAN_POINT('Origin',(4.42952305344106,-2.25,118.730053499536));
#61823=CARTESIAN_POINT('',(4.42952305344105,-4.42047694655895,118.730053499537));
#61824=CARTESIAN_POINT('',(4.5,-4.35,118.629401988787));
#61825=CARTESIAN_POINT('',(15.1740820836526,6.3240820836526,103.385232937216));
#61826=CARTESIAN_POINT('',(4.5,4.35,118.629401988787));
#61827=CARTESIAN_POINT('',(4.5,-2.25,118.629401988787));
#61828=CARTESIAN_POINT('',(4.42952305344105,4.42047694655895,118.730053499536));
#61829=CARTESIAN_POINT('',(15.7310669960099,-6.88106699600987,102.589776044847));
#61830=CARTESIAN_POINT('',(4.35904610688212,4.35,118.830705010286));
#61831=CARTESIAN_POINT('',(5.41160361685048,5.40255750996847,117.327497100443));
#61832=CARTESIAN_POINT('',(4.35904610688212,-4.35,118.830705010286));
#61833=CARTESIAN_POINT('',(4.35904610688212,-2.25,118.830705010286));
#61834=CARTESIAN_POINT('',(5.22110355729585,-5.21205745041383,117.59955938078));
#61835=CARTESIAN_POINT('Origin',(4.55,0.,118.761203477074));
#61836=CARTESIAN_POINT('',(3.15,4.35,119.270761805046));
#61837=CARTESIAN_POINT('',(14.0574156082888,4.35,115.300787190859));
#61838=CARTESIAN_POINT('',(3.15,-4.35,119.270761805046));
#61839=CARTESIAN_POINT('',(3.15,0.,119.270761805046));
#61840=CARTESIAN_POINT('',(10.0838156112711,-4.35,116.747059312653));
#61841=CARTESIAN_POINT('Origin',(14.0317640975394,4.425,115.2303102443));
#61842=CARTESIAN_POINT('',(4.35,4.5,118.674370858056));
#61843=CARTESIAN_POINT('',(-2.46989034119679,11.3198903411968,113.899032231386));
#61844=CARTESIAN_POINT('',(3.,4.5,119.165730674315));
#61845=CARTESIAN_POINT('',(14.00611258679,4.5,115.159833297741));
#61846=CARTESIAN_POINT('',(3.15,4.35,119.270761805046));
#61847=CARTESIAN_POINT('Origin',(4.425,4.425,59.4601776313845));
#61848=CARTESIAN_POINT('',(4.35,4.5,59.4601776313845));
#61849=CARTESIAN_POINT('',(4.5,4.35,59.4601776313845));
#61850=CARTESIAN_POINT('Origin',(3.075,4.425,86.5380363299847));
#61851=CARTESIAN_POINT('',(3.,4.5,86.5380363299847));
#61852=CARTESIAN_POINT('',(3.15,4.35,86.5380363299847));
#61853=CARTESIAN_POINT('Origin',(3.15,0.,113.615895028585));
#61854=CARTESIAN_POINT('',(3.15,-4.35,114.012417473262));
#61855=CARTESIAN_POINT('',(3.15,0.,114.012417473262));
#61856=CARTESIAN_POINT('',(3.15,-4.35,86.5380363299847));
#61857=CARTESIAN_POINT('Origin',(3.15,0.,114.012417473262));
#61858=CARTESIAN_POINT('',(-8.99393596021693,-4.35,109.592386256909));
#61859=CARTESIAN_POINT('Origin',(3.075,4.425,87.4805141260616));
#61860=CARTESIAN_POINT('',(3.,4.5,87.4805141260616));
#61861=CARTESIAN_POINT('',(3.15,4.35,87.4805141260616));
#61862=CARTESIAN_POINT('Origin',(4.55,0.,114.991292292766));
#61863=CARTESIAN_POINT('',(3.15,-4.35,115.500850620739));
#61864=CARTESIAN_POINT('',(3.15,0.,115.500850620739));
#61865=CARTESIAN_POINT('',(9.47800256154818,-4.35,113.197646045975));
#61866=CARTESIAN_POINT('Origin',(3.15,0.,115.500850620739));
#61867=CARTESIAN_POINT('',(3.15,-4.35,115.897373065416));
#61868=CARTESIAN_POINT('',(3.15,0.,115.897373065416));
#61869=CARTESIAN_POINT('',(3.15,-4.35,87.4805141260616));
#61870=CARTESIAN_POINT('Origin',(3.15,0.,115.897373065416));
#61871=CARTESIAN_POINT('',(-9.29684248507857,-4.35,111.367092890248));
#61872=CARTESIAN_POINT('Origin',(3.075,4.425,88.4229919221386));
#61873=CARTESIAN_POINT('',(3.,4.5,88.4229919221386));
#61874=CARTESIAN_POINT('',(3.15,4.35,88.4229919221386));
#61875=CARTESIAN_POINT('Origin',(4.55,0.,116.87624788492));
#61876=CARTESIAN_POINT('',(3.15,-4.35,117.385806212893));
#61877=CARTESIAN_POINT('',(3.15,0.,117.385806212893));
#61878=CARTESIAN_POINT('',(9.78090908640965,-4.35,114.972352679314));
#61879=CARTESIAN_POINT('Origin',(3.15,0.,117.385806212893));
#61880=CARTESIAN_POINT('',(3.15,-4.35,88.4229919221386));
#61881=CARTESIAN_POINT('Origin',(4.5,4.5,59.4601776313845));
#61882=CARTESIAN_POINT('',(4.35,4.5,112.723852828099));
#61883=CARTESIAN_POINT('',(4.35,4.5,59.4601776313845));
#61884=CARTESIAN_POINT('',(3.,4.5,112.23249301184));
#61885=CARTESIAN_POINT('',(-4.7687324598368,4.5,109.404905638482));
#61886=CARTESIAN_POINT('',(3.,4.5,111.6259083057));
#61887=CARTESIAN_POINT('',(3.,4.5,85.5955585339077));
#61888=CARTESIAN_POINT('',(4.35,4.5,111.13454848944));
#61889=CARTESIAN_POINT('',(12.7944864873441,4.5,108.061006764384));
#61890=CARTESIAN_POINT('',(4.35,4.5,110.838897235946));
#61891=CARTESIAN_POINT('',(4.35,4.5,59.4601776313845));
#61892=CARTESIAN_POINT('',(3.,4.5,110.347537419686));
#61893=CARTESIAN_POINT('',(-4.46582593497534,4.5,107.630199005142));
#61894=CARTESIAN_POINT('',(3.,4.5,109.740952713546));
#61895=CARTESIAN_POINT('',(3.,4.5,84.6530807378308));
#61896=CARTESIAN_POINT('',(4.35,4.5,109.249592897286));
#61897=CARTESIAN_POINT('',(12.4915799624826,4.5,106.286300131044));
#61898=CARTESIAN_POINT('',(4.35,4.5,108.953941643792));
#61899=CARTESIAN_POINT('',(4.35,4.5,59.4601776313845));
#61900=CARTESIAN_POINT('',(3.,4.5,108.462581827532));
#61901=CARTESIAN_POINT('',(-4.16291941011368,4.5,105.855492371803));
#61902=CARTESIAN_POINT('',(3.,4.5,107.855997121392));
#61903=CARTESIAN_POINT('',(3.,4.5,83.7106029417538));
#61904=CARTESIAN_POINT('',(4.35,4.5,107.364637305132));
#61905=CARTESIAN_POINT('',(12.1886734376211,4.5,104.511593497705));
#61906=CARTESIAN_POINT('',(4.35,4.5,107.068986051638));
#61907=CARTESIAN_POINT('',(4.35,4.5,59.4601776313845));
#61908=CARTESIAN_POINT('',(3.,4.5,106.577626235378));
#61909=CARTESIAN_POINT('',(-3.86001288525238,4.5,104.080785738464));
#61910=CARTESIAN_POINT('',(3.,4.5,105.971041529238));
#61911=CARTESIAN_POINT('',(3.,4.5,82.7681251456769));
#61912=CARTESIAN_POINT('',(4.35,4.5,105.479681712978));
#61913=CARTESIAN_POINT('',(11.8857669127596,4.5,102.736886864366));
#61914=CARTESIAN_POINT('',(4.35,4.5,105.184030459484));
#61915=CARTESIAN_POINT('',(4.35,4.5,59.4601776313845));
#61916=CARTESIAN_POINT('',(3.,4.5,104.692670643225));
#61917=CARTESIAN_POINT('',(-3.55710636039092,4.5,102.306079105125));
#61918=CARTESIAN_POINT('',(3.,4.5,104.086085937084));
#61919=CARTESIAN_POINT('',(3.,4.5,81.8256473496));
#61920=CARTESIAN_POINT('',(4.35,4.5,103.594726120825));
#61921=CARTESIAN_POINT('',(11.5828603878982,4.5,100.962180231027));
#61922=CARTESIAN_POINT('',(4.35,4.5,103.29907486733));
#61923=CARTESIAN_POINT('',(4.35,4.5,59.4601776313845));
#61924=CARTESIAN_POINT('',(3.,4.5,102.807715051071));
#61925=CARTESIAN_POINT('',(-3.25419983552944,4.5,100.531372471785));
#61926=CARTESIAN_POINT('',(3.,4.5,102.20113034493));
#61927=CARTESIAN_POINT('',(3.,4.5,80.883169553523));
#61928=CARTESIAN_POINT('',(4.35,4.5,101.709770528671));
#61929=CARTESIAN_POINT('',(11.2799538630365,4.5,99.1874735976874));
#61930=CARTESIAN_POINT('',(4.35,4.5,101.414119275176));
#61931=CARTESIAN_POINT('',(4.35,4.5,59.4601776313845));
#61932=CARTESIAN_POINT('',(3.,4.5,100.922759458917));
#61933=CARTESIAN_POINT('',(-2.95129331066782,4.5,98.7566658384461));
#61934=CARTESIAN_POINT('',(3.,4.5,100.316174752776));
#61935=CARTESIAN_POINT('',(3.,4.5,79.9406917574461));
#61936=CARTESIAN_POINT('',(10.9770473381751,4.5,97.4127669643481));
#61937=CARTESIAN_POINT('',(3.,4.5,78.9982139613691));
#61938=CARTESIAN_POINT('',(3.,4.5,78.0557361652922));
#61939=CARTESIAN_POINT('',(3.,4.5,94.6613079763146));
#61940=CARTESIAN_POINT('',(3.,4.5,77.1132583692153));
#61941=CARTESIAN_POINT('',(4.35,4.5,94.1699481600552));
#61942=CARTESIAN_POINT('',(10.0683277635907,4.5,92.0886470643302));
#61943=CARTESIAN_POINT('',(4.35,4.5,93.8742969065607));
#61944=CARTESIAN_POINT('',(4.35,4.5,59.4601776313845));
#61945=CARTESIAN_POINT('',(3.,4.5,93.3829370903013));
#61946=CARTESIAN_POINT('',(-1.73966721122195,4.5,91.657839305089));
#61947=CARTESIAN_POINT('',(3.,4.5,92.7763523841607));
#61948=CARTESIAN_POINT('',(3.,4.5,76.1707805731383));
#61949=CARTESIAN_POINT('',(4.35,4.5,92.2849925679014));
#61950=CARTESIAN_POINT('',(9.76542123872922,4.5,90.3139404309909));
#61951=CARTESIAN_POINT('',(4.35,4.5,91.9893413144068));
#61952=CARTESIAN_POINT('',(4.35,4.5,59.4601776313845));
#61953=CARTESIAN_POINT('',(3.,4.5,91.4979814981474));
#61954=CARTESIAN_POINT('',(-1.43676068636049,4.5,89.8831326717497));
#61955=CARTESIAN_POINT('',(3.,4.5,90.8913967920069));
#61956=CARTESIAN_POINT('',(3.,4.5,75.2283027770614));
#61957=CARTESIAN_POINT('',(4.35,4.5,90.4000369757475));
#61958=CARTESIAN_POINT('',(9.46251471386775,4.5,88.5392337976516));
#61959=CARTESIAN_POINT('',(4.35,4.5,90.1043857222529));
#61960=CARTESIAN_POINT('',(4.35,4.5,59.4601776313845));
#61961=CARTESIAN_POINT('',(3.,4.5,89.6130259059935));
#61962=CARTESIAN_POINT('',(-1.13385416149902,4.5,88.1084260384104));
#61963=CARTESIAN_POINT('',(3.,4.5,89.006441199853));
#61964=CARTESIAN_POINT('',(3.,4.5,74.2858249809845));
#61965=CARTESIAN_POINT('',(4.35,4.5,88.5150813835936));
#61966=CARTESIAN_POINT('',(9.15960818900628,4.5,86.7645271643124));
#61967=CARTESIAN_POINT('',(4.35,4.5,88.219430130099));
#61968=CARTESIAN_POINT('',(4.35,4.5,59.4601776313845));
#61969=CARTESIAN_POINT('',(3.,4.5,87.7280703138397));
#61970=CARTESIAN_POINT('',(-0.830947636637549,4.5,86.3337194050711));
#61971=CARTESIAN_POINT('',(3.,4.5,87.1214856076991));
#61972=CARTESIAN_POINT('',(3.,4.5,73.3433471849075));
#61973=CARTESIAN_POINT('',(4.35,4.5,86.6301257914397));
#61974=CARTESIAN_POINT('',(8.85670166414481,4.5,84.9898205309731));
#61975=CARTESIAN_POINT('',(4.35,4.5,86.3344745379451));
#61976=CARTESIAN_POINT('',(4.35,4.5,59.4601776313845));
#61977=CARTESIAN_POINT('',(3.,4.5,85.8431147216858));
#61978=CARTESIAN_POINT('',(-0.528041111776089,4.5,84.5590127717318));
#61979=CARTESIAN_POINT('',(3.,4.5,85.2365300155452));
#61980=CARTESIAN_POINT('',(3.,4.5,72.4008693888306));
#61981=CARTESIAN_POINT('',(4.35,4.5,84.7451701992859));
#61982=CARTESIAN_POINT('',(8.55379513928335,4.5,83.2151138976338));
#61983=CARTESIAN_POINT('',(4.35,4.5,84.4495189457913));
#61984=CARTESIAN_POINT('',(4.35,4.5,59.4601776313845));
#61985=CARTESIAN_POINT('',(3.,4.5,83.9581591295319));
#61986=CARTESIAN_POINT('',(-0.225134586914621,4.5,82.7843061383926));
#61987=CARTESIAN_POINT('',(3.,4.5,83.3515744233914));
#61988=CARTESIAN_POINT('',(3.,4.5,71.4583915927537));
#61989=CARTESIAN_POINT('',(8.25088861442188,4.5,81.4404072642945));
#61990=CARTESIAN_POINT('',(3.,4.5,70.5159137966767));
#61991=CARTESIAN_POINT('',(3.,4.5,69.5734360005998));
#61992=CARTESIAN_POINT('',(3.,4.5,68.6309582045228));
#61993=CARTESIAN_POINT('',(3.,4.5,67.6884804084459));
#61994=CARTESIAN_POINT('',(3.,4.5,74.5333811687625));
#61995=CARTESIAN_POINT('',(1.28939803739271,4.5,73.9107729716961));
#61996=CARTESIAN_POINT('',(3.,4.5,66.746002612369));
#61997=CARTESIAN_POINT('',(3.,4.5,65.803524816292));
#61998=CARTESIAN_POINT('',(3.,4.5,64.8610470202151));
#61999=CARTESIAN_POINT('',(4.35,4.5,59.4601776313845));
#62000=CARTESIAN_POINT('',(3.,4.5,129.197093341225));
#62001=CARTESIAN_POINT('',(-7.49489118358982,4.5,125.377265338535));
#62002=CARTESIAN_POINT('',(3.,4.5,128.590508635084));
#62003=CARTESIAN_POINT('',(3.,4.5,94.0778586986002));
#62004=CARTESIAN_POINT('',(4.35,4.5,128.099148818825));
#62005=CARTESIAN_POINT('',(15.5206452110971,4.5,124.033366464437));
#62006=CARTESIAN_POINT('',(4.35,4.5,127.80349756533));
#62007=CARTESIAN_POINT('',(4.35,4.5,59.4601776313845));
#62008=CARTESIAN_POINT('',(3.,4.5,127.312137749071));
#62009=CARTESIAN_POINT('',(-7.19198465872859,4.5,123.602558705196));
#62010=CARTESIAN_POINT('',(3.,4.5,93.1353809025232));
#62011=CARTESIAN_POINT('',(3.,4.5,92.1929031064463));
#62012=CARTESIAN_POINT('',(3.,4.5,91.2504253103694));
#62013=CARTESIAN_POINT('',(3.,4.5,90.3079475142924));
#62014=CARTESIAN_POINT('',(3.,4.5,89.3654697182155));
#62015=CARTESIAN_POINT('Origin',(3.075,4.425,89.3654697182155));
#62016=CARTESIAN_POINT('',(3.15,4.35,89.3654697182155));
#62017=CARTESIAN_POINT('Origin',(3.15,0.,119.270761805046));
#62018=CARTESIAN_POINT('',(3.15,-4.35,119.667284249724));
#62019=CARTESIAN_POINT('',(3.15,0.,119.667284249724));
#62020=CARTESIAN_POINT('',(3.15,-4.35,89.3654697182155));
#62021=CARTESIAN_POINT('Origin',(3.15,0.,119.667284249724));
#62022=CARTESIAN_POINT('',(-9.90265553480133,-4.35,114.916506156926));
#62023=CARTESIAN_POINT('Origin',(3.075,4.425,90.3079475142924));
#62024=CARTESIAN_POINT('',(3.15,4.35,90.3079475142924));
#62025=CARTESIAN_POINT('Origin',(4.55,0.,120.646159069228));
#62026=CARTESIAN_POINT('',(3.15,-4.35,121.1557173972));
#62027=CARTESIAN_POINT('',(3.15,0.,121.1557173972));
#62028=CARTESIAN_POINT('',(10.3867221361326,-4.35,118.521765945993));
#62029=CARTESIAN_POINT('Origin',(3.15,0.,121.1557173972));
#62030=CARTESIAN_POINT('',(3.15,-4.35,121.552239841878));
#62031=CARTESIAN_POINT('',(3.15,0.,121.552239841878));
#62032=CARTESIAN_POINT('',(3.15,-4.35,90.3079475142924));
#62033=CARTESIAN_POINT('Origin',(3.15,0.,121.552239841878));
#62034=CARTESIAN_POINT('',(-10.205562059663,-4.35,116.691212790265));
#62035=CARTESIAN_POINT('Origin',(3.075,4.425,91.2504253103694));
#62036=CARTESIAN_POINT('',(3.15,4.35,91.2504253103694));
#62037=CARTESIAN_POINT('Origin',(4.55,0.,122.531114661382));
#62038=CARTESIAN_POINT('',(3.15,-4.35,123.040672989354));
#62039=CARTESIAN_POINT('',(3.15,0.,123.040672989354));
#62040=CARTESIAN_POINT('',(10.6896286609941,-4.35,120.296472579332));
#62041=CARTESIAN_POINT('Origin',(3.15,0.,123.040672989354));
#62042=CARTESIAN_POINT('',(3.15,-4.35,123.437195434032));
#62043=CARTESIAN_POINT('',(3.15,0.,123.437195434032));
#62044=CARTESIAN_POINT('',(3.15,-4.35,91.2504253103694));
#62045=CARTESIAN_POINT('Origin',(3.15,0.,123.437195434032));
#62046=CARTESIAN_POINT('',(-10.5084685845245,-4.35,118.465919423605));
#62047=CARTESIAN_POINT('Origin',(3.075,4.425,92.1929031064463));
#62048=CARTESIAN_POINT('',(3.15,4.35,92.1929031064463));
#62049=CARTESIAN_POINT('Origin',(4.55,0.,124.416070253535));
#62050=CARTESIAN_POINT('',(3.15,-4.35,124.925628581508));
#62051=CARTESIAN_POINT('',(3.15,0.,124.925628581508));
#62052=CARTESIAN_POINT('',(10.9925351858555,-4.35,122.071179212671));
#62053=CARTESIAN_POINT('Origin',(3.15,0.,124.925628581508));
#62054=CARTESIAN_POINT('',(3.15,-4.35,125.322151026186));
#62055=CARTESIAN_POINT('',(3.15,0.,125.322151026186));
#62056=CARTESIAN_POINT('',(3.15,-4.35,92.1929031064463));
#62057=CARTESIAN_POINT('Origin',(3.15,0.,125.322151026186));
#62058=CARTESIAN_POINT('',(-10.8113751093857,-4.35,120.240626056944));
#62059=CARTESIAN_POINT('Origin',(3.075,4.425,93.1353809025232));
#62060=CARTESIAN_POINT('',(3.15,4.35,127.20710661834));
#62061=CARTESIAN_POINT('',(6.34023534238099,1.159764657619,124.973279782941));
#62062=CARTESIAN_POINT('',(3.15,4.35,93.1353809025232));
#62063=CARTESIAN_POINT('Origin',(4.55,0.,126.301025845689));
#62064=CARTESIAN_POINT('',(3.15,-4.35,126.810584173662));
#62065=CARTESIAN_POINT('',(3.15,0.,126.810584173662));
#62066=CARTESIAN_POINT('',(11.295441710717,-4.35,123.845885846011));
#62067=CARTESIAN_POINT('Origin',(3.15,0.,126.810584173662));
#62068=CARTESIAN_POINT('',(3.15,-4.35,127.20710661834));
#62069=CARTESIAN_POINT('',(3.15,0.,127.20710661834));
#62070=CARTESIAN_POINT('',(3.15,-4.35,93.1353809025232));
#62071=CARTESIAN_POINT('Origin',(-4.17803300858899,1.125,144.907144622795));
#62072=CARTESIAN_POINT('',(-4.04999999999999,4.2,144.960177631385));
#62073=CARTESIAN_POINT('',(-4.30606601717799,4.30606601717799,144.854111614207));
#62074=CARTESIAN_POINT('',(-1.33270642526082,3.07446014839374,146.085717482991));
#62075=CARTESIAN_POINT('',(-4.30606601717799,-4.30606601717799,144.854111614207));
#62076=CARTESIAN_POINT('',(-4.30606601717798,1.125,144.854111614207));
#62077=CARTESIAN_POINT('',(-4.04999999999999,-4.2,144.960177631385));
#62078=CARTESIAN_POINT('',(-2.66093885398715,-3.62463203435597,145.535545597029));
#62079=CARTESIAN_POINT('',(-4.04999999999999,1.125,144.960177631385));
#62080=CARTESIAN_POINT('Origin',(-2.25,-4.35,144.810177631385));
#62081=CARTESIAN_POINT('',(-4.39393398282201,-4.39393398282201,144.766243648562));
#62082=CARTESIAN_POINT('',(-4.2,-4.2,144.960177631385));
#62083=CARTESIAN_POINT('',(-3.375,-4.39393398282201,144.766243648562));
#62084=CARTESIAN_POINT('',(4.2,-4.2,144.960177631385));
#62085=CARTESIAN_POINT('',(4.2,-4.2,144.960177631385));
#62086=CARTESIAN_POINT('',(-2.25,-4.2,144.960177631385));
#62087=CARTESIAN_POINT('Origin',(-4.35,2.25,144.810177631385));
#62088=CARTESIAN_POINT('',(-4.2,4.2,144.960177631385));
#62089=CARTESIAN_POINT('',(-4.39393398282201,3.375,144.766243648562));
#62090=CARTESIAN_POINT('Origin',(-4.44696699141101,3.375,144.638210639973));
#62091=CARTESIAN_POINT('',(-4.425,-4.425,144.691243648562));
#62092=CARTESIAN_POINT('',(-3.87891329166412,-3.87891329166412,146.009613586059));
#62093=CARTESIAN_POINT('',(-4.5,-4.35,144.510177631384));
#62094=CARTESIAN_POINT('',(-4.5,3.375,144.510177631384));
#62095=CARTESIAN_POINT('',(-18.0749958490139,9.22499584901393,111.737238543536));
#62096=CARTESIAN_POINT('Origin',(-3.375,-4.44696699141101,144.638210639973));
#62097=CARTESIAN_POINT('',(-4.35,-4.5,144.510177631384));
#62098=CARTESIAN_POINT('',(8.7938747634856,-17.6438747634856,112.778056915244));
#62099=CARTESIAN_POINT('',(4.35,-4.5,144.510177631384));
#62100=CARTESIAN_POINT('',(-3.375,-4.5,144.510177631384));
#62101=CARTESIAN_POINT('',(-9.22499584901393,-18.0749958490139,111.737238543536));
#62102=CARTESIAN_POINT('Origin',(-4.425,-4.425,59.4601776313845));
#62103=CARTESIAN_POINT('',(-4.35,-4.5,59.9101776313845));
#62104=CARTESIAN_POINT('',(-4.38982461147609,-4.46017538852391,59.8140325142427));
#62105=CARTESIAN_POINT('',(-4.35,-4.5,59.4601776313845));
#62106=CARTESIAN_POINT('',(-4.5,-4.35,59.4601776313845));
#62107=CARTESIAN_POINT('Origin',(4.42952305344106,-2.25,129.632770516003));
#62108=CARTESIAN_POINT('',(4.42952305344107,-4.42047694655894,129.632770516003));
#62109=CARTESIAN_POINT('',(-7.70722990181154,-16.5572299018115,112.299690974637));
#62110=CARTESIAN_POINT('',(4.35904610688212,-4.35,129.532119005254));
#62111=CARTESIAN_POINT('',(1.17648980366091,-1.16744369677909,124.986957564464));
#62112=CARTESIAN_POINT('',(4.35904610688212,4.35,129.532119005254));
#62113=CARTESIAN_POINT('',(4.35904610688212,-2.25,129.532119005254));
#62114=CARTESIAN_POINT('',(1.36698986321579,1.35794375633333,125.259019844801));
#62115=CARTESIAN_POINT('Origin',(-7.46923967284039,4.425,125.306788391976));
#62116=CARTESIAN_POINT('',(3.15,4.35,129.092062210493));
#62117=CARTESIAN_POINT('',(-7.44358816209097,4.35,125.236311445418));
#62118=CARTESIAN_POINT('',(3.15,4.35,129.092062210493));
#62119=CARTESIAN_POINT('Origin',(4.42952305344106,-2.25,128.154831460306));
#62120=CARTESIAN_POINT('',(4.42952305344106,-4.42047694655895,128.154831460306));
#62121=CARTESIAN_POINT('',(4.5,-4.35,128.054179949556));
#62122=CARTESIAN_POINT('',(16.8400831031941,7.99008310319415,110.430714862697));
#62123=CARTESIAN_POINT('',(4.5,4.35,128.054179949556));
#62124=CARTESIAN_POINT('',(4.5,-2.25,128.054179949556));
#62125=CARTESIAN_POINT('',(4.42952305344105,4.42047694655895,128.154831460306));
#62126=CARTESIAN_POINT('',(17.3970680155514,-8.54706801555143,109.635257970328));
#62127=CARTESIAN_POINT('',(4.35904610688211,4.35,128.255482971055));
#62128=CARTESIAN_POINT('',(5.69650657059256,5.68746046371058,126.345391475711));
#62129=CARTESIAN_POINT('',(4.35904610688211,-4.35,128.255482971055));
#62130=CARTESIAN_POINT('',(4.35904610688211,-2.25,128.255482971055));
#62131=CARTESIAN_POINT('',(5.50600651103787,-5.49696040415596,126.617453756048));
#62132=CARTESIAN_POINT('Origin',(15.5462967218465,4.425,124.103843410996));
#62133=CARTESIAN_POINT('',(-3.56830707166375,12.4183070716637,122.554690517387));
#62134=CARTESIAN_POINT('',(3.15,4.35,128.695539765816));
#62135=CARTESIAN_POINT('',(3.15,4.35,128.695539765816));
#62136=CARTESIAN_POINT('',(15.5719482325959,4.35,124.174320357555));
#62137=CARTESIAN_POINT('Origin',(4.425,4.425,59.4601776313845));
#62138=CARTESIAN_POINT('',(4.5,4.35,127.848466434599));
#62139=CARTESIAN_POINT('',(4.5,4.35,59.4601776313845));
#62140=CARTESIAN_POINT('',(4.42952305344106,4.42047694655894,127.74781492385));
#62141=CARTESIAN_POINT('',(-6.81704478554588,15.6670447855459,111.686051481911));
#62142=CARTESIAN_POINT('',(12.2916539293204,-3.44165392932035,122.242691618166));
#62143=CARTESIAN_POINT('Origin',(4.5,-4.5,59.4601776313845));
#62144=CARTESIAN_POINT('',(4.5,-4.35,127.848466434599));
#62145=CARTESIAN_POINT('',(4.5,-4.35,59.4601776313845));
#62146=CARTESIAN_POINT('',(4.5,-2.25,127.848466434599));
#62147=CARTESIAN_POINT('Origin',(4.42952305344106,-2.25,127.74781492385));
#62148=CARTESIAN_POINT('',(4.42952305344107,-4.42047694655893,127.74781492385));
#62149=CARTESIAN_POINT('',(-7.37402969790322,-16.2240296979032,110.890594589543));
#62150=CARTESIAN_POINT('',(4.35904610688211,-4.35,127.6471634131));
#62151=CARTESIAN_POINT('',(1.23347039440895,-1.22442428752731,123.18337868941));
#62152=CARTESIAN_POINT('',(4.35904610688211,4.35,127.6471634131));
#62153=CARTESIAN_POINT('',(4.35904610688211,-2.25,127.6471634131));
#62154=CARTESIAN_POINT('',(1.42397045396367,1.41492434708228,123.455440969748));
#62155=CARTESIAN_POINT('Origin',(-7.16633314797917,4.425,123.532081758637));
#62156=CARTESIAN_POINT('',(-7.14068163722974,4.35,123.461604812078));
#62157=CARTESIAN_POINT('Origin',(3.15,0.,127.20710661834));
#62158=CARTESIAN_POINT('',(-11.1142816342474,-4.35,122.015332690283));
#62159=CARTESIAN_POINT('Origin',(3.075,4.425,94.0778586986002));
#62160=CARTESIAN_POINT('',(3.15,4.35,94.0778586986002));
#62161=CARTESIAN_POINT('Origin',(4.55,0.,128.185981437843));
#62162=CARTESIAN_POINT('',(3.15,-4.35,128.695539765816));
#62163=CARTESIAN_POINT('',(3.15,0.,128.695539765816));
#62164=CARTESIAN_POINT('',(11.5983482355782,-4.35,125.62059247935));
#62165=CARTESIAN_POINT('Origin',(3.15,0.,128.695539765816));
#62166=CARTESIAN_POINT('',(3.15,-4.35,129.092062210493));
#62167=CARTESIAN_POINT('',(3.15,0.,129.092062210493));
#62168=CARTESIAN_POINT('',(3.15,-4.35,94.0778586986002));
#62169=CARTESIAN_POINT('Origin',(3.15,0.,129.092062210493));
#62170=CARTESIAN_POINT('',(-11.4171881591087,-4.35,123.790039323623));
#62171=CARTESIAN_POINT('Origin',(3.075,4.425,64.8610470202151));
#62172=CARTESIAN_POINT('',(3.15,4.35,64.8610470202151));
#62173=CARTESIAN_POINT('Origin',(3.15,0.,70.2619164090457));
#62174=CARTESIAN_POINT('',(3.15,-4.35,70.6584388537233));
#62175=CARTESIAN_POINT('',(3.15,0.,70.6584388537233));
#62176=CARTESIAN_POINT('',(3.15,-4.35,64.8610470202151));
#62177=CARTESIAN_POINT('Origin',(3.15,0.,70.6584388537233));
#62178=CARTESIAN_POINT('',(-2.0270858884032,-4.35,68.7741336901049));
#62179=CARTESIAN_POINT('Origin',(3.075,4.425,65.803524816292));
#62180=CARTESIAN_POINT('',(3.15,4.35,65.803524816292));
#62181=CARTESIAN_POINT('Origin',(4.55,0.,71.6373136732269));
#62182=CARTESIAN_POINT('',(3.15,-4.35,72.1468720011996));
#62183=CARTESIAN_POINT('',(3.15,0.,72.1468720011996));
#62184=CARTESIAN_POINT('',(2.51115248973423,-4.35,72.3793934791714));
#62185=CARTESIAN_POINT('Origin',(3.15,0.,72.1468720011996));
#62186=CARTESIAN_POINT('',(3.15,-4.35,72.5433944458772));
#62187=CARTESIAN_POINT('',(3.15,0.,72.5433944458772));
#62188=CARTESIAN_POINT('',(3.15,-4.35,65.803524816292));
#62189=CARTESIAN_POINT('Origin',(3.15,0.,72.5433944458772));
#62190=CARTESIAN_POINT('',(-2.32999241326467,-4.35,70.5488403234442));
#62191=CARTESIAN_POINT('Origin',(1.31504954814214,4.425,73.8402960251372));
#62192=CARTESIAN_POINT('',(3.15,4.35,74.4283500380311));
#62193=CARTESIAN_POINT('Origin',(3.075,4.425,66.746002612369));
#62194=CARTESIAN_POINT('',(3.15,4.35,66.746002612369));
#62195=CARTESIAN_POINT('Origin',(4.55,0.,73.5222692653807));
#62196=CARTESIAN_POINT('',(3.15,-4.35,74.0318275933534));
#62197=CARTESIAN_POINT('',(3.15,0.,74.0318275933534));
#62198=CARTESIAN_POINT('',(2.8140590145957,-4.35,74.1541001125106));
#62199=CARTESIAN_POINT('Origin',(3.15,0.,74.0318275933534));
#62200=CARTESIAN_POINT('',(3.15,-4.35,66.746002612369));
#62201=CARTESIAN_POINT('Origin',(3.075,4.425,67.6884804084459));
#62202=CARTESIAN_POINT('',(3.15,4.35,67.6884804084459));
#62203=CARTESIAN_POINT('Origin',(3.15,0.,75.9167831855073));
#62204=CARTESIAN_POINT('',(3.15,-4.35,76.3133056301849));
#62205=CARTESIAN_POINT('',(3.15,0.,76.3133056301849));
#62206=CARTESIAN_POINT('',(3.15,-4.35,67.6884804084459));
#62207=CARTESIAN_POINT('Origin',(3.15,0.,76.3133056301849));
#62208=CARTESIAN_POINT('',(-2.9358054629876,-4.35,74.0982535901228));
#62209=CARTESIAN_POINT('Origin',(3.075,4.425,68.6309582045228));
#62210=CARTESIAN_POINT('',(3.15,4.35,68.6309582045228));
#62211=CARTESIAN_POINT('Origin',(4.55,0.,77.2921804496885));
#62212=CARTESIAN_POINT('',(3.15,-4.35,77.8017387776612));
#62213=CARTESIAN_POINT('',(3.15,0.,77.8017387776612));
#62214=CARTESIAN_POINT('',(3.41987206431863,-4.35,77.7035133791892));
#62215=CARTESIAN_POINT('Origin',(3.15,0.,77.8017387776612));
#62216=CARTESIAN_POINT('',(3.15,-4.35,68.6309582045228));
#62217=CARTESIAN_POINT('Origin',(3.075,4.425,69.5734360005998));
#62218=CARTESIAN_POINT('',(3.15,4.35,69.5734360005998));
#62219=CARTESIAN_POINT('Origin',(3.15,0.,79.6866943698151));
#62220=CARTESIAN_POINT('',(3.15,-4.35,80.0832168144927));
#62221=CARTESIAN_POINT('',(3.15,0.,80.0832168144927));
#62222=CARTESIAN_POINT('',(3.15,-4.35,69.5734360005998));
#62223=CARTESIAN_POINT('Origin',(3.15,0.,80.0832168144927));
#62224=CARTESIAN_POINT('',(-3.54161851271054,-4.35,77.6476668568014));
#62225=CARTESIAN_POINT('Origin',(3.075,4.425,70.5159137966767));
#62226=CARTESIAN_POINT('',(3.15,4.35,70.5159137966767));
#62227=CARTESIAN_POINT('Origin',(4.55,0.,81.0620916339962));
#62228=CARTESIAN_POINT('',(3.15,-4.35,81.5716499619689));
#62229=CARTESIAN_POINT('',(3.15,0.,81.5716499619689));
#62230=CARTESIAN_POINT('',(4.02568511404156,-4.35,81.2529266458678));
#62231=CARTESIAN_POINT('Origin',(3.15,0.,81.5716499619689));
#62232=CARTESIAN_POINT('',(3.15,-4.35,81.9681724066466));
#62233=CARTESIAN_POINT('',(3.15,0.,81.9681724066466));
#62234=CARTESIAN_POINT('',(3.15,-4.35,70.5159137966767));
#62235=CARTESIAN_POINT('Origin',(3.15,0.,81.9681724066466));
#62236=CARTESIAN_POINT('',(-3.844525037572,-4.35,79.4223734901407));
#62237=CARTESIAN_POINT('Origin',(4.42952305344105,-2.25,94.2256308015361));
#62238=CARTESIAN_POINT('',(4.42952305344106,-4.42047694655894,94.2256308015361));
#62239=CARTESIAN_POINT('',(4.5,-4.35,94.1249792907867));
#62240=CARTESIAN_POINT('',(10.8424794328446,1.99247943284463,85.0669799309673));
#62241=CARTESIAN_POINT('',(4.5,4.35,94.1249792907867));
#62242=CARTESIAN_POINT('',(4.5,-2.25,94.1249792907867));
#62243=CARTESIAN_POINT('',(4.42952305344106,4.42047694655895,94.2256308015361));
#62244=CARTESIAN_POINT('',(11.399464345202,-2.54946434520197,84.2715230385988));
#62245=CARTESIAN_POINT('',(4.35904610688211,4.35,94.3262823122855));
#62246=CARTESIAN_POINT('',(4.67085593712091,4.66180983023882,93.8809717247474));
#62247=CARTESIAN_POINT('',(4.35904610688211,-4.35,94.3262823122855));
#62248=CARTESIAN_POINT('',(4.35904610688211,-2.25,94.3262823122855));
#62249=CARTESIAN_POINT('',(4.48035587756627,-4.47130977068416,94.1530340050846));
#62250=CARTESIAN_POINT('Origin',(10.0939792743401,4.425,92.1591240108891));
#62251=CARTESIAN_POINT('',(0.385993158017769,8.46400684198224,91.394320687785));
#62252=CARTESIAN_POINT('',(3.15,4.35,94.7663391070461));
#62253=CARTESIAN_POINT('',(3.15,4.35,94.7663391070461));
#62254=CARTESIAN_POINT('',(10.1196307850895,4.35,92.2296009574481));
#62255=CARTESIAN_POINT('Origin',(4.425,4.425,59.4601776313845));
#62256=CARTESIAN_POINT('',(4.5,4.35,93.9192657758292));
#62257=CARTESIAN_POINT('',(4.5,4.35,59.4601776313845));
#62258=CARTESIAN_POINT('',(4.42952305344104,4.42047694655896,93.8186142650798));
#62259=CARTESIAN_POINT('',(-0.819441115196317,9.66944111519632,86.32231655018));
#62260=CARTESIAN_POINT('',(8.33735369963672,0.512646300363287,91.0823217885672));
#62261=CARTESIAN_POINT('Origin',(4.5,-4.5,59.4601776313845));
#62262=CARTESIAN_POINT('',(4.5,-4.35,93.9192657758292));
#62263=CARTESIAN_POINT('',(4.5,-4.35,59.4601776313845));
#62264=CARTESIAN_POINT('',(4.5,-2.25,93.9192657758292));
#62265=CARTESIAN_POINT('Origin',(4.42952305344105,-2.25,93.8186142650798));
#62266=CARTESIAN_POINT('',(4.42952305344105,-4.42047694655895,93.8186142650798));
#62267=CARTESIAN_POINT('',(-1.37642602755366,-10.2264260275537,85.5268596578114));
#62268=CARTESIAN_POINT('',(4.35904610688211,-4.35,93.7179627543304));
#62269=CARTESIAN_POINT('',(2.25912102788096,-2.25007492099894,90.7189589384473));
#62270=CARTESIAN_POINT('',(4.35904610688211,4.35,93.7179627543304));
#62271=CARTESIAN_POINT('',(4.35904610688211,-2.25,93.7179627543304));
#62272=CARTESIAN_POINT('',(2.44962108743568,2.44057498055347,90.9910212187846));
#62273=CARTESIAN_POINT('Origin',(-1.71401570047253,4.425,91.58736235853));
#62274=CARTESIAN_POINT('',(3.15,4.35,93.2779059595698));
#62275=CARTESIAN_POINT('',(-1.6883641897231,4.35,91.5168854119711));
#62276=CARTESIAN_POINT('',(3.15,4.35,93.2779059595698));
#62277=CARTESIAN_POINT('Origin',(4.42952305344106,-2.25,92.3406752093822));
#62278=CARTESIAN_POINT('',(4.42952305344104,-4.42047694655896,92.3406752093823));
#62279=CARTESIAN_POINT('',(4.5,-4.35,92.2400236986328));
#62280=CARTESIAN_POINT('',(10.5092792289363,1.65927922893628,83.6578835458703));
#62281=CARTESIAN_POINT('',(4.5,4.35,92.2400236986328));
#62282=CARTESIAN_POINT('',(4.5,-2.25,92.2400236986328));
#62283=CARTESIAN_POINT('',(4.42952305344105,4.42047694655895,92.3406752093823));
#62284=CARTESIAN_POINT('',(11.0662641412936,-2.21626414129357,82.8624266535018));
#62285=CARTESIAN_POINT('',(4.35904610688211,4.35,92.4413267201317));
#62286=CARTESIAN_POINT('',(4.61387534637246,4.60482923949037,92.0773928496939));
#62287=CARTESIAN_POINT('',(4.35904610688212,-4.35,92.4413267201317));
#62288=CARTESIAN_POINT('',(4.35904610688211,-2.25,92.4413267201317));
#62289=CARTESIAN_POINT('',(4.42337528681781,-4.4143291799357,92.3494551300312));
#62290=CARTESIAN_POINT('Origin',(9.79107274947864,4.425,90.3844173775499));
#62291=CARTESIAN_POINT('',(0.605676504110624,8.24432349588938,89.663189030584));
#62292=CARTESIAN_POINT('',(3.15,4.35,92.8813835148922));
#62293=CARTESIAN_POINT('',(3.15,4.35,92.8813835148922));
#62294=CARTESIAN_POINT('',(9.81672426022806,4.35,90.4548943241088));
#62295=CARTESIAN_POINT('Origin',(4.425,4.425,59.4601776313845));
#62296=CARTESIAN_POINT('',(4.5,4.35,92.0343101836753));
#62297=CARTESIAN_POINT('',(4.5,4.35,59.4601776313845));
#62298=CARTESIAN_POINT('',(4.42952305344105,4.42047694655895,91.9336586729259));
#62299=CARTESIAN_POINT('',(-0.48624091128816,9.33624091128816,84.9132201650821));
#62300=CARTESIAN_POINT('',(8.11767035354384,0.732329646456161,89.3511901313663));
#62301=CARTESIAN_POINT('Origin',(4.5,-4.5,59.4601776313845));
#62302=CARTESIAN_POINT('',(4.5,-4.35,92.0343101836753));
#62303=CARTESIAN_POINT('',(4.5,-4.35,59.4601776313845));
#62304=CARTESIAN_POINT('',(4.5,-2.25,92.0343101836753));
#62305=CARTESIAN_POINT('Origin',(4.42952305344106,-2.25,91.9336586729259));
#62306=CARTESIAN_POINT('',(4.42952305344105,-4.42047694655895,91.9336586729259));
#62307=CARTESIAN_POINT('',(-1.04322582364539,-9.89322582364539,84.1177632727136));
#62308=CARTESIAN_POINT('',(4.35904610688212,-4.35,91.8330071621765));
#62309=CARTESIAN_POINT('',(2.31610161862991,-2.30705551174733,88.9153800633939));
#62310=CARTESIAN_POINT('',(4.35904610688212,4.35,91.8330071621765));
#62311=CARTESIAN_POINT('',(4.35904610688212,-2.25,91.8330071621765));
#62312=CARTESIAN_POINT('',(2.50660167818446,2.49755557130189,89.187442343731));
#62313=CARTESIAN_POINT('Origin',(-1.41110917561106,4.425,89.8126557251908));
#62314=CARTESIAN_POINT('',(3.15,4.35,91.3929503674159));
#62315=CARTESIAN_POINT('',(-1.38545766486164,4.35,89.7421787786318));
#62316=CARTESIAN_POINT('',(3.15,4.35,91.3929503674159));
#62317=CARTESIAN_POINT('Origin',(4.42952305344106,-2.25,90.4557196172284));
#62318=CARTESIAN_POINT('',(4.42952305344106,-4.42047694655894,90.4557196172284));
#62319=CARTESIAN_POINT('',(4.5,-4.35,90.3550681064789));
#62320=CARTESIAN_POINT('',(10.1760790250279,1.32607902502795,82.2487871607733));
#62321=CARTESIAN_POINT('',(4.5,4.35,90.3550681064789));
#62322=CARTESIAN_POINT('',(4.5,-2.25,90.3550681064789));
#62323=CARTESIAN_POINT('',(4.42952305344105,4.42047694655895,90.4557196172284));
#62324=CARTESIAN_POINT('',(10.7330639373852,-1.88306393738517,81.4533302684048));
#62325=CARTESIAN_POINT('',(4.35904610688212,4.35,90.5563711279778));
#62326=CARTESIAN_POINT('',(4.55689475562393,4.54784864874185,90.2738139746405));
#62327=CARTESIAN_POINT('',(4.35904610688212,-4.35,90.5563711279778));
#62328=CARTESIAN_POINT('',(4.35904610688212,-2.25,90.5563711279778));
#62329=CARTESIAN_POINT('',(4.36639469606939,-4.35734858918728,90.5458762549776));
#62330=CARTESIAN_POINT('Origin',(9.48816622461717,4.425,88.6097107442106));
#62331=CARTESIAN_POINT('',(0.825359850204014,8.02464014979599,87.9320573733839));
#62332=CARTESIAN_POINT('',(3.15,4.35,90.9964279227383));
#62333=CARTESIAN_POINT('',(3.15,4.35,90.9964279227383));
#62334=CARTESIAN_POINT('',(9.5138177353666,4.35,88.6801876907695));
#62335=CARTESIAN_POINT('Origin',(4.425,4.425,59.4601776313845));
#62336=CARTESIAN_POINT('',(4.5,4.35,90.1493545915215));
#62337=CARTESIAN_POINT('',(4.5,4.35,59.4601776313845));
#62338=CARTESIAN_POINT('',(4.42952305344106,4.42047694655894,90.048703080772));
#62339=CARTESIAN_POINT('',(-0.153040707379776,9.00304070737977,83.5041237799868));
#62340=CARTESIAN_POINT('',(7.89798700745046,0.952012992549535,87.6200584741661));
#62341=CARTESIAN_POINT('Origin',(4.5,-4.5,59.4601776313845));
#62342=CARTESIAN_POINT('',(4.5,-4.35,90.1493545915215));
#62343=CARTESIAN_POINT('',(4.5,-4.35,59.4601776313845));
#62344=CARTESIAN_POINT('',(4.5,-2.25,90.1493545915215));
#62345=CARTESIAN_POINT('Origin',(4.42952305344106,-2.25,90.048703080772));
#62346=CARTESIAN_POINT('',(4.42952305344105,-4.42047694655895,90.048703080772));
#62347=CARTESIAN_POINT('',(-0.71002561973706,-9.56002561973706,82.7086668876183));
#62348=CARTESIAN_POINT('',(4.35904610688212,-4.35,89.9480515700226));
#62349=CARTESIAN_POINT('',(2.37308220937808,-2.36403610249577,87.1118011883403));
#62350=CARTESIAN_POINT('',(4.35904610688211,4.35,89.9480515700226));
#62351=CARTESIAN_POINT('',(4.35904610688211,-2.25,89.9480515700226));
#62352=CARTESIAN_POINT('',(2.5635822689327,2.55453616205042,87.3838634686775));
#62353=CARTESIAN_POINT('Origin',(-1.1082026507496,4.425,88.0379490918515));
#62354=CARTESIAN_POINT('',(3.15,4.35,89.5079947752621));
#62355=CARTESIAN_POINT('',(-1.08255114000017,4.35,87.9674721452925));
#62356=CARTESIAN_POINT('',(3.15,4.35,89.5079947752621));
#62357=CARTESIAN_POINT('Origin',(4.42952305344106,-2.25,88.5707640250745));
#62358=CARTESIAN_POINT('',(4.42952305344105,-4.42047694655895,88.5707640250745));
#62359=CARTESIAN_POINT('',(4.5,-4.35,88.4701125143251));
#62360=CARTESIAN_POINT('',(9.84287882111967,0.992878821119667,80.839690775678));
#62361=CARTESIAN_POINT('',(4.5,4.35,88.4701125143251));
#62362=CARTESIAN_POINT('',(4.5,-2.25,88.4701125143251));
#62363=CARTESIAN_POINT('',(4.42952305344105,4.42047694655895,88.5707640250745));
#62364=CARTESIAN_POINT('',(10.399863733477,-1.54986373347695,80.0442338833095));
#62365=CARTESIAN_POINT('',(4.35904610688211,4.35,88.6714155358239));
#62366=CARTESIAN_POINT('',(4.49991416487561,4.49086805799351,88.4702350995869));
#62367=CARTESIAN_POINT('',(4.35904610688211,-4.35,88.6714155358239));
#62368=CARTESIAN_POINT('',(4.35904610688211,-2.25,88.6714155358239));
#62369=CARTESIAN_POINT('',(4.30941410532098,-4.30036799843887,88.7422973799241));
#62370=CARTESIAN_POINT('Origin',(4.55,0.,88.6019140026118));
#62371=CARTESIAN_POINT('',(3.15,4.35,89.1114723305844));
#62372=CARTESIAN_POINT('',(9.21091121050513,4.35,86.9054810574302));
#62373=CARTESIAN_POINT('',(3.15,-4.35,89.1114723305844));
#62374=CARTESIAN_POINT('',(3.15,0.,89.1114723305844));
#62375=CARTESIAN_POINT('',(5.23731121348743,-4.35,88.351753179225));
#62376=CARTESIAN_POINT('Origin',(9.18525969975571,4.425,86.8350041108713));
#62377=CARTESIAN_POINT('',(1.04504319629739,7.80495680370261,86.2009257161837));
#62378=CARTESIAN_POINT('',(3.15,4.35,89.1114723305844));
#62379=CARTESIAN_POINT('Origin',(4.425,4.425,59.4601776313845));
#62380=CARTESIAN_POINT('',(4.5,4.35,88.2643989993676));
#62381=CARTESIAN_POINT('',(4.5,4.35,59.4601776313845));
#62382=CARTESIAN_POINT('',(4.42952305344106,4.42047694655894,88.1637474886182));
#62383=CARTESIAN_POINT('',(0.180159496528611,8.66984050347139,82.0950273948914));
#62384=CARTESIAN_POINT('',(7.67830366135663,1.17169633864337,85.8889268169666));
#62385=CARTESIAN_POINT('Origin',(4.42952305344105,-2.25,88.1637474886182));
#62386=CARTESIAN_POINT('',(4.5,-4.35,88.2643989993676));
#62387=CARTESIAN_POINT('',(4.5,-2.25,88.2643989993676));
#62388=CARTESIAN_POINT('',(4.42952305344106,-4.42047694655894,88.1637474886182));
#62389=CARTESIAN_POINT('',(-0.37682541582873,-9.22682541582873,81.2995705025229));
#62390=CARTESIAN_POINT('',(4.35904610688211,-4.35,88.0630959778687));
#62391=CARTESIAN_POINT('',(2.43006280012634,-2.42101669324411,85.3082223132868));
#62392=CARTESIAN_POINT('',(4.35904610688211,4.35,88.0630959778687));
#62393=CARTESIAN_POINT('',(4.35904610688211,-2.25,88.0630959778687));
#62394=CARTESIAN_POINT('',(2.62056285968098,2.61151675279877,85.580284593624));
#62395=CARTESIAN_POINT('Origin',(3.15,0.,87.6230391831082));
#62396=CARTESIAN_POINT('',(3.15,-4.35,87.6230391831082));
#62397=CARTESIAN_POINT('',(-4.75324461215641,-4.35,84.7464933901585));
#62398=CARTESIAN_POINT('',(3.15,4.35,87.6230391831082));
#62399=CARTESIAN_POINT('',(3.15,0.,87.6230391831082));
#62400=CARTESIAN_POINT('',(-0.779644615138703,4.35,86.1927655119533));
#62401=CARTESIAN_POINT('Origin',(-4.77889612290583,-4.425,84.8169703367175));
#62402=CARTESIAN_POINT('',(4.35,-4.5,88.219430130099));
#62403=CARTESIAN_POINT('',(7.08381293021095,-1.76618706978904,86.3051937083105));
#62404=CARTESIAN_POINT('',(3.,-4.5,87.7280703138396));
#62405=CARTESIAN_POINT('',(-4.80454763365525,-4.5,84.8874472832764));
#62406=CARTESIAN_POINT('',(3.,-4.5,87.7280703138396));
#62407=CARTESIAN_POINT('Origin',(4.425,-4.425,59.4601776313845));
#62408=CARTESIAN_POINT('',(4.35,-4.5,88.5150813835936));
#62409=CARTESIAN_POINT('',(0.450552465151825,-8.39944753484817,85.7846588248398));
#62410=CARTESIAN_POINT('',(4.35,-4.5,59.4601776313845));
#62411=CARTESIAN_POINT('',(4.5,-4.35,59.4601776313845));
#62412=CARTESIAN_POINT('Origin',(4.42952305344106,-2.25,86.6858084329206));
#62413=CARTESIAN_POINT('',(4.42952305344105,-4.42047694655895,86.6858084329206));
#62414=CARTESIAN_POINT('',(4.5,-4.35,86.5851569221712));
#62415=CARTESIAN_POINT('',(9.50967861721136,0.659678617211358,79.4305943905819));
#62416=CARTESIAN_POINT('',(4.5,4.35,86.5851569221712));
#62417=CARTESIAN_POINT('',(4.5,-2.25,86.5851569221712));
#62418=CARTESIAN_POINT('',(4.42952305344105,4.42047694655895,86.6858084329206));
#62419=CARTESIAN_POINT('',(10.0666635295686,-1.21666352956864,78.6351374982134));
#62420=CARTESIAN_POINT('',(4.35904610688211,4.35,86.78645994367));
#62421=CARTESIAN_POINT('',(4.44293357412718,4.43388746724507,86.6666562245334));
#62422=CARTESIAN_POINT('',(4.35904610688212,-4.35,86.78645994367));
#62423=CARTESIAN_POINT('',(4.35904610688211,-2.25,86.78645994367));
#62424=CARTESIAN_POINT('',(4.25243351457254,-4.24338740769039,86.9387185048706));
#62425=CARTESIAN_POINT('Origin',(8.88235317489424,4.425,85.060297477532));
#62426=CARTESIAN_POINT('',(1.26472654239079,7.5852734576092,84.4697940589836));
#62427=CARTESIAN_POINT('',(3.15,4.35,87.2265167384306));
#62428=CARTESIAN_POINT('',(3.15,4.35,87.2265167384306));
#62429=CARTESIAN_POINT('',(8.90800468564366,4.35,85.1307744240909));
#62430=CARTESIAN_POINT('Origin',(4.425,4.425,59.4601776313845));
#62431=CARTESIAN_POINT('',(4.5,4.35,86.3794434072137));
#62432=CARTESIAN_POINT('',(4.5,4.35,59.4601776313845));
#62433=CARTESIAN_POINT('',(4.42952305344105,4.42047694655895,86.2787918964643));
#62434=CARTESIAN_POINT('',(0.513359700436765,8.33664029956323,80.6859310097939));
#62435=CARTESIAN_POINT('',(7.45862031526367,1.39137968473633,84.1577951597658));
#62436=CARTESIAN_POINT('Origin',(4.5,-4.5,59.4601776313845));
#62437=CARTESIAN_POINT('',(4.5,-4.35,86.3794434072137));
#62438=CARTESIAN_POINT('',(4.5,-4.35,59.4601776313845));
#62439=CARTESIAN_POINT('',(4.5,-2.25,86.3794434072137));
#62440=CARTESIAN_POINT('Origin',(4.42952305344106,-2.25,86.2787918964643));
#62441=CARTESIAN_POINT('',(4.42952305344106,-4.42047694655894,86.2787918964643));
#62442=CARTESIAN_POINT('',(-0.0436252119204612,-8.89362521192046,79.8904741174253));
#62443=CARTESIAN_POINT('',(4.35904610688211,-4.35,86.1781403857149));
#62444=CARTESIAN_POINT('',(2.48704339087517,-2.47799728399261,83.5046434382333));
#62445=CARTESIAN_POINT('',(4.35904610688212,4.35,86.1781403857148));
#62446=CARTESIAN_POINT('',(4.35904610688212,-2.25,86.1781403857148));
#62447=CARTESIAN_POINT('',(2.67754345042971,2.6684973435472,83.7767057185704));
#62448=CARTESIAN_POINT('Origin',(-0.502389601026665,4.425,84.4885358251729));
#62449=CARTESIAN_POINT('',(3.15,4.35,85.7380835909543));
#62450=CARTESIAN_POINT('',(-0.476738090277241,4.35,84.4180588786139));
#62451=CARTESIAN_POINT('',(3.15,4.35,85.7380835909543));
#62452=CARTESIAN_POINT('Origin',(4.42952305344106,-2.25,84.8008528407667));
#62453=CARTESIAN_POINT('',(4.42952305344105,-4.42047694655895,84.8008528407668));
#62454=CARTESIAN_POINT('',(4.5,-4.35,84.7002013300173));
#62455=CARTESIAN_POINT('',(9.17647841330305,0.326478413303049,78.0214980054857));
#62456=CARTESIAN_POINT('',(4.5,4.35,84.7002013300173));
#62457=CARTESIAN_POINT('',(4.5,-2.25,84.7002013300173));
#62458=CARTESIAN_POINT('',(4.42952305344105,4.42047694655895,84.8008528407668));
#62459=CARTESIAN_POINT('',(9.73346332566033,-0.883463325660333,77.2260411131172));
#62460=CARTESIAN_POINT('',(4.35904610688211,4.35,84.9015043515162));
#62461=CARTESIAN_POINT('',(4.38595298337875,4.37690687649664,84.8630773494798));
#62462=CARTESIAN_POINT('',(4.35904610688211,-4.35,84.9015043515162));
#62463=CARTESIAN_POINT('',(4.35904610688211,-2.25,84.9015043515162));
#62464=CARTESIAN_POINT('',(4.19545292382413,-4.186406816942,85.135139629817));
#62465=CARTESIAN_POINT('Origin',(8.57944665003277,4.425,83.2855908441927));
#62466=CARTESIAN_POINT('',(1.48440988848418,7.36559011151582,82.7386624017834));
#62467=CARTESIAN_POINT('',(3.15,4.35,85.3415611462767));
#62468=CARTESIAN_POINT('',(3.15,4.35,85.3415611462767));
#62469=CARTESIAN_POINT('',(8.60509816078219,4.35,83.3560677907517));
#62470=CARTESIAN_POINT('Origin',(4.425,4.425,59.4601776313845));
#62471=CARTESIAN_POINT('',(4.5,4.35,84.4944878150598));
#62472=CARTESIAN_POINT('',(4.5,4.35,59.4601776313845));
#62473=CARTESIAN_POINT('',(4.42952305344106,4.42047694655894,84.3938363043104));
#62474=CARTESIAN_POINT('',(0.846559904345152,8.00344009565485,79.2768346246984));
#62475=CARTESIAN_POINT('',(7.23893696917029,1.61106303082971,82.4266635025656));
#62476=CARTESIAN_POINT('Origin',(4.5,-4.5,59.4601776313845));
#62477=CARTESIAN_POINT('',(4.5,-4.35,84.4944878150598));
#62478=CARTESIAN_POINT('',(4.5,-4.35,59.4601776313845));
#62479=CARTESIAN_POINT('',(4.5,-2.25,84.4944878150598));
#62480=CARTESIAN_POINT('Origin',(4.42952305344106,-2.25,84.3938363043104));
#62481=CARTESIAN_POINT('',(4.42952305344105,-4.42047694655895,84.3938363043104));
#62482=CARTESIAN_POINT('',(0.289574991987868,-8.56042500801213,78.4813777323299));
#62483=CARTESIAN_POINT('',(4.35904610688212,-4.35,84.293184793561));
#62484=CARTESIAN_POINT('',(2.54402398162343,-2.53497787474096,81.7010645631798));
#62485=CARTESIAN_POINT('',(4.35904610688211,4.35,84.293184793561));
#62486=CARTESIAN_POINT('',(4.35904610688211,-2.25,84.293184793561));
#62487=CARTESIAN_POINT('',(2.73452404117798,2.72547793429572,81.9731268435169));
#62488=CARTESIAN_POINT('Origin',(-0.199483076165196,4.425,82.7138291918336));
#62489=CARTESIAN_POINT('',(3.15,4.35,83.8531279988004));
#62490=CARTESIAN_POINT('',(-0.173831565415771,4.35,82.6433522452747));
#62491=CARTESIAN_POINT('',(3.15,4.35,83.8531279988004));
#62492=CARTESIAN_POINT('Origin',(4.42952305344106,-2.25,82.9158972486129));
#62493=CARTESIAN_POINT('',(4.42952305344105,-4.42047694655895,82.9158972486129));
#62494=CARTESIAN_POINT('',(8.84327820939474,-0.0067217906052579,76.6124016203896));
#62495=CARTESIAN_POINT('',(4.35904610688211,4.35,83.0165487593623));
#62496=CARTESIAN_POINT('',(4.32897239263033,4.31992628574822,83.0594984744263));
#62497=CARTESIAN_POINT('',(4.35904610688211,-4.35,83.0165487593623));
#62498=CARTESIAN_POINT('',(4.35904610688211,-2.25,83.0165487593623));
#62499=CARTESIAN_POINT('',(4.1384723330757,-4.12942622619357,83.3315607547635));
#62500=CARTESIAN_POINT('Origin',(4.30294012815361,-4.425,82.9571563326482));
#62501=CARTESIAN_POINT('',(3.15,-4.35,83.4566055541228));
#62502=CARTESIAN_POINT('',(4.32859163890303,-4.35,83.0276332792071));
#62503=CARTESIAN_POINT('',(3.,-4.5,83.3515744233914));
#62504=CARTESIAN_POINT('',(3.,-4.5,83.3515744233914));
#62505=CARTESIAN_POINT('',(4.35,-4.5,82.860214607132));
#62506=CARTESIAN_POINT('',(4.27728861740418,-4.5,82.8866793860892));
#62507=CARTESIAN_POINT('',(1.10960250343199,-7.740397496568,80.5912638532393));
#62508=CARTESIAN_POINT('Origin',(4.55,0.,82.9470472261501));
#62509=CARTESIAN_POINT('',(3.15,4.35,83.4566055541228));
#62510=CARTESIAN_POINT('',(8.30219163592073,4.35,81.5813611574124));
#62511=CARTESIAN_POINT('',(3.15,0.,83.4566055541228));
#62512=CARTESIAN_POINT('Origin',(8.27654012517131,4.425,81.5108842108534));
#62513=CARTESIAN_POINT('',(3.15,4.35,83.4566055541228));
#62514=CARTESIAN_POINT('Origin',(3.075,4.425,71.4583915927537));
#62515=CARTESIAN_POINT('',(3.15,4.35,71.4583915927537));
#62516=CARTESIAN_POINT('Origin',(3.15,0.,83.4566055541228));
#62517=CARTESIAN_POINT('',(3.15,-4.35,83.8531279988004));
#62518=CARTESIAN_POINT('',(3.15,0.,83.8531279988004));
#62519=CARTESIAN_POINT('',(3.15,-4.35,71.4583915927537));
#62520=CARTESIAN_POINT('Origin',(3.15,0.,83.8531279988004));
#62521=CARTESIAN_POINT('',(-4.14743156243347,-4.35,81.1970801234799));
#62522=CARTESIAN_POINT('Origin',(3.075,4.425,72.4008693888306));
#62523=CARTESIAN_POINT('',(3.15,4.35,72.4008693888306));
#62524=CARTESIAN_POINT('Origin',(4.55,0.,84.832002818304));
#62525=CARTESIAN_POINT('',(3.15,-4.35,85.3415611462767));
#62526=CARTESIAN_POINT('',(3.15,0.,85.3415611462767));
#62527=CARTESIAN_POINT('',(4.6314981637645,-4.35,84.8023399125464));
#62528=CARTESIAN_POINT('Origin',(3.15,0.,85.3415611462767));
#62529=CARTESIAN_POINT('',(3.15,-4.35,85.7380835909543));
#62530=CARTESIAN_POINT('',(3.15,0.,85.7380835909543));
#62531=CARTESIAN_POINT('',(3.15,-4.35,72.4008693888306));
#62532=CARTESIAN_POINT('Origin',(3.15,0.,85.7380835909543));
#62533=CARTESIAN_POINT('',(-4.45033808729494,-4.35,82.9717867568192));
#62534=CARTESIAN_POINT('Origin',(-0.805296125888126,4.425,86.2632424585122));
#62535=CARTESIAN_POINT('',(3.15,4.35,87.6230391831082));
#62536=CARTESIAN_POINT('Origin',(3.075,4.425,73.3433471849075));
#62537=CARTESIAN_POINT('',(3.15,4.35,73.3433471849075));
#62538=CARTESIAN_POINT('Origin',(4.55,0.,86.7169584104579));
#62539=CARTESIAN_POINT('',(3.15,-4.35,87.2265167384306));
#62540=CARTESIAN_POINT('',(3.15,0.,87.2265167384306));
#62541=CARTESIAN_POINT('',(4.93440468862596,-4.35,86.5770465458857));
#62542=CARTESIAN_POINT('Origin',(3.15,0.,87.2265167384306));
#62543=CARTESIAN_POINT('',(3.15,-4.35,73.3433471849075));
#62544=CARTESIAN_POINT('Origin',(3.075,4.425,74.2858249809845));
#62545=CARTESIAN_POINT('',(3.15,4.35,74.2858249809845));
#62546=CARTESIAN_POINT('Origin',(3.15,0.,89.1114723305844));
#62547=CARTESIAN_POINT('',(3.15,-4.35,89.5079947752621));
#62548=CARTESIAN_POINT('',(3.15,0.,89.5079947752621));
#62549=CARTESIAN_POINT('',(3.15,-4.35,74.2858249809845));
#62550=CARTESIAN_POINT('Origin',(3.15,0.,89.5079947752621));
#62551=CARTESIAN_POINT('',(-5.05615113701787,-4.35,86.5212000234978));
#62552=CARTESIAN_POINT('Origin',(3.075,4.425,75.2283027770614));
#62553=CARTESIAN_POINT('',(3.15,4.35,75.2283027770614));
#62554=CARTESIAN_POINT('Origin',(4.55,0.,90.4868695947656));
#62555=CARTESIAN_POINT('',(3.15,-4.35,90.9964279227383));
#62556=CARTESIAN_POINT('',(3.15,0.,90.9964279227383));
#62557=CARTESIAN_POINT('',(5.5402177383489,-4.35,90.1264598125642));
#62558=CARTESIAN_POINT('Origin',(3.15,0.,90.9964279227383));
#62559=CARTESIAN_POINT('',(3.15,-4.35,91.3929503674159));
#62560=CARTESIAN_POINT('',(3.15,0.,91.3929503674159));
#62561=CARTESIAN_POINT('',(3.15,-4.35,75.2283027770614));
#62562=CARTESIAN_POINT('Origin',(3.15,0.,91.3929503674159));
#62563=CARTESIAN_POINT('',(-5.35905766187934,-4.35,88.2959066568371));
#62564=CARTESIAN_POINT('Origin',(3.075,4.425,76.1707805731383));
#62565=CARTESIAN_POINT('',(3.15,4.35,76.1707805731383));
#62566=CARTESIAN_POINT('Origin',(4.55,0.,92.3718251869195));
#62567=CARTESIAN_POINT('',(3.15,-4.35,92.8813835148922));
#62568=CARTESIAN_POINT('',(3.15,0.,92.8813835148922));
#62569=CARTESIAN_POINT('',(5.84312426321037,-4.35,91.9011664459035));
#62570=CARTESIAN_POINT('Origin',(3.15,0.,92.8813835148922));
#62571=CARTESIAN_POINT('',(3.15,-4.35,93.2779059595698));
#62572=CARTESIAN_POINT('',(3.15,0.,93.2779059595698));
#62573=CARTESIAN_POINT('',(3.15,-4.35,76.1707805731383));
#62574=CARTESIAN_POINT('Origin',(3.15,0.,93.2779059595698));
#62575=CARTESIAN_POINT('',(-5.6619641867408,-4.35,90.0706132901764));
#62576=CARTESIAN_POINT('Origin',(3.075,4.425,77.1132583692153));
#62577=CARTESIAN_POINT('',(3.15,4.35,77.1132583692153));
#62578=CARTESIAN_POINT('Origin',(4.55,0.,94.2567807790734));
#62579=CARTESIAN_POINT('',(3.15,-4.35,94.7663391070461));
#62580=CARTESIAN_POINT('',(3.15,0.,94.7663391070461));
#62581=CARTESIAN_POINT('',(6.14603078807183,-4.35,93.6758730792428));
#62582=CARTESIAN_POINT('Origin',(3.15,0.,94.7663391070461));
#62583=CARTESIAN_POINT('',(3.15,-4.35,77.1132583692153));
#62584=CARTESIAN_POINT('Origin',(3.075,4.425,78.0557361652922));
#62585=CARTESIAN_POINT('',(3.15,4.35,78.0557361652922));
#62586=CARTESIAN_POINT('Origin',(3.15,0.,96.6512946992));
#62587=CARTESIAN_POINT('',(3.15,-4.35,97.0478171438776));
#62588=CARTESIAN_POINT('',(3.15,0.,97.0478171438776));
#62589=CARTESIAN_POINT('',(3.15,-4.35,78.0557361652922));
#62590=CARTESIAN_POINT('Origin',(3.15,0.,97.0478171438776));
#62591=CARTESIAN_POINT('',(-6.26777723646374,-4.35,93.620026556855));
#62592=CARTESIAN_POINT('Origin',(3.075,4.425,78.9982139613691));
#62593=CARTESIAN_POINT('',(3.15,4.35,78.9982139613691));
#62594=CARTESIAN_POINT('Origin',(4.55,0.,98.0266919633811));
#62595=CARTESIAN_POINT('',(3.15,-4.35,98.5362502913538));
#62596=CARTESIAN_POINT('',(3.15,0.,98.5362502913538));
#62597=CARTESIAN_POINT('',(6.75184383779476,-4.35,97.2252863459214));
#62598=CARTESIAN_POINT('Origin',(3.15,0.,98.5362502913538));
#62599=CARTESIAN_POINT('',(3.15,-4.35,98.9327727360315));
#62600=CARTESIAN_POINT('',(3.15,0.,98.9327727360315));
#62601=CARTESIAN_POINT('',(3.15,-4.35,78.9982139613691));
#62602=CARTESIAN_POINT('Origin',(3.15,0.,98.9327727360315));
#62603=CARTESIAN_POINT('',(-6.5706837613252,-4.35,95.3947331901942));
#62604=CARTESIAN_POINT('Origin',(4.42952305344106,-2.25,111.190231130921));
#62605=CARTESIAN_POINT('',(4.42952305344105,-4.42047694655895,111.190231130921));
#62606=CARTESIAN_POINT('',(4.5,-4.35,111.089579620172));
#62607=CARTESIAN_POINT('',(13.8412812680194,4.99128126801937,97.7488473968316));
#62608=CARTESIAN_POINT('',(4.5,4.35,111.089579620172));
#62609=CARTESIAN_POINT('',(4.5,-2.25,111.089579620172));
#62610=CARTESIAN_POINT('',(4.42952305344104,4.42047694655895,111.190231130921));
#62611=CARTESIAN_POINT('',(14.3982661803767,-5.54826618037665,96.9533905044631));
#62612=CARTESIAN_POINT('',(4.35904610688211,4.35,111.29088264167));
#62613=CARTESIAN_POINT('',(5.1836812538568,5.17463514697474,110.113181600229));
#62614=CARTESIAN_POINT('',(4.35904610688211,-4.35,111.29088264167));
#62615=CARTESIAN_POINT('',(4.35904610688211,-2.25,111.29088264167));
#62616=CARTESIAN_POINT('',(4.99318119430216,-4.98413508742011,110.385243880566));
#62617=CARTESIAN_POINT('Origin',(12.8201379980935,4.425,108.131483710943));
#62618=CARTESIAN_POINT('',(-1.59115695682325,10.4411569568232,106.974505602586));
#62619=CARTESIAN_POINT('',(3.15,4.35,111.730939436431));
#62620=CARTESIAN_POINT('',(3.15,4.35,111.730939436431));
#62621=CARTESIAN_POINT('',(12.8457895088429,4.35,108.201960657502));
#62622=CARTESIAN_POINT('Origin',(4.425,4.425,59.4601776313845));
#62623=CARTESIAN_POINT('',(4.5,4.35,110.883866105214));
#62624=CARTESIAN_POINT('',(4.5,4.35,59.4601776313845));
#62625=CARTESIAN_POINT('',(4.42952305344106,4.42047694655894,110.783214594465));
#62626=CARTESIAN_POINT('',(-3.81824295037126,12.6682429503713,99.0041840160429));
#62627=CARTESIAN_POINT('',(10.3145038144786,-1.46450381447857,106.662506703367));
#62628=CARTESIAN_POINT('Origin',(4.5,-4.5,59.4601776313845));
#62629=CARTESIAN_POINT('',(4.5,-4.35,110.883866105214));
#62630=CARTESIAN_POINT('',(4.5,-4.35,59.4601776313845));
#62631=CARTESIAN_POINT('',(4.5,-2.25,110.883866105214));
#62632=CARTESIAN_POINT('Origin',(4.42952305344106,-2.25,110.783214594465));
#62633=CARTESIAN_POINT('',(4.42952305344105,-4.42047694655896,110.783214594465));
#62634=CARTESIAN_POINT('',(-4.37522786272848,-13.2252278627285,98.2087271236743));
#62635=CARTESIAN_POINT('',(4.35904610688212,-4.35,110.682563083715));
#62636=CARTESIAN_POINT('',(1.74629571114559,-1.73724960426314,106.951168813929));
#62637=CARTESIAN_POINT('',(4.35904610688212,4.35,110.682563083715));
#62638=CARTESIAN_POINT('',(4.35904610688212,-2.25,110.682563083715));
#62639=CARTESIAN_POINT('',(1.9367957707002,1.92774966381778,107.223231094266));
#62640=CARTESIAN_POINT('Origin',(-4.44017442422591,4.425,107.559722058583));
#62641=CARTESIAN_POINT('',(3.15,4.35,110.242506288955));
#62642=CARTESIAN_POINT('',(-4.41452291347648,4.35,107.489245112025));
#62643=CARTESIAN_POINT('',(3.15,4.35,110.242506288955));
#62644=CARTESIAN_POINT('Origin',(4.42952305344106,-2.25,109.305275538767));
#62645=CARTESIAN_POINT('',(4.42952305344107,-4.42047694655893,109.305275538767));
#62646=CARTESIAN_POINT('',(4.5,-4.35,109.204624028018));
#62647=CARTESIAN_POINT('',(13.5080810641111,4.65808106411106,96.3397510117354));
#62648=CARTESIAN_POINT('',(4.5,4.35,109.204624028018));
#62649=CARTESIAN_POINT('',(4.5,-2.25,109.204624028018));
#62650=CARTESIAN_POINT('',(4.42952305344105,4.42047694655895,109.305275538767));
#62651=CARTESIAN_POINT('',(14.0650659764683,-5.21506597646833,95.5442941193668));
#62652=CARTESIAN_POINT('',(4.35904610688212,4.35,109.405927049517));
#62653=CARTESIAN_POINT('',(5.12670066310835,5.11765455622629,108.309602725176));
#62654=CARTESIAN_POINT('',(4.35904610688212,-4.35,109.405927049517));
#62655=CARTESIAN_POINT('',(4.35904610688212,-2.25,109.405927049517));
#62656=CARTESIAN_POINT('',(4.93620060355377,-4.92715449667165,108.581665005513));
#62657=CARTESIAN_POINT('Origin',(12.517231473232,4.425,106.356777077603));
#62658=CARTESIAN_POINT('',(-1.37147361072985,10.2214736107299,105.243373945386));
#62659=CARTESIAN_POINT('',(3.15,4.35,109.845983844277));
#62660=CARTESIAN_POINT('',(3.15,4.35,109.845983844277));
#62661=CARTESIAN_POINT('',(12.5428829839814,4.35,106.427254024162));
#62662=CARTESIAN_POINT('Origin',(4.425,4.425,59.4601776313845));
#62663=CARTESIAN_POINT('',(4.5,4.35,108.99891051306));
#62664=CARTESIAN_POINT('',(4.5,4.35,59.4601776313845));
#62665=CARTESIAN_POINT('',(4.42952305344105,4.42047694655895,108.898259002311));
#62666=CARTESIAN_POINT('',(-3.48504274646279,12.3350427464628,97.5950876309494));
#62667=CARTESIAN_POINT('',(10.0948204683843,-1.24482046838432,104.931375046168));
#62668=CARTESIAN_POINT('Origin',(4.5,-4.5,59.4601776313845));
#62669=CARTESIAN_POINT('',(4.5,-4.35,108.99891051306));
#62670=CARTESIAN_POINT('',(4.5,-4.35,59.4601776313845));
#62671=CARTESIAN_POINT('',(4.5,-2.25,108.99891051306));
#62672=CARTESIAN_POINT('Origin',(4.42952305344106,-2.25,108.898259002311));
#62673=CARTESIAN_POINT('',(4.42952305344105,-4.42047694655895,108.898259002311));
#62674=CARTESIAN_POINT('',(-4.04202765882012,-12.8920276588201,96.7996307385808));
#62675=CARTESIAN_POINT('',(4.35904610688211,-4.35,108.797607491561));
#62676=CARTESIAN_POINT('',(1.80327630189361,-1.79423019501132,105.147589938876));
#62677=CARTESIAN_POINT('',(4.35904610688211,4.35,108.797607491561));
#62678=CARTESIAN_POINT('',(4.35904610688211,-2.25,108.797607491561));
#62679=CARTESIAN_POINT('',(1.9937763614482,1.98473025456618,105.419652219213));
#62680=CARTESIAN_POINT('Origin',(-4.13726789936425,4.425,105.785015425244));
#62681=CARTESIAN_POINT('',(3.15,4.35,108.357550696801));
#62682=CARTESIAN_POINT('',(-4.11161638861483,4.35,105.714538478685));
#62683=CARTESIAN_POINT('',(3.15,4.35,108.357550696801));
#62684=CARTESIAN_POINT('Origin',(4.42952305344106,-2.25,107.420319946613));
#62685=CARTESIAN_POINT('',(4.42952305344105,-4.42047694655894,107.420319946613));
#62686=CARTESIAN_POINT('',(4.5,-4.35,107.319668435864));
#62687=CARTESIAN_POINT('',(13.1748808602028,4.32488086020279,94.9306546266404));
#62688=CARTESIAN_POINT('',(4.5,4.35,107.319668435864));
#62689=CARTESIAN_POINT('',(4.5,-2.25,107.319668435864));
#62690=CARTESIAN_POINT('',(4.42952305344105,4.42047694655895,107.420319946613));
#62691=CARTESIAN_POINT('',(13.7318657725601,-4.88186577256012,94.1351977342719));
#62692=CARTESIAN_POINT('',(4.35904610688211,4.35,107.520971457363));
#62693=CARTESIAN_POINT('',(5.06972007235996,5.06067396547791,106.506023850122));
#62694=CARTESIAN_POINT('',(4.35904610688211,-4.35,107.520971457363));
#62695=CARTESIAN_POINT('',(4.35904610688211,-2.25,107.520971457363));
#62696=CARTESIAN_POINT('',(4.87922001280538,-4.87017390592325,106.778086130459));
#62697=CARTESIAN_POINT('Origin',(12.2143249483705,4.425,104.582070444264));
#62698=CARTESIAN_POINT('',(-1.1517902646357,10.0017902646357,103.512242288186));
#62699=CARTESIAN_POINT('',(3.15,4.35,107.961028252123));
#62700=CARTESIAN_POINT('',(3.15,4.35,107.961028252123));
#62701=CARTESIAN_POINT('',(12.23997645912,4.35,104.652547390823));
#62702=CARTESIAN_POINT('Origin',(4.425,4.425,59.4601776313845));
#62703=CARTESIAN_POINT('',(4.5,4.35,107.113954920906));
#62704=CARTESIAN_POINT('',(4.5,4.35,59.4601776313845));
#62705=CARTESIAN_POINT('',(4.42952305344105,4.42047694655895,107.013303410157));
#62706=CARTESIAN_POINT('',(-3.15184254255455,12.0018425425546,96.1859912458521));
#62707=CARTESIAN_POINT('',(9.87513712229095,-1.02513712229095,103.200243388968));
#62708=CARTESIAN_POINT('Origin',(4.5,-4.5,59.4601776313845));
#62709=CARTESIAN_POINT('',(4.5,-4.35,107.113954920906));
#62710=CARTESIAN_POINT('',(4.5,-4.35,59.4601776313845));
#62711=CARTESIAN_POINT('',(4.5,-2.25,107.113954920906));
#62712=CARTESIAN_POINT('Origin',(4.42952305344106,-2.25,107.013303410157));
#62713=CARTESIAN_POINT('',(4.42952305344105,-4.42047694655895,107.013303410157));
#62714=CARTESIAN_POINT('',(-3.70882745491184,-12.5588274549118,95.3905343534835));
#62715=CARTESIAN_POINT('',(4.35904610688212,-4.35,106.912651899407));
#62716=CARTESIAN_POINT('',(1.86025689264218,-1.85121078575986,103.344011063822));
#62717=CARTESIAN_POINT('',(4.35904610688211,4.35,106.912651899407));
#62718=CARTESIAN_POINT('',(4.35904610688211,-2.25,106.912651899407));
#62719=CARTESIAN_POINT('',(2.05075695219681,2.04171084531453,103.616073344159));
#62720=CARTESIAN_POINT('Origin',(-3.83436137450296,4.425,104.010308791905));
#62721=CARTESIAN_POINT('',(3.15,4.35,106.472595104647));
#62722=CARTESIAN_POINT('',(-3.80870986375353,4.35,103.939831845346));
#62723=CARTESIAN_POINT('',(3.15,4.35,106.472595104647));
#62724=CARTESIAN_POINT('Origin',(4.42952305344106,-2.25,105.535364354459));
#62725=CARTESIAN_POINT('',(4.42952305344105,-4.42047694655895,105.535364354459));
#62726=CARTESIAN_POINT('',(4.5,-4.35,105.43471284371));
#62727=CARTESIAN_POINT('',(12.8416806562944,3.99168065629444,93.5215582415431));
#62728=CARTESIAN_POINT('',(4.5,4.35,105.43471284371));
#62729=CARTESIAN_POINT('',(4.5,-2.25,105.43471284371));
#62730=CARTESIAN_POINT('',(4.42952305344106,4.42047694655894,105.535364354459));
#62731=CARTESIAN_POINT('',(13.3986655686517,-4.54866556865172,92.7261013491746));
#62732=CARTESIAN_POINT('',(4.35904610688211,4.35,105.636015865209));
#62733=CARTESIAN_POINT('',(5.01273948161149,5.00369337472944,104.702444975068));
#62734=CARTESIAN_POINT('',(4.35904610688212,-4.35,105.636015865209));
#62735=CARTESIAN_POINT('',(4.35904610688212,-2.25,105.636015865209));
#62736=CARTESIAN_POINT('',(4.82223942205686,-4.81319331517479,104.974507255406));
#62737=CARTESIAN_POINT('Origin',(11.9114184235091,4.425,102.807363810925));
#62738=CARTESIAN_POINT('',(-0.932106918543077,9.78210691854308,101.781110630985));
#62739=CARTESIAN_POINT('',(3.15,4.35,106.076072659969));
#62740=CARTESIAN_POINT('',(3.15,4.35,106.076072659969));
#62741=CARTESIAN_POINT('',(11.9370699342585,4.35,102.877840757484));
#62742=CARTESIAN_POINT('Origin',(4.425,4.425,59.4601776313845));
#62743=CARTESIAN_POINT('',(4.5,4.35,105.228999328752));
#62744=CARTESIAN_POINT('',(4.5,4.35,59.4601776313845));
#62745=CARTESIAN_POINT('',(4.42952305344105,4.42047694655895,105.128347818003));
#62746=CARTESIAN_POINT('',(-2.81864233864633,11.6686423386463,94.7768948607546));
#62747=CARTESIAN_POINT('',(9.65545377619829,-0.805453776198292,101.469111731766));
#62748=CARTESIAN_POINT('Origin',(4.5,-4.5,59.4601776313845));
#62749=CARTESIAN_POINT('',(4.5,-4.35,105.228999328752));
#62750=CARTESIAN_POINT('',(4.5,-4.35,59.4601776313845));
#62751=CARTESIAN_POINT('',(4.5,-2.25,105.228999328752));
#62752=CARTESIAN_POINT('Origin',(4.42952305344106,-2.25,105.128347818003));
#62753=CARTESIAN_POINT('',(4.42952305344105,-4.42047694655895,105.128347818003));
#62754=CARTESIAN_POINT('',(-3.37562725100355,-12.2256272510036,93.9814379683861));
#62755=CARTESIAN_POINT('',(4.35904610688212,-4.35,105.027696307254));
#62756=CARTESIAN_POINT('',(1.91723748339086,-1.90819137650842,101.540432188768));
#62757=CARTESIAN_POINT('',(4.35904610688212,4.35,105.027696307254));
#62758=CARTESIAN_POINT('',(4.35904610688212,-2.25,105.027696307254));
#62759=CARTESIAN_POINT('',(2.10773754294547,2.09869143606306,101.812494469106));
#62760=CARTESIAN_POINT('Origin',(-3.53145484964149,4.425,102.235602158566));
#62761=CARTESIAN_POINT('',(3.15,4.35,104.587639512493));
#62762=CARTESIAN_POINT('',(-3.50580333889206,4.35,102.165125212007));
#62763=CARTESIAN_POINT('',(3.15,4.35,104.587639512493));
#62764=CARTESIAN_POINT('Origin',(4.42952305344106,-2.25,103.650408762305));
#62765=CARTESIAN_POINT('',(4.42952305344105,-4.42047694655894,103.650408762305));
#62766=CARTESIAN_POINT('',(4.5,-4.35,103.549757251556));
#62767=CARTESIAN_POINT('',(12.5084804523861,3.65848045238613,92.1124618564469));
#62768=CARTESIAN_POINT('',(4.5,4.35,103.549757251556));
#62769=CARTESIAN_POINT('',(4.5,-2.25,103.549757251556));
#62770=CARTESIAN_POINT('',(4.42952305344106,4.42047694655894,103.650408762305));
#62771=CARTESIAN_POINT('',(13.0654653647434,-4.21546536474341,91.3170049640784));
#62772=CARTESIAN_POINT('',(4.35904610688211,4.35,103.751060273055));
#62773=CARTESIAN_POINT('',(4.95575889086306,4.94671278398101,102.898866100015));
#62774=CARTESIAN_POINT('',(4.35904610688212,-4.35,103.751060273055));
#62775=CARTESIAN_POINT('',(4.35904610688212,-2.25,103.751060273055));
#62776=CARTESIAN_POINT('',(4.76525883130843,-4.75621272442636,103.170928380352));
#62777=CARTESIAN_POINT('Origin',(11.6085118986476,4.425,101.032657177585));
#62778=CARTESIAN_POINT('',(-0.712423572449715,9.56242357244971,100.049978973785));
#62779=CARTESIAN_POINT('',(3.15,4.35,104.191117067815));
#62780=CARTESIAN_POINT('',(3.15,4.35,104.191117067815));
#62781=CARTESIAN_POINT('',(11.634163409397,4.35,101.103134124144));
#62782=CARTESIAN_POINT('Origin',(4.425,4.425,59.4601776313845));
#62783=CARTESIAN_POINT('',(4.5,4.35,103.344043736599));
#62784=CARTESIAN_POINT('',(4.5,4.35,59.4601776313845));
#62785=CARTESIAN_POINT('',(4.42952305344105,4.42047694655894,103.243392225849));
#62786=CARTESIAN_POINT('',(-2.48544213473794,11.3354421347379,93.3677984756598));
#62787=CARTESIAN_POINT('',(9.43577043010417,-0.585770430104168,99.7379800745673));
#62788=CARTESIAN_POINT('Origin',(4.5,-4.5,59.4601776313845));
#62789=CARTESIAN_POINT('',(4.5,-4.35,103.344043736599));
#62790=CARTESIAN_POINT('',(4.5,-4.35,59.4601776313845));
#62791=CARTESIAN_POINT('',(4.5,-2.25,103.344043736599));
#62792=CARTESIAN_POINT('Origin',(4.42952305344106,-2.25,103.243392225849));
#62793=CARTESIAN_POINT('',(4.42952305344105,-4.42047694655895,103.243392225849));
#62794=CARTESIAN_POINT('',(-3.04242704709522,-11.8924270470952,92.5723415832913));
#62795=CARTESIAN_POINT('',(4.35904610688211,-4.35,103.1427407151));
#62796=CARTESIAN_POINT('',(1.97421807413904,-1.96517196725673,99.7368533137148));
#62797=CARTESIAN_POINT('',(4.35904610688211,4.35,103.1427407151));
#62798=CARTESIAN_POINT('',(4.35904610688211,-2.25,103.1427407151));
#62799=CARTESIAN_POINT('',(2.16471813369367,2.15567202681139,100.008915594052));
#62800=CARTESIAN_POINT('Origin',(-3.22854832478001,4.425,100.460895525226));
#62801=CARTESIAN_POINT('',(3.15,4.35,102.702683920339));
#62802=CARTESIAN_POINT('',(-3.20289681403059,4.35,100.390418578667));
#62803=CARTESIAN_POINT('',(3.15,4.35,102.702683920339));
#62804=CARTESIAN_POINT('Origin',(4.42952305344106,-2.25,101.765453170152));
#62805=CARTESIAN_POINT('',(4.42952305344105,-4.42047694655895,101.765453170152));
#62806=CARTESIAN_POINT('',(4.5,-4.35,101.664801659402));
#62807=CARTESIAN_POINT('',(12.1752802484778,3.32528024847783,90.703365471351));
#62808=CARTESIAN_POINT('',(4.5,4.35,101.664801659402));
#62809=CARTESIAN_POINT('',(4.5,-2.25,101.664801659402));
#62810=CARTESIAN_POINT('',(4.42952305344106,4.42047694655895,101.765453170152));
#62811=CARTESIAN_POINT('',(12.7322651608351,-3.88226516083512,89.9079085789825));
#62812=CARTESIAN_POINT('',(4.35904610688211,4.35,101.866104680901));
#62813=CARTESIAN_POINT('',(4.8987783001146,4.88973219323253,101.095287224962));
#62814=CARTESIAN_POINT('',(4.35904610688211,-4.35,101.866104680901));
#62815=CARTESIAN_POINT('',(4.35904610688211,-2.25,101.866104680901));
#62816=CARTESIAN_POINT('',(4.70827824055998,-4.69923213367789,101.367349505299));
#62817=CARTESIAN_POINT('Origin',(11.305605373786,4.425,99.2579505442463));
#62818=CARTESIAN_POINT('',(-0.492740226356329,9.34274022635633,98.3188473165849));
#62819=CARTESIAN_POINT('',(3.15,4.35,102.306161475662));
#62820=CARTESIAN_POINT('',(3.15,4.35,102.306161475662));
#62821=CARTESIAN_POINT('',(11.3312568845354,4.35,99.3284274908053));
#62822=CARTESIAN_POINT('Origin',(4.425,4.425,59.4601776313845));
#62823=CARTESIAN_POINT('',(4.5,4.35,101.459088144445));
#62824=CARTESIAN_POINT('',(4.5,4.35,59.4601776313845));
#62825=CARTESIAN_POINT('',(4.42952305344105,4.42047694655894,101.358436633695));
#62826=CARTESIAN_POINT('',(-2.15224193082962,11.0022419308296,91.9587020905637));
#62827=CARTESIAN_POINT('',(9.2160870840108,-0.366087084010803,98.0068484173671));
#62828=CARTESIAN_POINT('Origin',(4.5,-4.5,59.4601776313845));
#62829=CARTESIAN_POINT('',(4.5,-4.35,101.459088144445));
#62830=CARTESIAN_POINT('',(4.5,-4.35,59.4601776313845));
#62831=CARTESIAN_POINT('',(4.5,-2.25,101.459088144445));
#62832=CARTESIAN_POINT('Origin',(4.42952305344106,-2.25,101.358436633695));
#62833=CARTESIAN_POINT('',(4.42952305344105,-4.42047694655895,101.358436633695));
#62834=CARTESIAN_POINT('',(-2.70922684318691,-11.5592268431869,91.1632451981952));
#62835=CARTESIAN_POINT('',(4.35904610688212,-4.35,101.257785122946));
#62836=CARTESIAN_POINT('',(2.03119866488751,-2.02215255800518,97.9332744386614));
#62837=CARTESIAN_POINT('',(4.35904610688211,4.35,101.257785122946));
#62838=CARTESIAN_POINT('',(4.35904610688211,-2.25,101.257785122946));
#62839=CARTESIAN_POINT('',(2.22169872444213,2.21265261755984,98.2053367189986));
#62840=CARTESIAN_POINT('Origin',(-2.92564179991839,4.425,98.6861888918872));
#62841=CARTESIAN_POINT('',(3.15,4.35,100.817728328185));
#62842=CARTESIAN_POINT('',(-2.89999028916897,4.35,98.6157119453282));
#62843=CARTESIAN_POINT('',(3.15,4.35,100.817728328185));
#62844=CARTESIAN_POINT('Origin',(4.42952305344105,-2.25,99.8804975779977));
#62845=CARTESIAN_POINT('',(4.42952305344105,-4.42047694655895,99.8804975779977));
#62846=CARTESIAN_POINT('',(11.8420800445696,2.99208004456955,89.2942690862559));
#62847=CARTESIAN_POINT('',(4.35904610688211,4.35,99.9811490887472));
#62848=CARTESIAN_POINT('',(4.8417977093661,4.83275160248406,99.2917083499081));
#62849=CARTESIAN_POINT('',(4.35904610688211,-4.35,99.9811490887472));
#62850=CARTESIAN_POINT('',(4.35904610688211,-2.25,99.9811490887472));
#62851=CARTESIAN_POINT('',(4.65129764981156,-4.64225154292948,99.5637706302452));
#62852=CARTESIAN_POINT('Origin',(7.02909885190681,-4.425,98.9295160327017));
#62853=CARTESIAN_POINT('',(3.15,-4.35,100.421205883508));
#62854=CARTESIAN_POINT('',(7.05475036265623,-4.35,98.9999929792607));
#62855=CARTESIAN_POINT('',(3.,-4.5,100.316174752776));
#62856=CARTESIAN_POINT('',(3.,-4.5,100.316174752776));
#62857=CARTESIAN_POINT('',(4.35,-4.5,99.8248149365169));
#62858=CARTESIAN_POINT('',(7.00344734115739,-4.5,98.8590390861428));
#62859=CARTESIAN_POINT('',(-0.867547611407954,-9.71754761140796,96.1714487680417));
#62860=CARTESIAN_POINT('Origin',(4.55,0.,99.911647555535));
#62861=CARTESIAN_POINT('',(3.15,4.35,100.421205883508));
#62862=CARTESIAN_POINT('',(11.0283503596739,4.35,97.5537208574659));
#62863=CARTESIAN_POINT('',(3.15,0.,100.421205883508));
#62864=CARTESIAN_POINT('Origin',(11.0026988489245,4.425,97.483243910907));
#62865=CARTESIAN_POINT('',(3.15,4.35,100.421205883508));
#62866=CARTESIAN_POINT('Origin',(3.075,4.425,79.9406917574461));
#62867=CARTESIAN_POINT('',(3.15,4.35,79.9406917574461));
#62868=CARTESIAN_POINT('Origin',(3.15,0.,100.421205883508));
#62869=CARTESIAN_POINT('',(3.15,-4.35,100.817728328185));
#62870=CARTESIAN_POINT('',(3.15,0.,100.817728328185));
#62871=CARTESIAN_POINT('',(3.15,-4.35,79.9406917574461));
#62872=CARTESIAN_POINT('Origin',(3.15,0.,100.817728328185));
#62873=CARTESIAN_POINT('',(-6.87359028618667,-4.35,97.1694398235335));
#62874=CARTESIAN_POINT('Origin',(3.075,4.425,80.883169553523));
#62875=CARTESIAN_POINT('',(3.15,4.35,80.883169553523));
#62876=CARTESIAN_POINT('Origin',(4.55,0.,101.796603147689));
#62877=CARTESIAN_POINT('',(3.15,-4.35,102.306161475662));
#62878=CARTESIAN_POINT('',(3.15,0.,102.306161475662));
#62879=CARTESIAN_POINT('',(7.3576568875177,-4.35,100.7746996126));
#62880=CARTESIAN_POINT('Origin',(3.15,0.,102.306161475662));
#62881=CARTESIAN_POINT('',(3.15,-4.35,102.702683920339));
#62882=CARTESIAN_POINT('',(3.15,0.,102.702683920339));
#62883=CARTESIAN_POINT('',(3.15,-4.35,80.883169553523));
#62884=CARTESIAN_POINT('Origin',(3.15,0.,102.702683920339));
#62885=CARTESIAN_POINT('',(-7.17649681104826,-4.35,98.9441464568727));
#62886=CARTESIAN_POINT('Origin',(3.075,4.425,81.8256473496));
#62887=CARTESIAN_POINT('',(3.15,4.35,81.8256473496));
#62888=CARTESIAN_POINT('Origin',(4.55,0.,103.681558739843));
#62889=CARTESIAN_POINT('',(3.15,-4.35,104.191117067815));
#62890=CARTESIAN_POINT('',(3.15,0.,104.191117067815));
#62891=CARTESIAN_POINT('',(7.66056341237934,-4.35,102.549406245939));
#62892=CARTESIAN_POINT('Origin',(3.15,0.,104.191117067815));
#62893=CARTESIAN_POINT('',(3.15,-4.35,104.587639512493));
#62894=CARTESIAN_POINT('',(3.15,0.,104.587639512493));
#62895=CARTESIAN_POINT('',(3.15,-4.35,81.8256473496));
#62896=CARTESIAN_POINT('Origin',(3.15,0.,104.587639512493));
#62897=CARTESIAN_POINT('',(-7.47940333590974,-4.35,100.718853090212));
#62898=CARTESIAN_POINT('Origin',(3.075,4.425,82.7681251456769));
#62899=CARTESIAN_POINT('',(3.15,4.35,82.7681251456769));
#62900=CARTESIAN_POINT('Origin',(4.55,0.,105.566514331997));
#62901=CARTESIAN_POINT('',(3.15,-4.35,106.076072659969));
#62902=CARTESIAN_POINT('',(3.15,0.,106.076072659969));
#62903=CARTESIAN_POINT('',(7.96346993724081,-4.35,104.324112879278));
#62904=CARTESIAN_POINT('Origin',(3.15,0.,106.076072659969));
#62905=CARTESIAN_POINT('',(3.15,-4.35,106.472595104647));
#62906=CARTESIAN_POINT('',(3.15,0.,106.472595104647));
#62907=CARTESIAN_POINT('',(3.15,-4.35,82.7681251456769));
#62908=CARTESIAN_POINT('Origin',(3.15,0.,106.472595104647));
#62909=CARTESIAN_POINT('',(-7.78230986077121,-4.35,102.493559723551));
#62910=CARTESIAN_POINT('Origin',(3.075,4.425,83.7106029417538));
#62911=CARTESIAN_POINT('',(3.15,4.35,83.7106029417538));
#62912=CARTESIAN_POINT('Origin',(4.55,0.,107.451469924151));
#62913=CARTESIAN_POINT('',(3.15,-4.35,107.961028252123));
#62914=CARTESIAN_POINT('',(3.15,0.,107.961028252123));
#62915=CARTESIAN_POINT('',(8.26637646210229,-4.35,106.098819512618));
#62916=CARTESIAN_POINT('Origin',(3.15,0.,107.961028252123));
#62917=CARTESIAN_POINT('',(3.15,-4.35,108.357550696801));
#62918=CARTESIAN_POINT('',(3.15,0.,108.357550696801));
#62919=CARTESIAN_POINT('',(3.15,-4.35,83.7106029417538));
#62920=CARTESIAN_POINT('Origin',(3.15,0.,108.357550696801));
#62921=CARTESIAN_POINT('',(-8.08521638563253,-4.35,104.268266356891));
#62922=CARTESIAN_POINT('Origin',(3.075,4.425,84.6530807378308));
#62923=CARTESIAN_POINT('',(3.15,4.35,84.6530807378308));
#62924=CARTESIAN_POINT('Origin',(4.55,0.,109.336425516304));
#62925=CARTESIAN_POINT('',(3.15,-4.35,109.845983844277));
#62926=CARTESIAN_POINT('',(3.15,0.,109.845983844277));
#62927=CARTESIAN_POINT('',(8.56928298696376,-4.35,107.873526145957));
#62928=CARTESIAN_POINT('Origin',(3.15,0.,109.845983844277));
#62929=CARTESIAN_POINT('',(3.15,-4.35,110.242506288955));
#62930=CARTESIAN_POINT('',(3.15,0.,110.242506288955));
#62931=CARTESIAN_POINT('',(3.15,-4.35,84.6530807378308));
#62932=CARTESIAN_POINT('Origin',(3.15,0.,110.242506288955));
#62933=CARTESIAN_POINT('',(-8.38812291049415,-4.35,106.04297299023));
#62934=CARTESIAN_POINT('Origin',(3.075,4.425,85.5955585339077));
#62935=CARTESIAN_POINT('',(5.64277347156452,1.85722652843546,110.38200310527));
#62936=CARTESIAN_POINT('',(3.15,4.35,85.5955585339077));
#62937=CARTESIAN_POINT('Origin',(4.55,0.,111.221381108458));
#62938=CARTESIAN_POINT('',(3.15,-4.35,111.730939436431));
#62939=CARTESIAN_POINT('',(3.15,0.,111.730939436431));
#62940=CARTESIAN_POINT('',(8.87218951182523,-4.35,109.648232779296));
#62941=CARTESIAN_POINT('Origin',(3.15,0.,111.730939436431));
#62942=CARTESIAN_POINT('',(3.15,-4.35,85.5955585339077));
#62943=CARTESIAN_POINT('Origin',(-4.74308094908738,4.425,109.334428691923));
#62944=CARTESIAN_POINT('',(10.5341871605711,-1.68418716057113,108.393638360568));
#62945=CARTESIAN_POINT('Origin',(-10.8370266201352,-4.425,120.311103003503));
#62946=CARTESIAN_POINT('',(4.35,-4.5,125.918541973177));
#62947=CARTESIAN_POINT('',(11.4774798520793,2.62747985207928,120.927826852313));
#62948=CARTESIAN_POINT('',(3.,-4.5,125.427182156917));
#62949=CARTESIAN_POINT('',(-10.8626781308846,-4.5,120.381579950062));
#62950=CARTESIAN_POINT('',(3.,-4.5,125.427182156917));
#62951=CARTESIAN_POINT('Origin',(3.075,-4.425,92.1929031064463));
#62952=CARTESIAN_POINT('',(3.,-4.5,124.820597450777));
#62953=CARTESIAN_POINT('',(3.,-4.5,92.1929031064463));
#62954=CARTESIAN_POINT('',(3.,-4.5,124.820597450777));
#62955=CARTESIAN_POINT('Origin',(10.9668836751061,-4.425,122.000702266112));
#62956=CARTESIAN_POINT('',(4.35,-4.5,124.329237634517));
#62957=CARTESIAN_POINT('',(10.9412321643567,-4.5,121.930225319553));
#62958=CARTESIAN_POINT('',(-3.72343111062165,-12.5734311106217,118.676160311644));
#62959=CARTESIAN_POINT('Origin',(-4.5,-4.5,59.4601776313845));
#62960=CARTESIAN_POINT('',(4.35,-4.5,126.214193226671));
#62961=CARTESIAN_POINT('',(4.35,-4.5,59.4601776313845));
#62962=CARTESIAN_POINT('',(3.,-4.5,126.705553042931));
#62963=CARTESIAN_POINT('',(11.2441386892182,-4.5,123.704931952893));
#62964=CARTESIAN_POINT('',(3.,-4.5,127.312137749071));
#62965=CARTESIAN_POINT('',(3.,-4.5,93.1353809025232));
#62966=CARTESIAN_POINT('',(4.35,-4.5,127.80349756533));
#62967=CARTESIAN_POINT('',(-11.1655846557463,-4.5,122.156286583401));
#62968=CARTESIAN_POINT('',(4.35,-4.5,128.099148818825));
#62969=CARTESIAN_POINT('',(4.35,-4.5,59.4601776313845));
#62970=CARTESIAN_POINT('',(2.99999999999999,-4.5,128.590508635084));
#62971=CARTESIAN_POINT('',(11.5470452140794,-4.5,125.479638586232));
#62972=CARTESIAN_POINT('',(3.,-4.5,129.197093341225));
#62973=CARTESIAN_POINT('',(3.,-4.5,94.0778586986002));
#62974=CARTESIAN_POINT('',(4.35,-4.5,129.688453157484));
#62975=CARTESIAN_POINT('',(-11.4684911806075,-4.5,123.930993216741));
#62976=CARTESIAN_POINT('',(4.35,-4.5,59.4601776313845));
#62977=CARTESIAN_POINT('',(4.35,-4.5,59.9101776313845));
#62978=CARTESIAN_POINT('',(-3.375,-4.5,59.9101776313845));
#62979=CARTESIAN_POINT('',(4.35,-4.5,59.4601776313845));
#62980=CARTESIAN_POINT('',(3.,-4.5,70.7634699844547));
#62981=CARTESIAN_POINT('',(3.,-4.5,64.8610470202151));
#62982=CARTESIAN_POINT('',(4.35,-4.5,71.2548298007141));
#62983=CARTESIAN_POINT('',(-2.07838890990205,-4.5,68.9150875832228));
#62984=CARTESIAN_POINT('',(4.35,-4.5,71.5504810542087));
#62985=CARTESIAN_POINT('',(4.35,-4.5,59.4601776313845));
#62986=CARTESIAN_POINT('',(3.,-4.5,72.0418408704681));
#62987=CARTESIAN_POINT('',(2.45984946823538,-4.5,72.2384395860535));
#62988=CARTESIAN_POINT('',(3.,-4.5,72.6484255766087));
#62989=CARTESIAN_POINT('',(3.,-4.5,65.803524816292));
#62990=CARTESIAN_POINT('',(4.35,-4.5,73.139785392868));
#62991=CARTESIAN_POINT('',(-2.38129543476353,-4.5,70.6897942165621));
#62992=CARTESIAN_POINT('',(4.35,-4.5,73.4354366463626));
#62993=CARTESIAN_POINT('',(4.35,-4.5,59.4601776313845));
#62994=CARTESIAN_POINT('',(3.,-4.5,73.926796462622));
#62995=CARTESIAN_POINT('',(2.76275599309685,-4.5,74.0131462193928));
#62996=CARTESIAN_POINT('',(3.,-4.5,66.746002612369));
#62997=CARTESIAN_POINT('',(3.,-4.5,75.8117520547759));
#62998=CARTESIAN_POINT('',(3.06566251795832,-4.5,75.7878528527321));
#62999=CARTESIAN_POINT('',(3.,-4.5,76.4183367609164));
#63000=CARTESIAN_POINT('',(3.,-4.5,67.6884804084459));
#63001=CARTESIAN_POINT('',(4.35,-4.5,76.9096965771758));
#63002=CARTESIAN_POINT('',(-2.98710848448645,-4.5,74.2392074832407));
#63003=CARTESIAN_POINT('',(4.35,-4.5,77.2053478306704));
#63004=CARTESIAN_POINT('',(4.35,-4.5,59.4601776313845));
#63005=CARTESIAN_POINT('',(3.,-4.5,77.6967076469297));
#63006=CARTESIAN_POINT('',(3.36856904281978,-4.5,77.5625594860714));
#63007=CARTESIAN_POINT('',(3.,-4.5,68.6309582045228));
#63008=CARTESIAN_POINT('',(4.35,-4.5,79.0903034228242));
#63009=CARTESIAN_POINT('',(4.35,-4.5,59.4601776313845));
#63010=CARTESIAN_POINT('',(3.,-4.5,79.5816632390836));
#63011=CARTESIAN_POINT('',(3.67147556768125,-4.5,79.3372661194106));
#63012=CARTESIAN_POINT('',(3.,-4.5,80.1882479452242));
#63013=CARTESIAN_POINT('',(3.,-4.5,69.5734360005998));
#63014=CARTESIAN_POINT('',(4.35,-4.5,80.6796077614835));
#63015=CARTESIAN_POINT('',(-3.59292153420939,-4.5,77.7886207499193));
#63016=CARTESIAN_POINT('',(4.35,-4.5,80.9752590149781));
#63017=CARTESIAN_POINT('',(4.35,-4.5,59.4601776313845));
#63018=CARTESIAN_POINT('',(3.,-4.5,81.4666188312375));
#63019=CARTESIAN_POINT('',(3.97438209254272,-4.5,81.1119727527499));
#63020=CARTESIAN_POINT('',(3.,-4.5,82.073203537378));
#63021=CARTESIAN_POINT('',(3.,-4.5,70.5159137966767));
#63022=CARTESIAN_POINT('',(4.35,-4.5,82.5645633536374));
#63023=CARTESIAN_POINT('',(-3.89582805907085,-4.5,79.5633273832586));
#63024=CARTESIAN_POINT('',(4.35,-4.5,59.4601776313845));
#63025=CARTESIAN_POINT('',(3.,-4.5,83.9581591295319));
#63026=CARTESIAN_POINT('',(3.,-4.5,71.4583915927537));
#63027=CARTESIAN_POINT('',(4.35,-4.5,84.4495189457913));
#63028=CARTESIAN_POINT('',(-4.19873458393231,-4.5,81.3380340165978));
#63029=CARTESIAN_POINT('',(4.35,-4.5,84.7451701992859));
#63030=CARTESIAN_POINT('',(4.35,-4.5,59.4601776313845));
#63031=CARTESIAN_POINT('',(3.,-4.5,85.2365300155452));
#63032=CARTESIAN_POINT('',(4.58019514226565,-4.5,84.6613860194285));
#63033=CARTESIAN_POINT('',(3.,-4.5,85.8431147216858));
#63034=CARTESIAN_POINT('',(3.,-4.5,72.4008693888306));
#63035=CARTESIAN_POINT('',(4.35,-4.5,86.3344745379451));
#63036=CARTESIAN_POINT('',(-4.50164110879379,-4.5,83.1127406499371));
#63037=CARTESIAN_POINT('',(4.35,-4.5,86.6301257914398));
#63038=CARTESIAN_POINT('',(4.35,-4.5,59.4601776313845));
#63039=CARTESIAN_POINT('',(3.,-4.5,87.1214856076991));
#63040=CARTESIAN_POINT('',(4.88310166712712,-4.5,86.4360926527678));
#63041=CARTESIAN_POINT('',(3.,-4.5,73.3433471849075));
#63042=CARTESIAN_POINT('',(3.,-4.5,89.006441199853));
#63043=CARTESIAN_POINT('',(5.18600819198858,-4.5,88.2107992861071));
#63044=CARTESIAN_POINT('',(3.,-4.5,89.6130259059935));
#63045=CARTESIAN_POINT('',(3.,-4.5,74.2858249809845));
#63046=CARTESIAN_POINT('',(4.35,-4.5,90.1043857222529));
#63047=CARTESIAN_POINT('',(-5.10745415851671,-4.5,86.6621539166157));
#63048=CARTESIAN_POINT('',(4.35,-4.5,90.4000369757475));
#63049=CARTESIAN_POINT('',(4.35,-4.5,59.4601776313845));
#63050=CARTESIAN_POINT('',(2.99999999999999,-4.5,90.8913967920069));
#63051=CARTESIAN_POINT('',(5.48891471685005,-4.5,89.9855059194464));
#63052=CARTESIAN_POINT('',(3.,-4.5,91.4979814981474));
#63053=CARTESIAN_POINT('',(3.,-4.5,75.2283027770614));
#63054=CARTESIAN_POINT('',(4.35,-4.5,91.9893413144068));
#63055=CARTESIAN_POINT('',(-5.41036068337819,-4.5,88.436860549955));
#63056=CARTESIAN_POINT('',(4.35,-4.5,92.2849925679014));
#63057=CARTESIAN_POINT('',(4.35,-4.5,59.4601776313845));
#63058=CARTESIAN_POINT('',(3.,-4.5,92.7763523841608));
#63059=CARTESIAN_POINT('',(5.79182124171152,-4.5,91.7602125527857));
#63060=CARTESIAN_POINT('',(3.,-4.5,93.3829370903013));
#63061=CARTESIAN_POINT('',(3.,-4.5,76.1707805731383));
#63062=CARTESIAN_POINT('',(4.35,-4.5,93.8742969065607));
#63063=CARTESIAN_POINT('',(-5.71326720823965,-4.5,90.2115671832943));
#63064=CARTESIAN_POINT('',(4.35,-4.5,94.1699481600552));
#63065=CARTESIAN_POINT('',(4.35,-4.5,59.4601776313845));
#63066=CARTESIAN_POINT('',(3.,-4.5,94.6613079763146));
#63067=CARTESIAN_POINT('',(6.09472776657299,-4.5,93.5349191861249));
#63068=CARTESIAN_POINT('',(3.,-4.5,77.1132583692153));
#63069=CARTESIAN_POINT('',(4.35,-4.5,96.0549037522091));
#63070=CARTESIAN_POINT('',(4.35,-4.5,59.4601776313845));
#63071=CARTESIAN_POINT('',(2.99999999999999,-4.5,96.5462635684685));
#63072=CARTESIAN_POINT('',(6.39763429143445,-4.5,95.3096258194642));
#63073=CARTESIAN_POINT('',(3.,-4.5,97.152848274609));
#63074=CARTESIAN_POINT('',(3.,-4.5,78.0557361652922));
#63075=CARTESIAN_POINT('',(4.35,-4.5,97.6442080908684));
#63076=CARTESIAN_POINT('',(-6.31908025796259,-4.5,93.7609804499728));
#63077=CARTESIAN_POINT('',(4.35,-4.5,97.939859344363));
#63078=CARTESIAN_POINT('',(4.35,-4.5,59.4601776313845));
#63079=CARTESIAN_POINT('',(3.,-4.5,98.4312191606224));
#63080=CARTESIAN_POINT('',(6.70054081629591,-4.5,97.0843324528035));
#63081=CARTESIAN_POINT('',(3.,-4.5,99.0378038667629));
#63082=CARTESIAN_POINT('',(3.,-4.5,78.9982139613691));
#63083=CARTESIAN_POINT('',(4.35,-4.5,99.5291636830223));
#63084=CARTESIAN_POINT('',(-6.62198678282405,-4.5,95.5356870833121));
#63085=CARTESIAN_POINT('',(4.35,-4.5,59.4601776313845));
#63086=CARTESIAN_POINT('',(3.,-4.5,100.922759458917));
#63087=CARTESIAN_POINT('',(3.,-4.5,79.9406917574461));
#63088=CARTESIAN_POINT('',(4.35,-4.5,101.414119275176));
#63089=CARTESIAN_POINT('',(-6.92489330768551,-4.5,97.3103937166514));
#63090=CARTESIAN_POINT('',(4.35,-4.5,101.709770528671));
#63091=CARTESIAN_POINT('',(4.35,-4.5,59.4601776313845));
#63092=CARTESIAN_POINT('',(3.,-4.5,102.20113034493));
#63093=CARTESIAN_POINT('',(7.30635386601885,-4.5,100.633745719482));
#63094=CARTESIAN_POINT('',(3.,-4.5,102.807715051071));
#63095=CARTESIAN_POINT('',(3.,-4.5,80.883169553523));
#63096=CARTESIAN_POINT('',(4.35,-4.5,103.29907486733));
#63097=CARTESIAN_POINT('',(-7.22779983254711,-4.5,99.0851003499905));
#63098=CARTESIAN_POINT('',(4.35,-4.5,103.594726120825));
#63099=CARTESIAN_POINT('',(4.35,-4.5,59.4601776313845));
#63100=CARTESIAN_POINT('',(3.,-4.5,104.086085937084));
#63101=CARTESIAN_POINT('',(7.60926039088049,-4.5,102.408452352821));
#63102=CARTESIAN_POINT('',(3.,-4.5,104.692670643225));
#63103=CARTESIAN_POINT('',(3.,-4.5,81.8256473496));
#63104=CARTESIAN_POINT('',(4.35,-4.5,105.184030459484));
#63105=CARTESIAN_POINT('',(-7.53070635740859,-4.5,100.85980698333));
#63106=CARTESIAN_POINT('',(4.35,-4.5,105.479681712979));
#63107=CARTESIAN_POINT('',(4.35,-4.5,59.4601776313845));
#63108=CARTESIAN_POINT('',(3.,-4.5,105.971041529238));
#63109=CARTESIAN_POINT('',(7.91216691574196,-4.5,104.183158986161));
#63110=CARTESIAN_POINT('',(3.,-4.5,106.577626235378));
#63111=CARTESIAN_POINT('',(3.,-4.5,82.7681251456769));
#63112=CARTESIAN_POINT('',(4.35,-4.5,107.068986051638));
#63113=CARTESIAN_POINT('',(-7.83361288227006,-4.5,102.634513616669));
#63114=CARTESIAN_POINT('',(4.35,-4.5,107.364637305132));
#63115=CARTESIAN_POINT('',(4.35,-4.5,59.4601776313845));
#63116=CARTESIAN_POINT('',(3.,-4.5,107.855997121392));
#63117=CARTESIAN_POINT('',(8.21507344060344,-4.5,105.9578656195));
#63118=CARTESIAN_POINT('',(3.,-4.5,108.462581827532));
#63119=CARTESIAN_POINT('',(3.,-4.5,83.7106029417538));
#63120=CARTESIAN_POINT('',(4.35,-4.5,108.953941643792));
#63121=CARTESIAN_POINT('',(-8.13651940713138,-4.5,104.409220250009));
#63122=CARTESIAN_POINT('',(4.35,-4.5,109.249592897286));
#63123=CARTESIAN_POINT('',(4.35,-4.5,59.4601776313845));
#63124=CARTESIAN_POINT('',(3.,-4.5,109.740952713546));
#63125=CARTESIAN_POINT('',(8.51797996546491,-4.5,107.732572252839));
#63126=CARTESIAN_POINT('',(3.,-4.5,110.347537419686));
#63127=CARTESIAN_POINT('',(3.,-4.5,84.6530807378308));
#63128=CARTESIAN_POINT('',(4.35,-4.5,110.838897235946));
#63129=CARTESIAN_POINT('',(-8.43942593199301,-4.5,106.183926883348));
#63130=CARTESIAN_POINT('',(4.35,-4.5,111.13454848944));
#63131=CARTESIAN_POINT('',(4.35,-4.5,59.4601776313845));
#63132=CARTESIAN_POINT('',(3.,-4.5,111.6259083057));
#63133=CARTESIAN_POINT('',(8.82088649032638,-4.5,109.507278886178));
#63134=CARTESIAN_POINT('',(3.,-4.5,85.5955585339077));
#63135=CARTESIAN_POINT('',(3.,-4.5,114.117448603994));
#63136=CARTESIAN_POINT('',(3.,-4.5,86.5380363299847));
#63137=CARTESIAN_POINT('',(4.35,-4.5,114.608808420253));
#63138=CARTESIAN_POINT('',(-9.04523898171578,-4.5,109.733340150026));
#63139=CARTESIAN_POINT('',(4.35,-4.5,114.904459673748));
#63140=CARTESIAN_POINT('',(4.35,-4.5,59.4601776313845));
#63141=CARTESIAN_POINT('',(3.,-4.5,115.395819490007));
#63142=CARTESIAN_POINT('',(9.42669954004933,-4.5,113.056692152857));
#63143=CARTESIAN_POINT('',(3.,-4.5,116.002404196148));
#63144=CARTESIAN_POINT('',(3.,-4.5,87.4805141260616));
#63145=CARTESIAN_POINT('',(4.35,-4.5,116.493764012407));
#63146=CARTESIAN_POINT('',(-9.34814550657743,-4.5,111.508046783366));
#63147=CARTESIAN_POINT('',(4.35,-4.5,116.789415265902));
#63148=CARTESIAN_POINT('',(4.35,-4.5,59.4601776313845));
#63149=CARTESIAN_POINT('',(3.,-4.5,117.280775082161));
#63150=CARTESIAN_POINT('',(9.7296060649108,-4.5,114.831398786196));
#63151=CARTESIAN_POINT('',(3.,-4.5,88.4229919221386));
#63152=CARTESIAN_POINT('',(4.35,-4.5,118.674370858056));
#63153=CARTESIAN_POINT('',(4.35,-4.5,59.4601776313845));
#63154=CARTESIAN_POINT('',(3.,-4.5,119.165730674315));
#63155=CARTESIAN_POINT('',(10.0325125897723,-4.5,116.606105419536));
#63156=CARTESIAN_POINT('',(3.,-4.5,119.772315380456));
#63157=CARTESIAN_POINT('',(3.,-4.5,89.3654697182155));
#63158=CARTESIAN_POINT('',(4.35,-4.5,120.263675196715));
#63159=CARTESIAN_POINT('',(-9.95395855630018,-4.5,115.057460050044));
#63160=CARTESIAN_POINT('',(4.35,-4.5,120.559326450209));
#63161=CARTESIAN_POINT('',(4.35,-4.5,59.4601776313845));
#63162=CARTESIAN_POINT('',(3.,-4.5,121.050686266469));
#63163=CARTESIAN_POINT('',(10.3354191146337,-4.5,118.380812052875));
#63164=CARTESIAN_POINT('',(3.,-4.5,121.657270972609));
#63165=CARTESIAN_POINT('',(3.,-4.5,90.3079475142924));
#63166=CARTESIAN_POINT('',(4.35,-4.5,122.148630788869));
#63167=CARTESIAN_POINT('',(-10.2568650811618,-4.5,116.832166683383));
#63168=CARTESIAN_POINT('',(4.35,-4.5,122.444282042363));
#63169=CARTESIAN_POINT('',(4.35,-4.5,59.4601776313845));
#63170=CARTESIAN_POINT('',(3.,-4.5,122.935641858623));
#63171=CARTESIAN_POINT('',(10.6383256394952,-4.5,120.155518686214));
#63172=CARTESIAN_POINT('',(3.,-4.5,123.542226564763));
#63173=CARTESIAN_POINT('',(3.,-4.5,91.2504253103694));
#63174=CARTESIAN_POINT('',(4.35,-4.5,124.033586381023));
#63175=CARTESIAN_POINT('',(-10.5597716060233,-4.5,118.606873316723));
#63176=CARTESIAN_POINT('',(4.35,-4.5,59.4601776313845));
#63177=CARTESIAN_POINT('',(1.10830535322836E-16,-4.5,60.5551776313845));
#63178=CARTESIAN_POINT('Origin',(0.,-4.5,61.4601776313845));
#63179=CARTESIAN_POINT('Origin',(4.425,-4.425,59.4601776313845));
#63180=CARTESIAN_POINT('',(-3.94311445671589,-12.7931144567159,120.407291968843));
#63181=CARTESIAN_POINT('Origin',(-10.5341200952739,-4.425,118.536396370164));
#63182=CARTESIAN_POINT('',(11.2577965059859,2.4077965059859,119.196695195113));
#63183=CARTESIAN_POINT('',(3.,-4.5,123.542226564763));
#63184=CARTESIAN_POINT('Origin',(3.075,-4.425,91.2504253103694));
#63185=CARTESIAN_POINT('',(3.,-4.5,122.935641858623));
#63186=CARTESIAN_POINT('Origin',(10.6639771502446,-4.425,120.225995632773));
#63187=CARTESIAN_POINT('',(-3.50374776452922,-12.3537477645292,116.945028654443));
#63188=CARTESIAN_POINT('Origin',(4.425,-4.425,59.4601776313845));
#63189=CARTESIAN_POINT('Origin',(-10.2312135704124,-4.425,116.761689736824));
#63190=CARTESIAN_POINT('',(11.0381131598936,2.18811315989359,117.465563537911));
#63191=CARTESIAN_POINT('',(3.,-4.5,121.657270972609));
#63192=CARTESIAN_POINT('Origin',(3.075,-4.425,90.3079475142924));
#63193=CARTESIAN_POINT('',(3.,-4.5,121.050686266469));
#63194=CARTESIAN_POINT('Origin',(10.3610706253832,-4.425,118.451288999434));
#63195=CARTESIAN_POINT('',(-3.28406441843662,-12.1340644184366,115.213896997241));
#63196=CARTESIAN_POINT('Origin',(4.425,-4.425,59.4601776313845));
#63197=CARTESIAN_POINT('Origin',(-9.92830704555076,-4.425,114.986983103485));
#63198=CARTESIAN_POINT('',(10.8184298137991,1.96842981379911,115.734431880713));
#63199=CARTESIAN_POINT('',(3.,-4.5,119.772315380456));
#63200=CARTESIAN_POINT('Origin',(3.075,-4.425,89.3654697182155));
#63201=CARTESIAN_POINT('',(3.,-4.5,119.165730674315));
#63202=CARTESIAN_POINT('Origin',(10.0581641005217,-4.425,116.676582366094));
#63203=CARTESIAN_POINT('',(-3.06438107234234,-11.9143810723423,113.482765340042));
#63204=CARTESIAN_POINT('Origin',(4.425,-4.425,59.4601776313845));
#63205=CARTESIAN_POINT('Origin',(3.075,-4.425,88.4229919221386));
#63206=CARTESIAN_POINT('',(3.,-4.5,117.280775082161));
#63207=CARTESIAN_POINT('Origin',(9.75525757566023,-4.425,114.901875732755));
#63208=CARTESIAN_POINT('',(-2.84469772624895,-11.694697726249,111.751633682842));
#63209=CARTESIAN_POINT('Origin',(4.425,-4.425,59.4601776313845));
#63210=CARTESIAN_POINT('',(4.5,-4.35,59.4601776313845));
#63211=CARTESIAN_POINT('Origin',(-9.322493995828,-4.425,111.437569836807));
#63212=CARTESIAN_POINT('',(10.3790631216133,1.52906312161332,112.272168566311));
#63213=CARTESIAN_POINT('',(3.,-4.5,116.002404196148));
#63214=CARTESIAN_POINT('Origin',(3.075,-4.425,87.4805141260616));
#63215=CARTESIAN_POINT('',(3.,-4.5,115.395819490007));
#63216=CARTESIAN_POINT('Origin',(9.45235105079875,-4.425,113.127169099416));
#63217=CARTESIAN_POINT('',(-2.62501438015637,-11.4750143801564,110.020502025641));
#63218=CARTESIAN_POINT('Origin',(4.425,-4.425,59.4601776313845));
#63219=CARTESIAN_POINT('Origin',(-9.01958747096636,-4.425,109.662863203467));
#63220=CARTESIAN_POINT('',(10.159379775519,1.30937977551898,110.541036909112));
#63221=CARTESIAN_POINT('',(5.13546547427087,-2.36453452572912,112.622179581323));
#63222=CARTESIAN_POINT('Origin',(3.075,-4.425,86.5380363299847));
#63223=CARTESIAN_POINT('Origin',(3.075,-4.425,85.5955585339077));
#63224=CARTESIAN_POINT('',(3.,-4.5,111.6259083057));
#63225=CARTESIAN_POINT('Origin',(8.84653800107581,-4.425,109.577755832737));
#63226=CARTESIAN_POINT('',(-2.18564768796881,-11.0356476879688,106.558238711242));
#63227=CARTESIAN_POINT('Origin',(-8.41377442124358,-4.425,106.113449936789));
#63228=CARTESIAN_POINT('',(9.72001308333303,0.870013083333027,107.078773594711));
#63229=CARTESIAN_POINT('',(3.,-4.5,110.347537419686));
#63230=CARTESIAN_POINT('Origin',(3.075,-4.425,84.6530807378308));
#63231=CARTESIAN_POINT('',(3.,-4.5,109.740952713546));
#63232=CARTESIAN_POINT('Origin',(8.54363147621433,-4.425,107.803049199398));
#63233=CARTESIAN_POINT('',(-1.96596434187612,-10.8159643418761,104.82710705404));
#63234=CARTESIAN_POINT('Origin',(4.425,-4.425,59.4601776313845));
#63235=CARTESIAN_POINT('Origin',(-8.11086789638195,-4.425,104.33874330345));
#63236=CARTESIAN_POINT('',(9.50032973723794,0.650329737237946,105.347641937513));
#63237=CARTESIAN_POINT('',(3.,-4.5,108.462581827532));
#63238=CARTESIAN_POINT('Origin',(3.075,-4.425,83.7106029417538));
#63239=CARTESIAN_POINT('',(3.,-4.5,107.855997121392));
#63240=CARTESIAN_POINT('Origin',(8.24072495135287,-4.425,106.028342566059));
#63241=CARTESIAN_POINT('',(-1.74628099578204,-10.596280995782,103.095975396841));
#63242=CARTESIAN_POINT('Origin',(4.425,-4.425,59.4601776313845));
#63243=CARTESIAN_POINT('Origin',(-7.80796137152063,-4.425,102.56403667011));
#63244=CARTESIAN_POINT('',(9.28064639114536,0.430646391145358,103.616510280312));
#63245=CARTESIAN_POINT('',(3.,-4.5,106.577626235378));
#63246=CARTESIAN_POINT('Origin',(3.075,-4.425,82.7681251456769));
#63247=CARTESIAN_POINT('',(3.,-4.5,105.971041529238));
#63248=CARTESIAN_POINT('Origin',(7.93781842649139,-4.425,104.253635932719));
#63249=CARTESIAN_POINT('',(-1.52659764968865,-10.3765976496886,101.364843739641));
#63250=CARTESIAN_POINT('Origin',(4.425,-4.425,59.4601776313845));
#63251=CARTESIAN_POINT('Origin',(-7.50505484665916,-4.425,100.789330036771));
#63252=CARTESIAN_POINT('',(9.06096304505277,0.210963045052771,101.88537862311));
#63253=CARTESIAN_POINT('',(3.,-4.5,104.692670643225));
#63254=CARTESIAN_POINT('Origin',(3.075,-4.425,81.8256473496));
#63255=CARTESIAN_POINT('',(3.,-4.5,104.086085937084));
#63256=CARTESIAN_POINT('Origin',(7.63491190162991,-4.425,102.47892929938));
#63257=CARTESIAN_POINT('',(-1.30691430359526,-10.1569143035953,99.6337120824411));
#63258=CARTESIAN_POINT('Origin',(4.425,-4.425,59.4601776313845));
#63259=CARTESIAN_POINT('Origin',(-7.20214832179769,-4.425,99.0146234034316));
#63260=CARTESIAN_POINT('',(8.84127969895858,-0.00872030104142052,100.154246965911));
#63261=CARTESIAN_POINT('',(3.,-4.5,102.807715051071));
#63262=CARTESIAN_POINT('Origin',(3.075,-4.425,80.883169553523));
#63263=CARTESIAN_POINT('',(3.,-4.5,102.20113034493));
#63264=CARTESIAN_POINT('Origin',(7.33200537676827,-4.425,100.704222666041));
#63265=CARTESIAN_POINT('',(-1.08723095750194,-9.93723095750194,97.9025804252409));
#63266=CARTESIAN_POINT('Origin',(4.425,-4.425,59.4601776313845));
#63267=CARTESIAN_POINT('Origin',(-6.89924179693609,-4.425,97.2399167700925));
#63268=CARTESIAN_POINT('',(8.62159635286518,-0.22840364713482,98.423115308711));
#63269=CARTESIAN_POINT('',(3.,-4.5,100.922759458917));
#63270=CARTESIAN_POINT('Origin',(3.075,-4.425,79.9406917574461));
#63271=CARTESIAN_POINT('Origin',(4.425,-4.425,59.4601776313845));
#63272=CARTESIAN_POINT('Origin',(-6.59633527207463,-4.425,95.4652101367532));
#63273=CARTESIAN_POINT('',(8.40191300677184,-0.448086993228164,96.6919836515108));
#63274=CARTESIAN_POINT('',(3.,-4.5,99.0378038667629));
#63275=CARTESIAN_POINT('Origin',(3.075,-4.425,78.9982139613691));
#63276=CARTESIAN_POINT('',(3.,-4.5,98.4312191606224));
#63277=CARTESIAN_POINT('Origin',(6.72619232704534,-4.425,97.1548093993624));
#63278=CARTESIAN_POINT('',(-0.647864265315112,-9.49786426531512,94.4403171108406));
#63279=CARTESIAN_POINT('Origin',(4.425,-4.425,59.4601776313845));
#63280=CARTESIAN_POINT('Origin',(-6.29342874721316,-4.425,93.6905035034139));
#63281=CARTESIAN_POINT('',(8.18222966067847,-0.667770339321526,94.9608519943106));
#63282=CARTESIAN_POINT('',(3.,-4.5,97.152848274609));
#63283=CARTESIAN_POINT('Origin',(3.075,-4.425,78.0557361652922));
#63284=CARTESIAN_POINT('',(3.,-4.5,96.5462635684685));
#63285=CARTESIAN_POINT('Origin',(6.42328580218387,-4.425,95.3801027660232));
#63286=CARTESIAN_POINT('',(-0.428180919221253,-9.27818091922125,92.7091854536413));
#63287=CARTESIAN_POINT('Origin',(4.425,-4.425,59.4601776313845));
#63288=CARTESIAN_POINT('Origin',(3.075,-4.425,77.1132583692153));
#63289=CARTESIAN_POINT('',(3.,-4.5,94.6613079763146));
#63290=CARTESIAN_POINT('Origin',(6.12037927732241,-4.425,93.6053961326839));
#63291=CARTESIAN_POINT('',(-0.208497573127868,-9.05849757312787,90.9780537964411));
#63292=CARTESIAN_POINT('Origin',(4.425,-4.425,59.4601776313845));
#63293=CARTESIAN_POINT('',(4.5,-4.35,59.4601776313845));
#63294=CARTESIAN_POINT('Origin',(-5.68761569749023,-4.425,90.1410902367353));
#63295=CARTESIAN_POINT('',(7.74286296849167,-1.10713703150834,91.4985886799104));
#63296=CARTESIAN_POINT('',(3.,-4.5,93.3829370903013));
#63297=CARTESIAN_POINT('Origin',(3.075,-4.425,76.1707805731383));
#63298=CARTESIAN_POINT('',(3.,-4.5,92.7763523841608));
#63299=CARTESIAN_POINT('Origin',(5.81747275246094,-4.425,91.8306894993446));
#63300=CARTESIAN_POINT('',(0.0111857729655158,-8.83881422703448,89.246922139241));
#63301=CARTESIAN_POINT('Origin',(4.425,-4.425,59.4601776313845));
#63302=CARTESIAN_POINT('Origin',(-5.38470917262876,-4.425,88.366383603396));
#63303=CARTESIAN_POINT('',(7.5231796223983,-1.3268203776017,89.7674570227101));
#63304=CARTESIAN_POINT('',(3.,-4.5,91.4979814981474));
#63305=CARTESIAN_POINT('Origin',(3.075,-4.425,75.2283027770614));
#63306=CARTESIAN_POINT('',(3.,-4.5,90.8913967920069));
#63307=CARTESIAN_POINT('Origin',(5.51456622759947,-4.425,90.0559828660053));
#63308=CARTESIAN_POINT('',(0.230869119058417,-8.61913088094158,87.5157904820399));
#63309=CARTESIAN_POINT('Origin',(4.425,-4.425,59.4601776313845));
#63310=CARTESIAN_POINT('Origin',(-5.08180264776729,-4.425,86.5916769700568));
#63311=CARTESIAN_POINT('',(7.30349627630486,-1.54650372369514,88.0363253655101));
#63312=CARTESIAN_POINT('',(3.,-4.5,89.6130259059935));
#63313=CARTESIAN_POINT('Origin',(3.075,-4.425,74.2858249809845));
#63314=CARTESIAN_POINT('',(1.31774799117218,-6.18225200882782,87.8285156621034));
#63315=CARTESIAN_POINT('Origin',(5.21165970273801,-4.425,88.281276232666));
#63316=CARTESIAN_POINT('Origin',(3.075,-4.425,73.3433471849075));
#63317=CARTESIAN_POINT('',(3.,-4.5,87.1214856076991));
#63318=CARTESIAN_POINT('Origin',(4.90875317787654,-4.425,86.5065695993267));
#63319=CARTESIAN_POINT('',(0.670235811245595,-8.1797641887544,84.0535271676404));
#63320=CARTESIAN_POINT('Origin',(-4.47598959804436,-4.425,83.0422637033782));
#63321=CARTESIAN_POINT('',(6.86412958411812,-1.98587041588188,84.5740620511097));
#63322=CARTESIAN_POINT('',(3.,-4.5,85.8431147216858));
#63323=CARTESIAN_POINT('Origin',(3.075,-4.425,72.4008693888306));
#63324=CARTESIAN_POINT('',(3.,-4.5,85.2365300155452));
#63325=CARTESIAN_POINT('Origin',(4.60584665301507,-4.425,84.7318629659874));
#63326=CARTESIAN_POINT('',(0.889919157338593,-7.96008084266141,82.3223955104395));
#63327=CARTESIAN_POINT('Origin',(4.425,-4.425,59.4601776313845));
#63328=CARTESIAN_POINT('Origin',(-4.17308307318289,-4.425,81.2675570700389));
#63329=CARTESIAN_POINT('',(6.64444623802422,-2.20555376197578,82.8429303939101));
#63330=CARTESIAN_POINT('',(3.,-4.5,83.9581591295319));
#63331=CARTESIAN_POINT('Origin',(3.075,-4.425,71.4583915927537));
#63332=CARTESIAN_POINT('Origin',(4.425,-4.425,59.4601776313845));
#63333=CARTESIAN_POINT('Origin',(-3.87017654832143,-4.425,79.4928504366996));
#63334=CARTESIAN_POINT('',(6.42476289193132,-2.42523710806868,81.1117987367094));
#63335=CARTESIAN_POINT('',(3.,-4.5,82.073203537378));
#63336=CARTESIAN_POINT('Origin',(3.075,-4.425,70.5159137966767));
#63337=CARTESIAN_POINT('',(3.,-4.5,81.4666188312375));
#63338=CARTESIAN_POINT('Origin',(4.00003360329214,-4.425,81.1824496993089));
#63339=CARTESIAN_POINT('',(1.32928584952567,-7.52071415047433,78.8601321960397));
#63340=CARTESIAN_POINT('Origin',(4.425,-4.425,59.4601776313845));
#63341=CARTESIAN_POINT('Origin',(-3.56727002345996,-4.425,77.7181438033603));
#63342=CARTESIAN_POINT('',(6.20507954583794,-2.64492045416205,79.3806670795092));
#63343=CARTESIAN_POINT('',(3.,-4.5,80.1882479452242));
#63344=CARTESIAN_POINT('Origin',(3.075,-4.425,69.5734360005998));
#63345=CARTESIAN_POINT('',(3.,-4.5,79.5816632390836));
#63346=CARTESIAN_POINT('Origin',(3.69712707843067,-4.425,79.4077430659696));
#63347=CARTESIAN_POINT('',(1.54896919561877,-7.30103080438123,77.129000538839));
#63348=CARTESIAN_POINT('Origin',(4.425,-4.425,59.4601776313845));
#63349=CARTESIAN_POINT('Origin',(3.075,-4.425,68.6309582045228));
#63350=CARTESIAN_POINT('',(3.,-4.5,77.6967076469297));
#63351=CARTESIAN_POINT('Origin',(3.39422055356921,-4.425,77.6330364326303));
#63352=CARTESIAN_POINT('',(1.76865254171217,-7.08134745828783,75.3978688816388));
#63353=CARTESIAN_POINT('Origin',(4.425,-4.425,59.4601776313845));
#63354=CARTESIAN_POINT('',(4.5,-4.35,59.4601776313845));
#63355=CARTESIAN_POINT('Origin',(-2.96145697373703,-4.425,74.1687305366817));
#63356=CARTESIAN_POINT('',(5.7657128536508,-3.0842871463492,75.9184037651093));
#63357=CARTESIAN_POINT('',(3.39181079723248,-4.10818920276752,76.1439878871423));
#63358=CARTESIAN_POINT('Origin',(3.075,-4.425,67.6884804084459));
#63359=CARTESIAN_POINT('',(3.,-4.5,75.8117520547759));
#63360=CARTESIAN_POINT('Origin',(3.09131402870775,-4.425,75.858329799291));
#63361=CARTESIAN_POINT('Origin',(3.075,-4.425,66.746002612369));
#63362=CARTESIAN_POINT('',(3.,-4.5,73.926796462622));
#63363=CARTESIAN_POINT('Origin',(2.78840750384627,-4.425,74.0836231659517));
#63364=CARTESIAN_POINT('',(2.20801923389894,-6.64198076610106,71.9356055672385));
#63365=CARTESIAN_POINT('Origin',(-2.3556439240141,-4.425,70.6193172700032));
#63366=CARTESIAN_POINT('',(5.32634616146465,-3.52365383853535,72.4561404507083));
#63367=CARTESIAN_POINT('',(3.,-4.5,72.6484255766087));
#63368=CARTESIAN_POINT('Origin',(3.075,-4.425,65.803524816292));
#63369=CARTESIAN_POINT('',(3.,-4.5,72.0418408704681));
#63370=CARTESIAN_POINT('Origin',(2.48550097898481,-4.425,72.3089165326124));
#63371=CARTESIAN_POINT('',(2.42770257999234,-6.42229742000766,70.2044739100384));
#63372=CARTESIAN_POINT('Origin',(4.425,-4.425,59.4601776313845));
#63373=CARTESIAN_POINT('Origin',(-2.05273739915263,-4.425,68.8446106366639));
#63374=CARTESIAN_POINT('',(5.10666281537071,-3.74333718462929,70.7250087935087));
#63375=CARTESIAN_POINT('',(3.,-4.5,70.7634699844547));
#63376=CARTESIAN_POINT('Origin',(3.075,-4.425,64.8610470202151));
#63377=CARTESIAN_POINT('Origin',(4.425,-4.425,59.4601776313845));
#63378=CARTESIAN_POINT('Origin',(-3.375,-4.44696699141101,59.7821446227955));
#63379=CARTESIAN_POINT('',(4.43786796564403,-4.41213203435596,59.6980455970285));
#63380=CARTESIAN_POINT('',(2.41498854218627,-3.57422794211429,57.6751661735708));
#63381=CARTESIAN_POINT('',(3.95870352594775,-4.89129647405225,60.8548508859502));
#63382=CARTESIAN_POINT('Origin',(-11.4428396698581,-4.425,123.860516270182));
#63383=CARTESIAN_POINT('',(11.9168465442685,3.06684654426849,124.39009016671));
#63384=CARTESIAN_POINT('',(3.,-4.5,129.197093341225));
#63385=CARTESIAN_POINT('Origin',(3.075,-4.425,94.0778586986002));
#63386=CARTESIAN_POINT('',(2.99999999999999,-4.5,128.590508635084));
#63387=CARTESIAN_POINT('Origin',(11.5726967248288,-4.425,125.550115532791));
#63388=CARTESIAN_POINT('',(-4.16279780280838,-13.0127978028084,122.138423626045));
#63389=CARTESIAN_POINT('Origin',(4.425,-4.425,59.4601776313845));
#63390=CARTESIAN_POINT('Origin',(-11.1399331449968,-4.425,122.085809636842));
#63391=CARTESIAN_POINT('',(11.6971631981738,2.84716319817385,122.658958509512));
#63392=CARTESIAN_POINT('',(3.,-4.5,127.312137749071));
#63393=CARTESIAN_POINT('Origin',(3.075,-4.425,93.1353809025232));
#63394=CARTESIAN_POINT('',(3.,-4.5,126.705553042931));
#63395=CARTESIAN_POINT('Origin',(11.2697901999676,-4.425,123.775408899452));
#63396=CARTESIAN_POINT('Origin',(4.425,-4.425,59.4601776313845));
#63397=CARTESIAN_POINT('Ctrl Pts',(-0.935227410421504,-1.48505040008624,
61.4601776313845));
#63398=CARTESIAN_POINT('Ctrl Pts',(-0.935227410421504,-1.48505040008624,
61.3891441263593));
#63399=CARTESIAN_POINT('Ctrl Pts',(-0.919615649085625,-1.49487746321015,
61.2422731598338));
#63400=CARTESIAN_POINT('Ctrl Pts',(-0.849468438578091,-1.53686812251223,
61.0333879936081));
#63401=CARTESIAN_POINT('Ctrl Pts',(-0.735914858055534,-1.59497632661104,
60.8514498111743));
#63402=CARTESIAN_POINT('Ctrl Pts',(-0.598310313784555,-1.65242100436025,
60.7107010115764));
#63403=CARTESIAN_POINT('Ctrl Pts',(-0.448703130287871,-1.69877028516103,
60.6130238318804));
#63404=CARTESIAN_POINT('Ctrl Pts',(-0.33264122576857,-1.72358803958856,
60.564437741829));
#63405=CARTESIAN_POINT('Ctrl Pts',(-0.272364982794092,-1.73372376318135,
60.5450033341972));
#63406=CARTESIAN_POINT('Ctrl Pts',(-0.237531681197459,-1.73876819237024,
60.5354423077009));
#63407=CARTESIAN_POINT('Ctrl Pts',(-0.0789701298399566,-1.75925740461135,
60.4969143456161));
#63408=CARTESIAN_POINT('Ctrl Pts',(0.0760194607809564,-1.75928712608876,
60.4968764455387));
#63409=CARTESIAN_POINT('Ctrl Pts',(0.228735482046854,-1.73994680766547,
60.5332249124204));
#63410=CARTESIAN_POINT('Ctrl Pts',(0.252049875042143,-1.73674755611036,
60.5392730095349));
#63411=CARTESIAN_POINT('Ctrl Pts',(0.292578207370474,-1.73057269707577,
60.5510083786442));
#63412=CARTESIAN_POINT('Ctrl Pts',(0.372075688502887,-1.71598007394311,
60.5791940588586));
#63413=CARTESIAN_POINT('Ctrl Pts',(0.479224028492418,-1.6897225475368,60.6316466004299));
#63414=CARTESIAN_POINT('Ctrl Pts',(0.594393972224216,-1.6522873143202,60.7127508682801));
#63415=CARTESIAN_POINT('Ctrl Pts',(0.722593849137971,-1.60147251676923,
60.834783417798));
#63416=CARTESIAN_POINT('Ctrl Pts',(0.814959219695543,-1.55505030204574,
60.9708247013374));
#63417=CARTESIAN_POINT('Ctrl Pts',(0.871291361756753,-1.52340370940006,
61.10429390882));
#63418=CARTESIAN_POINT('Ctrl Pts',(0.902393644067836,-1.50528176938052,
61.196100120568));
#63419=CARTESIAN_POINT('Ctrl Pts',(0.938735066575289,-1.48284224282614,
61.3654968018582));
#63420=CARTESIAN_POINT('Ctrl Pts',(0.938582534367773,-1.48290872908077,
61.5313282028974));
#63421=CARTESIAN_POINT('Ctrl Pts',(0.904175169636998,-1.50419692024269,
61.7242600329632));
#63422=CARTESIAN_POINT('Ctrl Pts',(0.85721285894179,-1.53213405783326,61.8633698692225));
#63423=CARTESIAN_POINT('Ctrl Pts',(0.775381471169404,-1.57514340099823,
62.0083583724577));
#63424=CARTESIAN_POINT('Ctrl Pts',(0.690738387260799,-1.61425222701105,
62.1162128434089));
#63425=CARTESIAN_POINT('Ctrl Pts',(0.59471425097924,-1.6523256721306,62.2076820178571));
#63426=CARTESIAN_POINT('Ctrl Pts',(0.441520175140093,-1.70219588091644,
62.3156185449291));
#63427=CARTESIAN_POINT('Ctrl Pts',(0.260489914084767,-1.74025400897717,
62.3877929030015));
#63428=CARTESIAN_POINT('Ctrl Pts',(0.0692954676913469,-1.75545738735951,
62.4159688547089));
#63429=CARTESIAN_POINT('Ctrl Pts',(-0.116362742719129,-1.75565543297752,
62.4160667144284));
#63430=CARTESIAN_POINT('Ctrl Pts',(-0.356773244315879,-1.72599810988677,
62.3624101762215));
#63431=CARTESIAN_POINT('Ctrl Pts',(-0.583275116725225,-1.65894838175102,
62.2258716165825));
#63432=CARTESIAN_POINT('Ctrl Pts',(-0.736417081706063,-1.59492671578796,
62.0687636727456));
#63433=CARTESIAN_POINT('Ctrl Pts',(-0.849635873494022,-1.53689456816766,
61.8870852321429));
#63434=CARTESIAN_POINT('Ctrl Pts',(-0.919766275354451,-1.49486469045067,
61.6780476559334));
#63435=CARTESIAN_POINT('Ctrl Pts',(-0.935227410421504,-1.48505040008624,
61.5312111364096));
#63436=CARTESIAN_POINT('Ctrl Pts',(-0.935227410421504,-1.48505040008624,
61.4601776313845));
#63437=CARTESIAN_POINT('Ctrl Pts',(-0.891818273614336,-1.55986263178064,
61.4601776313845));
#63438=CARTESIAN_POINT('Ctrl Pts',(-0.891818273614336,-1.55986263178064,
61.3951284615141));
#63439=CARTESIAN_POINT('Ctrl Pts',(-0.877744688906537,-1.56849750781793,
61.2606215699825));
#63440=CARTESIAN_POINT('Ctrl Pts',(-0.813799731091216,-1.60578900068647,
61.0666402243125));
#63441=CARTESIAN_POINT('Ctrl Pts',(-0.70816041514642,-1.65818502178782,
60.8940616379229));
#63442=CARTESIAN_POINT('Ctrl Pts',(-0.578021741472897,-1.71056879712429,
60.7580300263371));
#63443=CARTESIAN_POINT('Ctrl Pts',(-0.434686640643755,-1.75314130539658,
60.6621866866951));
#63444=CARTESIAN_POINT('Ctrl Pts',(-0.32265618707681,-1.77601059240704,
60.6141022029886));
#63445=CARTESIAN_POINT('Ctrl Pts',(-0.264331980636356,-1.78535838340448,
60.5948182695924));
#63446=CARTESIAN_POINT('Ctrl Pts',(-0.230589683070617,-1.79001281129946,
60.585317478617));
#63447=CARTESIAN_POINT('Ctrl Pts',(-0.0768991900276076,-1.8089236687873,
60.5469930291481));
#63448=CARTESIAN_POINT('Ctrl Pts',(0.0740287221081122,-1.80895102721411,
60.5469534448937));
#63449=CARTESIAN_POINT('Ctrl Pts',(0.222067318628145,-1.79110012631182,
60.5831123928036));
#63450=CARTESIAN_POINT('Ctrl Pts',(0.244658308810622,-1.78814794047804,
60.5891243889555));
#63451=CARTESIAN_POINT('Ctrl Pts',(0.283904295083939,-1.78245099890452,
60.6007819234622));
#63452=CARTESIAN_POINT('Ctrl Pts',(0.360767972306015,-1.76899704119178,
60.6287231584559));
#63453=CARTESIAN_POINT('Ctrl Pts',(0.463978823988154,-1.7448203980967,60.6805097909023));
#63454=CARTESIAN_POINT('Ctrl Pts',(0.574112430572595,-1.71048215605517,
60.7598502334435));
#63455=CARTESIAN_POINT('Ctrl Pts',(0.695680975640035,-1.66408640779924,
60.8780352498123));
#63456=CARTESIAN_POINT('Ctrl Pts',(0.781805858564989,-1.6221390249812,61.0075932553954));
#63457=CARTESIAN_POINT('Ctrl Pts',(0.833613079412961,-1.59385921572437,
61.1323587545323));
#63458=CARTESIAN_POINT('Ctrl Pts',(0.862072495872827,-1.57772634548218,
61.2176672311318));
#63459=CARTESIAN_POINT('Ctrl Pts',(0.895009775933105,-1.55789844255671,
61.373753949522));
#63460=CARTESIAN_POINT('Ctrl Pts',(0.894856619732835,-1.55796819614332,
61.5251376909164));
#63461=CARTESIAN_POINT('Ctrl Pts',(0.863683914665523,-1.57677134969902,
61.7026244669316));
#63462=CARTESIAN_POINT('Ctrl Pts',(0.820835411334987,-1.60159600839885,
61.8318004513303));
#63463=CARTESIAN_POINT('Ctrl Pts',(0.744933623620128,-1.64028625542469,
61.9687681386248));
#63464=CARTESIAN_POINT('Ctrl Pts',(0.665475763530155,-1.67576108720713,
62.0719971623455));
#63465=CARTESIAN_POINT('Ctrl Pts',(0.57442728941605,-1.7105169688379,62.160574523964));
#63466=CARTESIAN_POINT('Ctrl Pts',(0.427934605144566,-1.75626706312665,
62.266178371631));
#63467=CARTESIAN_POINT('Ctrl Pts',(0.25300223677069,-1.79138357718446,62.3378865426985));
#63468=CARTESIAN_POINT('Ctrl Pts',(0.0673494918380112,-1.80542289158326,
62.365969662501));
#63469=CARTESIAN_POINT('Ctrl Pts',(-0.113085827426488,-1.80561147465042,
62.3661013522531));
#63470=CARTESIAN_POINT('Ctrl Pts',(-0.346407983829098,-1.77819658625783,
62.312460591346));
#63471=CARTESIAN_POINT('Ctrl Pts',(-0.563841388541595,-1.7165160210848,
62.1779743621097));
#63472=CARTESIAN_POINT('Ctrl Pts',(-0.708642961553554,-1.6581402336975,
62.0261579496237));
#63473=CARTESIAN_POINT('Ctrl Pts',(-0.813969536493406,-1.60581191306522,
61.8538230221461));
#63474=CARTESIAN_POINT('Ctrl Pts',(-0.877889851198672,-1.56848592986011,
61.6597004901767));
#63475=CARTESIAN_POINT('Ctrl Pts',(-0.891818273614336,-1.55986263178064,
61.5252268012549));
#63476=CARTESIAN_POINT('Ctrl Pts',(-0.891818273614336,-1.55986263178064,
61.4601776313845));
#63477=CARTESIAN_POINT('Ctrl Pts',(-0.848409136807168,-1.63467486347503,
61.4601776313845));
#63478=CARTESIAN_POINT('Ctrl Pts',(-0.848409136807168,-1.63467486347503,
61.4011127966688));
#63479=CARTESIAN_POINT('Ctrl Pts',(-0.835873728727449,-1.6421175524257,
61.2789699801313));
#63480=CARTESIAN_POINT('Ctrl Pts',(-0.778131023604341,-1.67470987886071,
61.0998924550167));
#63481=CARTESIAN_POINT('Ctrl Pts',(-0.680405972237307,-1.72139371696459,
60.9366734646713));
#63482=CARTESIAN_POINT('Ctrl Pts',(-0.55773316916124,-1.76871658988833,
60.8053590410978));
#63483=CARTESIAN_POINT('Ctrl Pts',(-0.420670150999641,-1.80751232563214,
60.7113495415097));
#63484=CARTESIAN_POINT('Ctrl Pts',(-0.312671148385052,-1.82843314522552,
60.6637666641482));
#63485=CARTESIAN_POINT('Ctrl Pts',(-0.256298978478621,-1.83699300362762,
60.6446332049876));
#63486=CARTESIAN_POINT('Ctrl Pts',(-0.223647684943777,-1.84125743022868,
60.635192649533));
#63487=CARTESIAN_POINT('Ctrl Pts',(-0.0748282502152587,-1.85858993296325,
60.5970717126801));
#63488=CARTESIAN_POINT('Ctrl Pts',(0.0720379834352672,-1.85861492833947,
60.5970304442487));
#63489=CARTESIAN_POINT('Ctrl Pts',(0.215399155209435,-1.84225344495817,
60.6329998731868));
#63490=CARTESIAN_POINT('Ctrl Pts',(0.237266742579102,-1.83954832484572,
60.6389757683761));
#63491=CARTESIAN_POINT('Ctrl Pts',(0.275230382797404,-1.83432930073327,
60.6505554682802));
#63492=CARTESIAN_POINT('Ctrl Pts',(0.349460256109143,-1.82201400844044,
60.6782522580532));
#63493=CARTESIAN_POINT('Ctrl Pts',(0.448733619483891,-1.7999182486566,60.7293729813747));
#63494=CARTESIAN_POINT('Ctrl Pts',(0.553830888920974,-1.76867699779014,
60.8069495986068));
#63495=CARTESIAN_POINT('Ctrl Pts',(0.6687681021421,-1.72670029882925,60.9212870818265));
#63496=CARTESIAN_POINT('Ctrl Pts',(0.748652497434435,-1.68922774791666,
61.0443618094534));
#63497=CARTESIAN_POINT('Ctrl Pts',(0.795934797069171,-1.66431472204868,
61.1604236002446));
#63498=CARTESIAN_POINT('Ctrl Pts',(0.821751347677819,-1.65017092158383,
61.2392343416956));
#63499=CARTESIAN_POINT('Ctrl Pts',(0.851284485290922,-1.63295464228727,
61.3820110971857));
#63500=CARTESIAN_POINT('Ctrl Pts',(0.851130705097898,-1.63302766320586,
61.5189471789355));
#63501=CARTESIAN_POINT('Ctrl Pts',(0.823192659694048,-1.64934577915535,
61.6809889009));
#63502=CARTESIAN_POINT('Ctrl Pts',(0.784457963728185,-1.67105795896445,
61.8002310334381));
#63503=CARTESIAN_POINT('Ctrl Pts',(0.714485776070854,-1.70542910985115,
61.9291779047919));
#63504=CARTESIAN_POINT('Ctrl Pts',(0.640213139799511,-1.73726994740321,
62.0277814812822));
#63505=CARTESIAN_POINT('Ctrl Pts',(0.554140327852861,-1.76870826554519,
62.113467030071));
#63506=CARTESIAN_POINT('Ctrl Pts',(0.414349035149039,-1.81033824533686,
62.216738198333));
#63507=CARTESIAN_POINT('Ctrl Pts',(0.245514559456612,-1.84251314539175,
62.2879801823955));
#63508=CARTESIAN_POINT('Ctrl Pts',(0.0654035159846756,-1.855388395807,62.3159704702932));
#63509=CARTESIAN_POINT('Ctrl Pts',(-0.109808912133848,-1.85556751632333,
62.3161359900777));
#63510=CARTESIAN_POINT('Ctrl Pts',(-0.336042723342318,-1.8303950626289,
62.2625110064705));
#63511=CARTESIAN_POINT('Ctrl Pts',(-0.544407660357965,-1.77408366041858,
62.130077107637));
#63512=CARTESIAN_POINT('Ctrl Pts',(-0.680868841401045,-1.72135375160704,
61.9835522265018));
#63513=CARTESIAN_POINT('Ctrl Pts',(-0.778303199492791,-1.67472925796279,
61.8205608121493));
#63514=CARTESIAN_POINT('Ctrl Pts',(-0.836013427042894,-1.64210716926955,
61.6413533244201));
#63515=CARTESIAN_POINT('Ctrl Pts',(-0.848409136807168,-1.63467486347503,
61.5192424661002));
#63516=CARTESIAN_POINT('Ctrl Pts',(-0.848409136807168,-1.63467486347503,
61.4601776313845));
#63517=CARTESIAN_POINT('Ctrl Pts',(-0.805,-1.70948709516943,61.4601776313845));
#63518=CARTESIAN_POINT('Ctrl Pts',(-0.805,-1.70948709516943,61.4070971318236));
#63519=CARTESIAN_POINT('Ctrl Pts',(-0.794002768548361,-1.71573759703348,
61.29731839028));
#63520=CARTESIAN_POINT('Ctrl Pts',(-0.742462316117465,-1.74363075703495,
61.133144685721));
#63521=CARTESIAN_POINT('Ctrl Pts',(-0.652651529328193,-1.78460241214137,
60.9792852914198));
#63522=CARTESIAN_POINT('Ctrl Pts',(-0.537444596849582,-1.82686438265237,
60.8526880558586));
#63523=CARTESIAN_POINT('Ctrl Pts',(-0.406653661355526,-1.8618833458677,
60.7605123963243));
#63524=CARTESIAN_POINT('Ctrl Pts',(-0.302686109693293,-1.880855698044,60.7134311253077));
#63525=CARTESIAN_POINT('Ctrl Pts',(-0.248265976320886,-1.88862762385075,
60.6944481403828));
#63526=CARTESIAN_POINT('Ctrl Pts',(-0.216705686816935,-1.8925020491579,
60.685067820449));
#63527=CARTESIAN_POINT('Ctrl Pts',(-0.0727573104029104,-1.9082561971392,
60.6471503962121));
#63528=CARTESIAN_POINT('Ctrl Pts',(0.0700472447624226,-1.90827882946482,
60.6471074436038));
#63529=CARTESIAN_POINT('Ctrl Pts',(0.208730991790726,-1.89340676360453,
60.68288735357));
#63530=CARTESIAN_POINT('Ctrl Pts',(0.229875176347581,-1.8909487092134,60.6888271477967));
#63531=CARTESIAN_POINT('Ctrl Pts',(0.266556470510869,-1.88620760256202,
60.7003290130983));
#63532=CARTESIAN_POINT('Ctrl Pts',(0.33815253991227,-1.8750309756891,60.7277813576505));
#63533=CARTESIAN_POINT('Ctrl Pts',(0.433488414979626,-1.8550160992165,60.7782361718472));
#63534=CARTESIAN_POINT('Ctrl Pts',(0.533549347269353,-1.82687183952511,
60.8540489637702));
#63535=CARTESIAN_POINT('Ctrl Pts',(0.641855228644165,-1.78931418985927,
60.9645389138408));
#63536=CARTESIAN_POINT('Ctrl Pts',(0.715499136303881,-1.75631647085212,
61.0811303635114));
#63537=CARTESIAN_POINT('Ctrl Pts',(0.75825651472538,-1.73477022837298,61.1884884459569));
#63538=CARTESIAN_POINT('Ctrl Pts',(0.781430199482811,-1.72261549768548,
61.2608014522594));
#63539=CARTESIAN_POINT('Ctrl Pts',(0.807559194648739,-1.70801084201783,
61.3902682448495));
#63540=CARTESIAN_POINT('Ctrl Pts',(0.80740479046296,-1.70808713026841,61.5127566669546));
#63541=CARTESIAN_POINT('Ctrl Pts',(0.782701404722573,-1.72192020861167,
61.6593533348685));
#63542=CARTESIAN_POINT('Ctrl Pts',(0.748080516121382,-1.74051990953005,
61.7686616155459));
#63543=CARTESIAN_POINT('Ctrl Pts',(0.684037928521579,-1.7705719642776,61.889587670959));
#63544=CARTESIAN_POINT('Ctrl Pts',(0.614950516068867,-1.79877880759929,
61.9835658002188));
#63545=CARTESIAN_POINT('Ctrl Pts',(0.533853366289671,-1.82689956225249,
62.0663595361779));
#63546=CARTESIAN_POINT('Ctrl Pts',(0.400763465153512,-1.86440942754707,
62.1672980250349));
#63547=CARTESIAN_POINT('Ctrl Pts',(0.238026882142535,-1.89364271359903,
62.2380738220926));
#63548=CARTESIAN_POINT('Ctrl Pts',(0.0634575401313399,-1.90535390003075,
62.2659712780854));
#63549=CARTESIAN_POINT('Ctrl Pts',(-0.106531996841207,-1.90552355799623,
62.2661706279024));
#63550=CARTESIAN_POINT('Ctrl Pts',(-0.325677462855537,-1.88259353899996,
62.2125614215949));
#63551=CARTESIAN_POINT('Ctrl Pts',(-0.524973932174335,-1.83165129975237,
62.0821798531642));
#63552=CARTESIAN_POINT('Ctrl Pts',(-0.653094721248536,-1.78456726951658,
61.9409465033799));
#63553=CARTESIAN_POINT('Ctrl Pts',(-0.742636862492175,-1.74364660286035,
61.7872986021525));
#63554=CARTESIAN_POINT('Ctrl Pts',(-0.794137002887115,-1.71572840867899,
61.6230061586634));
#63555=CARTESIAN_POINT('Ctrl Pts',(-0.805,-1.70948709516943,61.5132581309454));
#63556=CARTESIAN_POINT('Ctrl Pts',(-0.805,-1.70948709516943,61.4601776313845));
#63557=CARTESIAN_POINT('',(-0.935227410421504,-1.48505040008624,61.4601776313845));
#63558=CARTESIAN_POINT('',(-0.805,-1.70948709516943,61.4601776313845));
#63559=CARTESIAN_POINT('',(-0.935227410421504,-1.48505040008624,61.4601776313845));
#63560=CARTESIAN_POINT('',(-3.66463531352099E-6,-1.90497281869116,60.6550571401644));
#63561=CARTESIAN_POINT('Ctrl Pts',(-0.805,-1.70948709516943,61.4601776313845));
#63562=CARTESIAN_POINT('Ctrl Pts',(-0.805,-1.70948709516943,61.4070971318236));
#63563=CARTESIAN_POINT('Ctrl Pts',(-0.794002768548361,-1.71573759703348,
61.29731839028));
#63564=CARTESIAN_POINT('Ctrl Pts',(-0.742462316117465,-1.74363075703495,
61.133144685721));
#63565=CARTESIAN_POINT('Ctrl Pts',(-0.652651529328193,-1.78460241214137,
60.9792852914198));
#63566=CARTESIAN_POINT('Ctrl Pts',(-0.537444596849582,-1.82686438265237,
60.8526880558586));
#63567=CARTESIAN_POINT('Ctrl Pts',(-0.406653661355526,-1.8618833458677,
60.7605123963243));
#63568=CARTESIAN_POINT('Ctrl Pts',(-0.302686109693293,-1.880855698044,60.7134311253077));
#63569=CARTESIAN_POINT('Ctrl Pts',(-0.248265976320886,-1.88862762385075,
60.6944481403828));
#63570=CARTESIAN_POINT('Ctrl Pts',(-0.216705686816935,-1.8925020491579,
60.685067820449));
#63571=CARTESIAN_POINT('Ctrl Pts',(-0.136734366586922,-1.90125435359195,
60.6640025847618));
#63572=CARTESIAN_POINT('Ctrl Pts',(-0.0643497242950811,-1.90496731588625,
60.6550692535498));
#63573=CARTESIAN_POINT('Ctrl Pts',(-3.66463531351058E-6,-1.90497281869116,
60.6550571401644));
#63574=CARTESIAN_POINT('Ctrl Pts',(-3.66463531351058E-6,-1.90497281869116,
60.6550571401644));
#63575=CARTESIAN_POINT('Ctrl Pts',(0.0643423950244553,-1.90497832149607,
60.655045026779));
#63576=CARTESIAN_POINT('Ctrl Pts',(0.134055128006254,-1.90141479906776,
60.6636212482036));
#63577=CARTESIAN_POINT('Ctrl Pts',(0.208730991790726,-1.89340676360453,
60.68288735357));
#63578=CARTESIAN_POINT('Ctrl Pts',(0.229875176347581,-1.8909487092134,60.6888271477967));
#63579=CARTESIAN_POINT('Ctrl Pts',(0.266556470510869,-1.88620760256202,
60.7003290130983));
#63580=CARTESIAN_POINT('Ctrl Pts',(0.33815253991227,-1.8750309756891,60.7277813576505));
#63581=CARTESIAN_POINT('Ctrl Pts',(0.433488414979626,-1.8550160992165,60.7782361718472));
#63582=CARTESIAN_POINT('Ctrl Pts',(0.533549347269353,-1.82687183952511,
60.8540489637702));
#63583=CARTESIAN_POINT('Ctrl Pts',(0.641855228644165,-1.78931418985927,
60.9645389138408));
#63584=CARTESIAN_POINT('Ctrl Pts',(0.715499136303881,-1.75631647085212,
61.0811303635114));
#63585=CARTESIAN_POINT('Ctrl Pts',(0.75825651472538,-1.73477022837298,61.1884884459569));
#63586=CARTESIAN_POINT('Ctrl Pts',(0.781430199482811,-1.72261549768548,
61.2608014522594));
#63587=CARTESIAN_POINT('Ctrl Pts',(0.807559194648739,-1.70801084201783,
61.3902682448495));
#63588=CARTESIAN_POINT('Ctrl Pts',(0.80740479046296,-1.70808713026841,61.5127566669546));
#63589=CARTESIAN_POINT('Ctrl Pts',(0.782701404722573,-1.72192020861167,
61.6593533348685));
#63590=CARTESIAN_POINT('Ctrl Pts',(0.748080516121382,-1.74051990953005,
61.7686616155459));
#63591=CARTESIAN_POINT('Ctrl Pts',(0.684037928521579,-1.7705719642776,61.889587670959));
#63592=CARTESIAN_POINT('Ctrl Pts',(0.614950516068867,-1.79877880759929,
61.9835658002188));
#63593=CARTESIAN_POINT('Ctrl Pts',(0.533853366289671,-1.82689956225249,
62.0663595361779));
#63594=CARTESIAN_POINT('Ctrl Pts',(0.400763465153512,-1.86440942754707,
62.1672980250349));
#63595=CARTESIAN_POINT('Ctrl Pts',(0.238026882142535,-1.89364271359903,
62.2380738220926));
#63596=CARTESIAN_POINT('Ctrl Pts',(0.0634575401313399,-1.90535390003075,
62.2659712780854));
#63597=CARTESIAN_POINT('Ctrl Pts',(-0.106531996841207,-1.90552355799623,
62.2661706279024));
#63598=CARTESIAN_POINT('Ctrl Pts',(-0.325677462855537,-1.88259353899996,
62.2125614215949));
#63599=CARTESIAN_POINT('Ctrl Pts',(-0.524973932174335,-1.83165129975237,
62.0821798531642));
#63600=CARTESIAN_POINT('Ctrl Pts',(-0.653094721248536,-1.78456726951658,
61.9409465033799));
#63601=CARTESIAN_POINT('Ctrl Pts',(-0.742636862492175,-1.74364660286035,
61.7872986021525));
#63602=CARTESIAN_POINT('Ctrl Pts',(-0.794137002887115,-1.71572840867899,
61.6230061586634));
#63603=CARTESIAN_POINT('Ctrl Pts',(-0.805,-1.70948709516943,61.5132581309454));
#63604=CARTESIAN_POINT('Ctrl Pts',(-0.805,-1.70948709516943,61.4601776313845));
#63605=CARTESIAN_POINT('Ctrl Pts',(-0.935227410421504,-1.48505040008624,
61.4601776313845));
#63606=CARTESIAN_POINT('Ctrl Pts',(-0.935227410421504,-1.48505040008624,
61.5312111364096));
#63607=CARTESIAN_POINT('Ctrl Pts',(-0.919766275354451,-1.49486469045067,
61.6780476559334));
#63608=CARTESIAN_POINT('Ctrl Pts',(-0.849635873494022,-1.53689456816766,
61.8870852321429));
#63609=CARTESIAN_POINT('Ctrl Pts',(-0.736417081706063,-1.59492671578796,
62.0687636727456));
#63610=CARTESIAN_POINT('Ctrl Pts',(-0.583275116725225,-1.65894838175102,
62.2258716165825));
#63611=CARTESIAN_POINT('Ctrl Pts',(-0.356773244315879,-1.72599810988677,
62.3624101762215));
#63612=CARTESIAN_POINT('Ctrl Pts',(-0.116362742719129,-1.75565543297752,
62.4160667144284));
#63613=CARTESIAN_POINT('Ctrl Pts',(0.0692954676913469,-1.75545738735951,
62.4159688547089));
#63614=CARTESIAN_POINT('Ctrl Pts',(0.260489914084767,-1.74025400897717,
62.3877929030015));
#63615=CARTESIAN_POINT('Ctrl Pts',(0.441520175140093,-1.70219588091644,
62.3156185449291));
#63616=CARTESIAN_POINT('Ctrl Pts',(0.59471425097924,-1.6523256721306,62.2076820178571));
#63617=CARTESIAN_POINT('Ctrl Pts',(0.690738387260799,-1.61425222701105,
62.1162128434089));
#63618=CARTESIAN_POINT('Ctrl Pts',(0.775381471169404,-1.57514340099823,
62.0083583724577));
#63619=CARTESIAN_POINT('Ctrl Pts',(0.85721285894179,-1.53213405783326,61.8633698692225));
#63620=CARTESIAN_POINT('Ctrl Pts',(0.904175169636998,-1.50419692024269,
61.7242600329632));
#63621=CARTESIAN_POINT('Ctrl Pts',(0.938582534367773,-1.48290872908077,
61.5313282028974));
#63622=CARTESIAN_POINT('Ctrl Pts',(0.938735066575289,-1.48284224282614,
61.3654968018582));
#63623=CARTESIAN_POINT('Ctrl Pts',(0.902393644067836,-1.50528176938052,
61.196100120568));
#63624=CARTESIAN_POINT('Ctrl Pts',(0.871291361756753,-1.52340370940006,
61.10429390882));
#63625=CARTESIAN_POINT('Ctrl Pts',(0.814959219695543,-1.55505030204574,
60.9708247013374));
#63626=CARTESIAN_POINT('Ctrl Pts',(0.722593849137971,-1.60147251676923,
60.834783417798));
#63627=CARTESIAN_POINT('Ctrl Pts',(0.594393972224216,-1.6522873143202,60.7127508682801));
#63628=CARTESIAN_POINT('Ctrl Pts',(0.479224028492418,-1.6897225475368,60.6316466004299));
#63629=CARTESIAN_POINT('Ctrl Pts',(0.372075688502887,-1.71598007394311,
60.5791940588586));
#63630=CARTESIAN_POINT('Ctrl Pts',(0.292578207370474,-1.73057269707577,
60.5510083786442));
#63631=CARTESIAN_POINT('Ctrl Pts',(0.252049875042143,-1.73674755611036,
60.5392730095349));
#63632=CARTESIAN_POINT('Ctrl Pts',(0.228735482046854,-1.73994680766547,
60.5332249124204));
#63633=CARTESIAN_POINT('Ctrl Pts',(0.0760194607809564,-1.75928712608876,
60.4968764455387));
#63634=CARTESIAN_POINT('Ctrl Pts',(-0.0789701298399566,-1.75925740461135,
60.4969143456161));
#63635=CARTESIAN_POINT('Ctrl Pts',(-0.237531681197459,-1.73876819237024,
60.5354423077009));
#63636=CARTESIAN_POINT('Ctrl Pts',(-0.272364982794092,-1.73372376318135,
60.5450033341972));
#63637=CARTESIAN_POINT('Ctrl Pts',(-0.33264122576857,-1.72358803958856,
60.564437741829));
#63638=CARTESIAN_POINT('Ctrl Pts',(-0.448703130287871,-1.69877028516103,
60.6130238318804));
#63639=CARTESIAN_POINT('Ctrl Pts',(-0.598310313784555,-1.65242100436025,
60.7107010115764));
#63640=CARTESIAN_POINT('Ctrl Pts',(-0.735914858055534,-1.59497632661104,
60.8514498111743));
#63641=CARTESIAN_POINT('Ctrl Pts',(-0.849468438578091,-1.53686812251223,
61.0333879936081));
#63642=CARTESIAN_POINT('Ctrl Pts',(-0.919615649085625,-1.49487746321015,
61.2422731598338));
#63643=CARTESIAN_POINT('Ctrl Pts',(-0.935227410421504,-1.48505040008624,
61.3891441263593));
#63644=CARTESIAN_POINT('Ctrl Pts',(-0.935227410421504,-1.48505040008624,
61.4601776313845));
#63645=CARTESIAN_POINT('Origin',(0.,-2.865,61.4601776313845));
#63646=CARTESIAN_POINT('',(-9.85840673313619E-17,-4.4,60.6551776313845));
#63647=CARTESIAN_POINT('Origin',(0.,-4.4,61.4601776313845));
#63648=CARTESIAN_POINT('',(-9.85840673313619E-17,-2.865,60.6551776313845));
#63649=CARTESIAN_POINT('Origin',(0.,0.,64.4451776313845));
#63650=CARTESIAN_POINT('',(-1.755,-2.1492551325036E-16,59.6101776313845));
#63651=CARTESIAN_POINT('Origin',(0.,0.,59.6101776313845));
#63652=CARTESIAN_POINT('',(-1.755,-2.1492551325036E-16,69.4601776313845));
#63653=CARTESIAN_POINT('',(-1.755,-2.1492551325036E-16,64.4451776313845));
#63654=CARTESIAN_POINT('Origin',(0.,0.,69.4601776313845));
#63655=CARTESIAN_POINT('Origin',(0.,-4.45,61.4601776313845));
#63656=CARTESIAN_POINT('',(1.04707301327099E-16,-4.45,60.6051776313845));
#63657=CARTESIAN_POINT('Origin',(0.,0.,59.5351776313845));
#63658=CARTESIAN_POINT('',(-1.83,2.24110364243966E-16,59.5351776313845));
#63659=CARTESIAN_POINT('Origin',(0.,0.,69.4601776313845));
#63660=CARTESIAN_POINT('',(0.,0.,70.5146880177779));
#63661=CARTESIAN_POINT('',(-1.755,-2.1492551325036E-16,69.4601776313845));
#63662=CARTESIAN_POINT('Origin',(4.425,4.425,59.4601776313845));
#63663=CARTESIAN_POINT('',(4.5,4.35,59.7601776313845));
#63664=CARTESIAN_POINT('',(4.5,4.35,59.4601776313845));
#63665=CARTESIAN_POINT('',(5.47500000000001,3.37499999999999,60.7351776313845));
#63666=CARTESIAN_POINT('Origin',(4.425,4.425,59.4601776313845));
#63667=CARTESIAN_POINT('',(4.5,4.35,59.4601776313845));
#63668=CARTESIAN_POINT('Origin',(4.5,-4.5,59.4601776313845));
#63669=CARTESIAN_POINT('',(4.5,-4.35,59.7601776313845));
#63670=CARTESIAN_POINT('',(4.5,-4.35,59.4601776313845));
#63671=CARTESIAN_POINT('',(4.5,-2.25,59.7601776313845));
#63672=CARTESIAN_POINT('Origin',(4.5,-4.5,59.4601776313845));
#63673=CARTESIAN_POINT('Origin',(4.5,-4.5,59.4601776313845));
#63674=CARTESIAN_POINT('Origin',(4.5,-4.5,59.4601776313845));
#63675=CARTESIAN_POINT('Origin',(4.5,-4.5,59.4601776313845));
#63676=CARTESIAN_POINT('Origin',(4.5,-4.5,59.4601776313845));
#63677=CARTESIAN_POINT('Origin',(4.5,-4.5,59.4601776313845));
#63678=CARTESIAN_POINT('Origin',(4.425,-4.425,59.4601776313845));
#63679=CARTESIAN_POINT('',(4.725,-4.125,59.9851776313845));
#63680=CARTESIAN_POINT('Origin',(4.425,-4.425,59.4601776313845));
#63681=CARTESIAN_POINT('Origin',(4.425,-4.425,59.4601776313845));
#63682=CARTESIAN_POINT('Origin',(4.425,-4.425,59.4601776313845));
#63683=CARTESIAN_POINT('Origin',(2.25,4.35,144.810177631385));
#63684=CARTESIAN_POINT('',(4.2,4.2,144.960177631385));
#63685=CARTESIAN_POINT('',(2.25,4.2,144.960177631385));
#63686=CARTESIAN_POINT('',(4.2,4.2,144.960177631385));
#63687=CARTESIAN_POINT('Origin',(4.35,-2.25,59.6101776313845));
#63688=CARTESIAN_POINT('',(4.2,4.2,59.4601776313845));
#63689=CARTESIAN_POINT('Origin',(4.35,-2.25,144.810177631385));
#63690=CARTESIAN_POINT('',(4.2,-2.25,144.960177631385));
#63691=CARTESIAN_POINT('Origin',(2.25,4.35,59.6101776313845));
#63692=CARTESIAN_POINT('Origin',(0.,0.,144.960177631385));
#63693=CARTESIAN_POINT('Origin',(-4.5,4.5,59.4601776313845));
#70736=UNCERTAINTY_MEASURE_WITH_UNIT(LENGTH_MEASURE(0.001),#70758,
'DISTANCE_ACCURACY_VALUE',
'Maximum model space distance between geometric entities at asserted c
onnectivities');
#70740=UNCERTAINTY_MEASURE_WITH_UNIT(LENGTH_MEASURE(0.001),#70758,
'DISTANCE_ACCURACY_VALUE',
'Maximum model space distance between geometric entities at asserted c
onnectivities');
#70753=(
GEOMETRIC_REPRESENTATION_CONTEXT(3)
GLOBAL_UNCERTAINTY_ASSIGNED_CONTEXT((#70736))
GLOBAL_UNIT_ASSIGNED_CONTEXT((#70758,#70760,#70761))
REPRESENTATION_CONTEXT('','3D')
);
#70757=(
GEOMETRIC_REPRESENTATION_CONTEXT(3)
GLOBAL_UNCERTAINTY_ASSIGNED_CONTEXT((#70740))
GLOBAL_UNIT_ASSIGNED_CONTEXT((#70758,#70760,#70761))
REPRESENTATION_CONTEXT('','3D')
);
#70758=(
LENGTH_UNIT()
NAMED_UNIT(*)
SI_UNIT(.CENTI.,.METRE.)
);
#70760=(
NAMED_UNIT(*)
PLANE_ANGLE_UNIT()
SI_UNIT($,.RADIAN.)
);
#70761=(
NAMED_UNIT(*)
SI_UNIT($,.STERADIAN.)
SOLID_ANGLE_UNIT()
);
#70774=SHAPE_DEFINITION_REPRESENTATION(#70790,#70829);
#70790=PRODUCT_DEFINITION_SHAPE('',$,#70846);
#70829=SHAPE_REPRESENTATION('',(#27818),#70753);
#70833=PRODUCT_DEFINITION_CONTEXT('part definition',#70883,'design');
#70846=PRODUCT_DEFINITION('2026-10-19-02-58-48-360',
'02_Rack_Ram_90x90x855_m6_Rack',#70862,#70833);
#70862=PRODUCT_DEFINITION_FORMATION('',$,#70897);
#70883=APPLICATION_CONTEXT(
'Core Data for Automotive Mechanical Design Process');
#70884=PRODUCT_CONTEXT('part definition',#70883,'mechanical');
#70897=PRODUCT('2026-10-19-02-58-48-360',
'02_Rack_Ram_90x90x855_m6_Rack',$,(#70884));
#71027=COLOUR_RGB('Light Blue',0.38,0.62,0.78);
#71028=FILL_AREA_STYLE_COLOUR('',#71027);
#71029=FILL_AREA_STYLE('',(#71028));
#71030=SURFACE_STYLE_FILL_AREA(#71029);
#71031=SURFACE_SIDE_STYLE('',(#71030));
#71032=SURFACE_STYLE_USAGE(.BOTH.,#71031);
#71033=PRESENTATION_STYLE_ASSIGNMENT((#71032));
ENDSEC;
END-ISO-10303-21;
